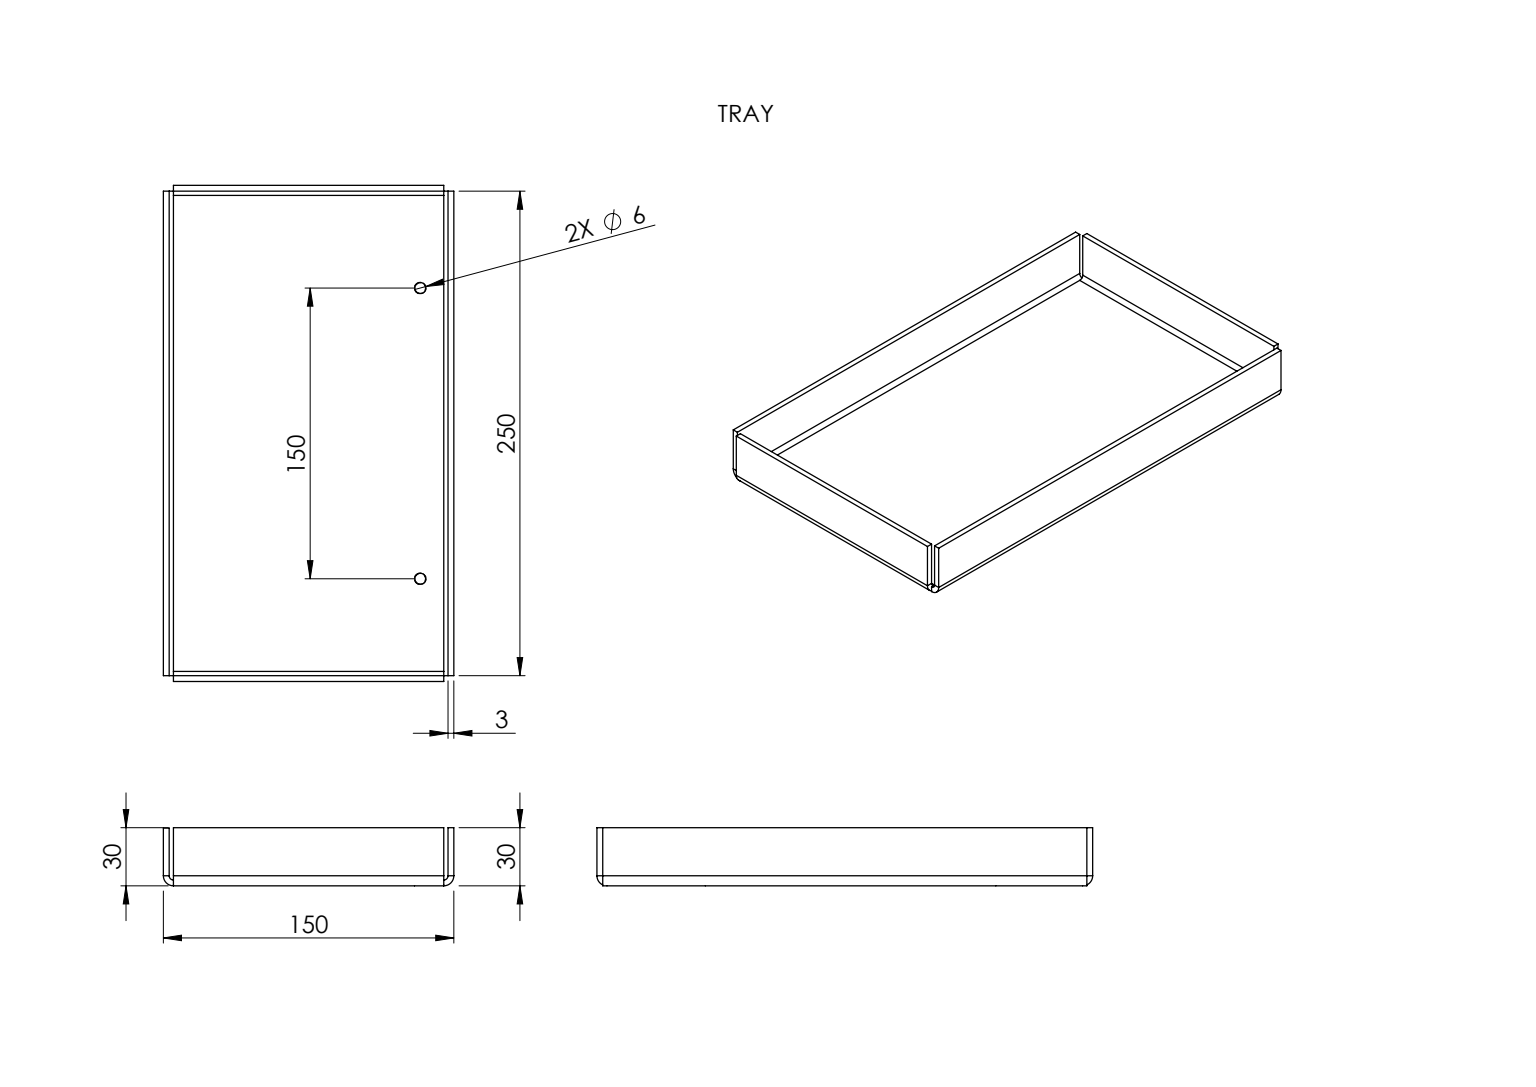
ISO-10303-21;
HEADER;
FILE_DESCRIPTION (('STEP AP214'),
    '1' );
FILE_NAME ('tray.step',
    '2026-10-25T17:17:34',
    ( '' ),
    ( '' ),
    'SwSTEP 2.0',
    'SolidWorks 2026',
    '' );
FILE_SCHEMA (( 'AUTOMOTIVE_DESIGN' ));
ENDSEC;

DATA;
#6=CARTESIAN_POINT ( 'NONE',  ( 231.0999999999999375, -32.62499999999999289, 102.5980762113533018 ) ) ;
#10=CARTESIAN_POINT ( 'NONE',  ( 232.5999999999999375, -34.55624999877095860, 96.53589838486223584 ) ) ;
#11=CARTESIAN_POINT ( 'NONE',  ( 234.0999999999999375, -32.34374999877096002, -52.59807621135342970 ) ) ;
#18=ORIENTED_EDGE ( 'NONE', *, *, #10099, .F. ) ;
#24=CARTESIAN_POINT ( 'NONE',  ( 231.7961524227065979, -33.50759618943233420, 103.0000000000000000 ) ) ;
#28=CARTESIAN_POINT ( 'NONE',  ( 233.9782151781249411, -31.19062499938547717, 97.61286128772489690 ) ) ;
#32=CARTESIAN_POINT ( 'NONE',  ( 233.4038475772933339, -34.57634618820330275, -53.00000000000011369 ) ) ;
#36=CARTESIAN_POINT ( 'NONE',  ( 233.9782151781249411, -32.54062499938547859, -52.38713871227520968 ) ) ;
#44=CARTESIAN_POINT ( 'NONE',  ( 235.3564303562499447, -33.92812499938548143, 98.40857419181659793 ) ) ;
#45=CARTESIAN_POINT ( 'NONE',  ( 232.5999999999999943, -33.40312499938547575, -53.18285161636690361 ) ) ;
#47=EDGE_CURVE ( 'NONE', #12317, #11119, #12856, .T. ) ;
#49=ORIENTED_EDGE ( 'NONE', *, *, #18550, .F. ) ;
#51=CARTESIAN_POINT ( 'NONE',  ( 235.3564303562499447, -34.41562499938547859, -50.00000000000011369 ) ) ;
#52=CARTESIAN_POINT ( 'NONE',  ( 232.5999999999999375, -33.20624999877097139, 97.00000000000000000 ) ) ;
#56=CARTESIAN_POINT ( 'NONE',  ( 233.9782151781249411, -31.90312499938548285, -47.61286128772501769 ) ) ;
#71=B_SPLINE_CURVE_WITH_KNOTS ( 'NONE', 3,
 ( #6677, #3729, #9694, #17123, #815, #2842, #14458, #7240, #5600, #9889, #2460, #18880, #18782, #15852, #1291, #17315, #16038, #17507 ),
 .UNSPECIFIED., .F., .F.,
 ( 4, 2, 2, 2, 2, 2, 2, 2, 4 ),
 ( 0.000000000000000000, 0.0007106627595359568412, 0.001421325519071913682, 0.002131988278607870740, 0.002842651038143827365, 0.003553313797679783989, 0.004263976557215741481, 0.004974639316751698105, 0.005685302076287654729 ),
 .UNSPECIFIED. ) ;
#78=PLANE ( 'NONE',  #7094 ) ;
#88=CARTESIAN_POINT ( 'NONE',  ( 105.2000000000000455, -29.80000000000002203, 147.7999999999999829 ) ) ;
#92=CARTESIAN_POINT ( 'NONE',  ( 229.8435696437499303, -31.60312499938548214, 99.99999999999998579 ) ) ;
#96=CARTESIAN_POINT ( 'NONE',  ( 233.4038475772933339, -33.67634618820329706, 96.99999999999998579 ) ) ;
#100=CARTESIAN_POINT ( 'NONE',  ( 232.5999999999999375, -33.43124999877096570, 102.9999999999999858 ) ) ;
#101=EDGE_CURVE ( 'NONE', #1894, #1510, #1410, .T. ) ;
#103=CARTESIAN_POINT ( 'NONE',  ( 232.5999999999999375, -34.61249999999999716, 96.53589838486223584 ) ) ;
#105=CARTESIAN_POINT ( 'NONE',  ( 231.2217848218749339, -34.22812499938548569, -47.61286128772501769 ) ) ;
#107=CARTESIAN_POINT ( 'NONE',  ( 233.9782151781249411, -30.55312499938548143, 102.3871387122750889 ) ) ;
#108=CARTESIAN_POINT ( 'NONE',  ( 229.5999999999999375, -33.99374999877096570, -50.00000000000011369 ) ) ;
#111=EDGE_CURVE ( 'NONE', #18607, #16633, #16646, .T. ) ;
#117=ORIENTED_EDGE ( 'NONE', *, *, #1142, .T. ) ;
#119=CARTESIAN_POINT ( 'NONE',  ( 232.5999999999999375, -32.36249999999999716, 97.00000000000000000 ) ) ;
#123=FACE_OUTER_BOUND ( 'NONE', #5516, .T. ) ;
#125=CARTESIAN_POINT ( 'NONE',  ( 234.0999999999999375, -33.29999999999999716, 97.40192378864668399 ) ) ;
#128=CARTESIAN_POINT ( 'NONE',  ( 229.8435696437499303, -31.04062499938547859, 99.99999999999998579 ) ) ;
#130=SHAPE_REPRESENTATION_RELATIONSHIP ( 'NONE' , 'NONE' ,  #4499, #5537 ) ;
#133=CARTESIAN_POINT ( 'NONE',  ( 233.4038475772933054, -34.76115380933863008, -47.00000000000011369 ) ) ;
#136=FACE_OUTER_BOUND ( 'NONE', #875, .T. ) ;
#137=CARTESIAN_POINT ( 'NONE',  ( 233.9782151781249411, -32.24062499938548143, -47.61286128772501769 ) ) ;
#138=VERTEX_POINT ( 'NONE', #3624 ) ;
#144=CARTESIAN_POINT ( 'NONE',  ( 244.7999999999999545, -32.00000000000000000, -100.0000000000000000 ) ) ;
#145=CARTESIAN_POINT ( 'NONE',  ( 231.2217848218749339, -34.71562499938547575, 97.61286128772489690 ) ) ;
#150=CARTESIAN_POINT ( 'NONE',  ( 235.5999999999999375, -32.47499999999999432, -50.00000000000011369 ) ) ;
#155=CARTESIAN_POINT ( 'NONE',  ( 229.8435696437499871, -31.11562499938547788, -48.40857419181671162 ) ) ;
#159=CARTESIAN_POINT ( 'NONE',  ( 233.9782151781249411, -34.94062499938547717, 102.3871387122750889 ) ) ;
#162=EDGE_CURVE ( 'NONE', #9344, #9023, #15270, .T. ) ;
#165=CARTESIAN_POINT ( 'NONE',  ( 230.0248882325332147, -35.00000000000000711, 98.48300226792288470 ) ) ;
#175=EDGE_CURVE ( 'NONE', #12231, #5767, #14452, .T. ) ;
#186=CARTESIAN_POINT ( 'NONE',  ( 232.5999999999999375, -34.61249999999999716, -53.00000000000011369 ) ) ;
#188=CARTESIAN_POINT ( 'NONE',  ( 233.9782151781249411, -32.35312499938547859, 102.3871387122750889 ) ) ;
#197=CARTESIAN_POINT ( 'NONE',  ( 235.5999999999999943, -34.76249999999999574, 101.7320508075688537 ) ) ;
#199=CARTESIAN_POINT ( 'NONE',  ( 231.2217848218749339, -34.37812499938547717, -52.38713871227520968 ) ) ;
#201=CARTESIAN_POINT ( 'NONE',  ( 229.8435696437499871, -30.66562499938547859, 101.5914258081833879 ) ) ;
#202=CARTESIAN_POINT ( 'NONE',  ( 229.5999999999999375, -33.95624999877095718, -48.26794919243123161 ) ) ;
#205=ORIENTED_EDGE ( 'NONE', *, *, #14467, .T. ) ;
#207=CARTESIAN_POINT ( 'NONE',  ( 105.1999999999999886, -29.80000000000002203, -100.0000000000000142 ) ) ;
#214=CARTESIAN_POINT ( 'NONE',  ( 229.5999999999999375, -33.60000000000000142, 99.99999999999998579 ) ) ;
#221=CARTESIAN_POINT ( 'NONE',  ( 235.3564303562499447, -32.16562499938547859, 99.99999999999998579 ) ) ;
#226=CARTESIAN_POINT ( 'NONE',  ( 235.5999999999999375, -33.82499999999999574, 99.99999999999998579 ) ) ;
#227=LINE ( 'NONE', #4417, #3668 ) ;
#228=CARTESIAN_POINT ( 'NONE',  ( 230.7429016803109221, -35.00000000000000711, -47.88253972981398476 ) ) ;
#229=LINE ( 'NONE', #334, #1662 ) ;
#238=CARTESIAN_POINT ( 'NONE',  ( 229.8435696437499303, -33.29062499938547148, 99.99999999999998579 ) ) ;
#239=CARTESIAN_POINT ( 'NONE',  ( 231.7960411235079050, -35.00000000000002132, -47.36341917746382535 ) ) ;
#240=VECTOR ( 'NONE', #19274, 1000.000000000000000 ) ;
#243=ORIENTED_EDGE ( 'NONE', *, *, #11982, .F. ) ;
#244=CARTESIAN_POINT ( 'NONE',  ( 229.5999999999999375, -32.21249999999999858, -48.26794919243123161 ) ) ;
#251=CARTESIAN_POINT ( 'NONE',  ( 233.9782151781249411, -33.70312499938548001, -47.61286128772501769 ) ) ;
#253=ORIENTED_EDGE ( 'NONE', *, *, #17135, .F. ) ;
#256=AXIS2_PLACEMENT_3D ( 'NONE', #7391, #10235, #1349 ) ;
#257=DIRECTION ( 'NONE',  ( 0.000000000000000000, 0.000000000000000000, -1.000000000000000000 ) ) ;
#267=CARTESIAN_POINT ( 'NONE',  ( 235.5999999999999943, -32.96249999999999858, -48.26794919243124582 ) ) ;
#274=AXIS2_PLACEMENT_3D ( 'NONE', #18067, #19141, #10151 ) ;
#285=CARTESIAN_POINT ( 'NONE',  ( 232.5999999999999375, -33.74062499938548143, 103.1828516163667899 ) ) ;
#297=CARTESIAN_POINT ( 'NONE',  ( 234.0999999999999375, -34.35000000000000142, 102.5980762113533018 ) ) ;
#299=CARTESIAN_POINT ( 'NONE',  ( 235.3564303562499447, -34.04062499938548569, -51.59142580818350154 ) ) ;
#301=CARTESIAN_POINT ( 'NONE',  ( 232.5999999999999375, -31.04062499938547859, 103.1828516163667899 ) ) ;
#302=CARTESIAN_POINT ( 'NONE',  ( 234.0999999999999375, -35.04374999877096286, -52.59807621135342970 ) ) ;
#303=ADVANCED_FACE ( 'NONE', ( #13187 ), #10269, .F. ) ;
#306=ORIENTED_EDGE ( 'NONE', *, *, #13225, .F. ) ;
#309=DIRECTION ( 'NONE',  ( -0.000000000000000000, -1.000000000000000000, -0.000000000000000000 ) ) ;
#310=ORIENTED_EDGE ( 'NONE', *, *, #16679, .T. ) ;
#312=CARTESIAN_POINT ( 'NONE',  ( 229.5999999999999375, -34.03124999877096002, 98.26794919243111792 ) ) ;
#317=CARTESIAN_POINT ( 'NONE',  ( 235.2013144571816952, -32.00000000000002132, -51.47161334219405404 ) ) ;
#318=ADVANCED_FACE ( 'NONE', ( #11630 ), #5967, .F. ) ;
#325=CARTESIAN_POINT ( 'NONE',  ( 229.8435696437499871, -32.42812499938548143, 98.40857419181659793 ) ) ;
#331=DIRECTION ( 'NONE',  ( 1.000000000000000000, 0.000000000000000000, 0.000000000000000000 ) ) ;
#333=CARTESIAN_POINT ( 'NONE',  ( 231.5655627039840567, -35.00000000000000000, -47.42249611015796518 ) ) ;
#334=CARTESIAN_POINT ( 'NONE',  ( 102.9999999999999858, -29.80000000000000071, -100.0000000000000000 ) ) ;
#343=CARTESIAN_POINT ( 'NONE',  ( 229.8435696437499871, -33.77812499938548285, 98.40857419181659793 ) ) ;
#347=ORIENTED_EDGE ( 'NONE', *, *, #19285, .F. ) ;
#348=CARTESIAN_POINT ( 'NONE',  ( 235.5999999999999943, -33.78749999999999432, -51.73205080756900287 ) ) ;
#354=CARTESIAN_POINT ( 'NONE',  ( 235.3564303562499447, -33.14062499938548001, -51.59142580818350865 ) ) ;
#356=ORIENTED_EDGE ( 'NONE', *, *, #12713, .T. ) ;
#358=CARTESIAN_POINT ( 'NONE',  ( 232.5999999999999943, -34.30312499938547433, 96.81714838363319586 ) ) ;
#360=CARTESIAN_POINT ( 'NONE',  ( 235.5999999999999943, -34.76249999999999574, 101.7320508075688537 ) ) ;
#362=CARTESIAN_POINT ( 'NONE',  ( 235.5999999999999375, -32.01330983656912821, 99.46005447970520663 ) ) ;
#365=CARTESIAN_POINT ( 'NONE',  ( 229.8435696437499303, -30.59062499938547575, -50.00000000000011369 ) ) ;
#370=CARTESIAN_POINT ( 'NONE',  ( 232.5999999999999091, -34.38749999999999574, 102.9999999999999858 ) ) ;
#379=CARTESIAN_POINT ( 'NONE',  ( 235.3564303562499447, -34.97812499938547859, 99.99999999999998579 ) ) ;
#381=EDGE_LOOP ( 'NONE', ( #16724, #7367, #9403, #6838, #9257, #5214, #15859, #12633, #9758, #10396, #17402, #15523, #2220, #3836, #18473, #563, #7521 ) ) ;
#385=CARTESIAN_POINT ( 'NONE',  ( 232.5999999999999375, -29.99999999999999645, -47.00000000000010658 ) ) ;
#389=AXIS2_PLACEMENT_3D ( 'NONE', #88, #5845, #13359 ) ;
#390=VECTOR ( 'NONE', #16629, 1000.000000000000000 ) ;
#392=CARTESIAN_POINT ( 'NONE',  ( 235.3564303562499447, -32.27812499938548285, -50.00000000000011369 ) ) ;
#393=CARTESIAN_POINT ( 'NONE',  ( 233.9782151781249411, -31.30312499938547788, 97.61286128772489690 ) ) ;
#394=CARTESIAN_POINT ( 'NONE',  ( 229.8435696437499303, -30.25312499938548072, -50.00000000000011369 ) ) ;
#401=ORIENTED_EDGE ( 'NONE', *, *, #14601, .T. ) ;
#407=AXIS2_PLACEMENT_3D ( 'NONE', #8734, #12848, #1036 ) ;
#412=EDGE_CURVE ( 'NONE', #3766, #15452, #4691, .T. ) ;
#416=CARTESIAN_POINT ( 'NONE',  ( 232.5999999999999375, -34.97812499938547859, 103.1828516163667899 ) ) ;
#417=CARTESIAN_POINT ( 'NONE',  ( 235.3564303562499447, -31.75312499938547717, 101.5914258081833879 ) ) ;
#424=CYLINDRICAL_SURFACE ( 'NONE', #15195, 5.200000000000009948 ) ;
#426=CARTESIAN_POINT ( 'NONE',  ( 230.1446115142513804, -34.99999999999998579, -51.72243138600839529 ) ) ;
#432=CARTESIAN_POINT ( 'NONE',  ( 233.4038475772933339, -33.28259618943232567, -53.00000000000011369 ) ) ;
#442=CARTESIAN_POINT ( 'NONE',  ( 231.0999999999999375, -33.07499999999999574, -47.40192378864679768 ) ) ;
#445=CARTESIAN_POINT ( 'NONE',  ( 230.2961164517930968, -35.00002705695767702, -51.92148140967023551 ) ) ;
#447=CARTESIAN_POINT ( 'NONE',  ( 232.5999999999999375, -33.29062499938547859, -46.81714838363331666 ) ) ;
#458=EDGE_CURVE ( 'NONE', #16633, #11798, #16899, .T. ) ;
#459=CARTESIAN_POINT ( 'NONE',  ( 229.8435696437499871, -31.90312499938547575, -48.40857419181671162 ) ) ;
#462=ORIENTED_EDGE ( 'NONE', *, *, #14610, .T. ) ;
#464=FACE_OUTER_BOUND ( 'NONE', #16767, .T. ) ;
#471=CARTESIAN_POINT ( 'NONE',  ( 231.7960411235079050, -35.00000000000002132, -47.36341917746382535 ) ) ;
#473=CARTESIAN_POINT ( 'NONE',  ( 231.7961524227065695, -33.00134618820329990, -47.00000000000011369 ) ) ;
#474=CARTESIAN_POINT ( 'NONE',  ( 230.4884518427504076, -35.25364861271050643, 98.22820072003833047 ) ) ;
#476=ORIENTED_EDGE ( 'NONE', *, *, #19168, .T. ) ;
#484=VERTEX_POINT ( 'NONE', #207 ) ;
#485=CARTESIAN_POINT ( 'NONE',  ( 235.3564303562499447, -32.76562499938548001, -48.40857419181671162 ) ) ;
#486=CARTESIAN_POINT ( 'NONE',  ( 231.2217848218749339, -32.42812499938548143, 102.3871387122750889 ) ) ;
#487=CARTESIAN_POINT ( 'NONE',  ( 229.8435696437499871, -31.56562499938547717, -48.40857419181671162 ) ) ;
#491=ORIENTED_EDGE ( 'NONE', *, *, #16294, .F. ) ;
#495=CARTESIAN_POINT ( 'NONE',  ( 105.1999999999999886, -29.80000000000001492, -97.80000000000002558 ) ) ;
#503=CARTESIAN_POINT ( 'NONE',  ( 233.4038475772933623, -32.32634618820329564, 97.00000000000000000 ) ) ;
#505=CARTESIAN_POINT ( 'NONE',  ( 235.3140393761304665, -32.00000000000000000, 101.2782762865722361 ) ) ;
#506=CARTESIAN_POINT ( 'NONE',  ( 235.3564303562499447, -34.45312499938548001, 101.5914258081833879 ) ) ;
#508=CARTESIAN_POINT ( 'NONE',  ( 235.5999999999999943, -30.58124999877096073, 98.26794919243110371 ) ) ;
#509=ORIENTED_EDGE ( 'NONE', *, *, #9352, .F. ) ;
#512=FACE_OUTER_BOUND ( 'NONE', #17537, .T. ) ;
#513=CARTESIAN_POINT ( 'NONE',  ( 229.7512376763150996, -35.00000000000002842, -49.45334139305044374 ) ) ;
#515=DIRECTION ( 'NONE',  ( 0.000000000000000000, 0.000000000000000000, 1.000000000000000000 ) ) ;
#524=CARTESIAN_POINT ( 'NONE',  ( 231.7961524227065979, -33.24240381056766580, 97.00000000000000000 ) ) ;
#525=AXIS2_PLACEMENT_3D ( 'NONE', #5549, #9836, #16188 ) ;
#529=ADVANCED_FACE ( 'NONE', ( #15427 ), #2038, .T. ) ;
#531=VERTEX_POINT ( 'NONE', #18462 ) ;
#532=CARTESIAN_POINT ( 'NONE',  ( 234.0999999999999375, -32.99999999999999289, -47.40192378864679768 ) ) ;
#535=CARTESIAN_POINT ( 'NONE',  ( 233.9782151781249411, -32.20312499938548001, 97.61286128772489690 ) ) ;
#537=CARTESIAN_POINT ( 'NONE',  ( 233.9782151781249411, -33.55312499938548143, -52.38713871227520968 ) ) ;
#539=EDGE_CURVE ( 'NONE', #8610, #7775, #12491, .T. ) ;
#542=CARTESIAN_POINT ( 'NONE',  ( 235.5999999999999943, -33.86249999999999716, -48.26794919243124582 ) ) ;
#545=CARTESIAN_POINT ( 'NONE',  ( 229.8848725447336960, -31.99999999999998579, -49.40473233008078324 ) ) ;
#552=CARTESIAN_POINT ( 'NONE',  ( 229.8435696437499303, -31.04062499938547859, -50.00000000000011369 ) ) ;
#558=AXIS2_PLACEMENT_3D ( 'NONE', #13780, #18191, #10944 ) ;
#562=CARTESIAN_POINT ( 'NONE',  ( 233.4038475772933623, -32.11740381056766580, -47.00000000000011369 ) ) ;
#563=ORIENTED_EDGE ( 'NONE', *, *, #2545, .T. ) ;
#565=AXIS2_PLACEMENT_3D ( 'NONE', #10279, #11928, #5692 ) ;
#570=CARTESIAN_POINT ( 'NONE',  ( 232.5999999999999375, -33.29062499938547859, 103.1828516163667899 ) ) ;
#578=DIRECTION ( 'NONE',  ( -0.000000000000000000, -1.000000000000000000, -0.000000000000000000 ) ) ;
#586=CARTESIAN_POINT ( 'NONE',  ( 231.2217848218749339, -33.32812499938548001, 102.3871387122750889 ) ) ;
#587=ADVANCED_FACE ( 'NONE', ( #14472 ), #5613, .F. ) ;
#588=CARTESIAN_POINT ( 'NONE',  ( 231.2217848218749339, -31.67812499938547788, -52.38713871227520968 ) ) ;
#605=DIRECTION ( 'NONE',  ( 0.000000000000000000, 0.000000000000000000, 1.000000000000000000 ) ) ;
#608=CARTESIAN_POINT ( 'NONE',  ( 229.8435696437499303, -33.74062499938548143, 99.99999999999998579 ) ) ;
#618=CARTESIAN_POINT ( 'NONE',  ( 233.9782151781249411, -34.34062499938547575, -52.38713871227520968 ) ) ;
#623=FACE_OUTER_BOUND ( 'NONE', #2442, .T. ) ;
#627=CARTESIAN_POINT ( 'NONE',  ( 229.5999999999999375, -33.14999999999999147, 99.99999999999998579 ) ) ;
#629=CARTESIAN_POINT ( 'NONE',  ( 235.2218879900010506, -35.00000000000000000, -49.14934632385183022 ) ) ;
#633=CARTESIAN_POINT ( 'NONE',  ( 231.0999999999999375, -33.97500000000000142, -47.40192378864679768 ) ) ;
#637=CARTESIAN_POINT ( 'NONE',  ( 232.5999999999999943, -32.84062499938548285, 103.1828516163667899 ) ) ;
#639=CARTESIAN_POINT ( 'NONE',  ( 235.3564303562499447, -33.59062499938548285, -51.59142580818350865 ) ) ;
#643=CARTESIAN_POINT ( 'NONE',  ( 232.5999999999999375, -33.93749999999999289, -47.00000000000011369 ) ) ;
#645=EDGE_CURVE ( 'NONE', #12702, #6637, #2949, .T. ) ;
#646=CARTESIAN_POINT ( 'NONE',  ( 230.5871892821561175, -32.00000000000001421, -51.89178425775511272 ) ) ;
#652=CARTESIAN_POINT ( 'NONE',  ( 235.3564303562499447, -31.26562499938547646, -50.00000000000011369 ) ) ;
#657=CARTESIAN_POINT ( 'NONE',  ( 233.4038475772933054, -34.36740381056765870, 102.9999999999999858 ) ) ;
#660=CARTESIAN_POINT ( 'NONE',  ( 235.5999999999999659, -32.01330983656912110, -50.53994552029475074 ) ) ;
#668=CARTESIAN_POINT ( 'NONE',  ( 229.8435696437499303, -33.40312499938547575, 99.99999999999998579 ) ) ;
#676=FACE_OUTER_BOUND ( 'NONE', #12537, .T. ) ;
#681=CARTESIAN_POINT ( 'NONE',  ( 235.3564303562499447, -33.17812499938548143, 99.99999999999998579 ) ) ;
#682=CARTESIAN_POINT ( 'NONE',  ( 232.5999999999999375, -32.39062499938548001, -46.81714838363331666 ) ) ;
#698=CARTESIAN_POINT ( 'NONE',  ( 229.5999999999999375, -34.03124999877096002, -51.73205080756898866 ) ) ;
#700=CARTESIAN_POINT ( 'NONE',  ( 235.3564303562499447, -33.02812499938547575, 98.40857419181659793 ) ) ;
#705=CARTESIAN_POINT ( 'NONE',  ( 229.5999999999999375, -31.25624999877096144, 101.7320508075688679 ) ) ;
#707=ORIENTED_EDGE ( 'NONE', *, *, #14527, .F. ) ;
#713=VECTOR ( 'NONE', #18943, 1000.000000000000000 ) ;
#727=AXIS2_PLACEMENT_3D ( 'NONE', #19099, #14307, #4057 ) ;
#730=CARTESIAN_POINT ( 'NONE',  ( 229.5999999999999375, -34.01249999999999574, -48.26794919243123161 ) ) ;
#732=DIRECTION ( 'NONE',  ( 0.000000000000000000, 0.000000000000000000, -1.000000000000000000 ) ) ;
#734=CARTESIAN_POINT ( 'NONE',  ( 235.3564303562499447, -31.22812499938548214, -51.59142580818350865 ) ) ;
#743=( BOUNDED_CURVE ( )  B_SPLINE_CURVE ( 2, ( #10018, #7083, #18723, #14593, #5344, #12754, #5443, #17347, #18913 ),
 .UNSPECIFIED., .F., .F. ) 
 B_SPLINE_CURVE_WITH_KNOTS ( ( 3, 2, 2, 2, 3 ),
 ( 0.6874999999999997780, 0.6944444444444444198, 0.7083333333333333703, 0.7222222222222222099, 0.7291666666666665186 ),
 .UNSPECIFIED. ) 
 CURVE ( )  GEOMETRIC_REPRESENTATION_ITEM ( )  RATIONAL_B_SPLINE_CURVE ( ( 0.9330127018922194093, 0.9330127018922171889, 1.000000000000000000, 0.8660254037844387076, 1.000000000000000000, 0.8660254037844387076, 1.000000000000000000, 0.9330127018922209636, 0.9330127018922194093 ) ) 
 REPRESENTATION_ITEM ( '' )  );
#745=CARTESIAN_POINT ( 'NONE',  ( 235.3564303562499447, -32.57812499938547290, -51.59142580818350865 ) ) ;
#754=EDGE_LOOP ( 'NONE', ( #205, #16125, #13208, #6303 ) ) ;
#756=EDGE_CURVE ( 'NONE', #10068, #15900, #4525, .T. ) ;
#757=EDGE_CURVE ( 'NONE', #1894, #5820, #10757, .T. ) ;
#759=CARTESIAN_POINT ( 'NONE',  ( 230.8788704469753839, -35.00000000000000000, -52.46580019096116132 ) ) ;
#761=CARTESIAN_POINT ( 'NONE',  ( 232.5999999999999375, -30.70312499938548001, 96.81714838363319586 ) ) ;
#764=CARTESIAN_POINT ( 'NONE',  ( 232.5999999999999659, -32.81249999999999289, 97.00000000000000000 ) ) ;
#774=CARTESIAN_POINT ( 'NONE',  ( 235.3564303562499447, -32.27812499938548285, 99.99999999999998579 ) ) ;
#775=CARTESIAN_POINT ( 'NONE',  ( 232.5999999999999375, -32.16562499938547859, -53.18285161636690361 ) ) ;
#783=EDGE_LOOP ( 'NONE', ( #3113, #7017, #8709, #2513 ) ) ;
#791=PRODUCT ( 'tray', 'tray', '', ( #18646 ) ) ;
#793=CARTESIAN_POINT ( 'NONE',  ( 234.1936318287815197, -32.00000000000000711, 102.4696265554870678 ) ) ;
#794=CARTESIAN_POINT ( 'NONE',  ( 232.5999999999999375, -32.95312499938548001, 96.81714838363319586 ) ) ;
#795=EDGE_LOOP ( 'NONE', ( #1159, #6294, #4402, #9977 ) ) ;
#797=CARTESIAN_POINT ( 'NONE',  ( 234.0999999999999375, -30.54374999877096286, 97.40192378864668399 ) ) ;
#798=CARTESIAN_POINT ( 'NONE',  ( 235.5999999999999943, -31.10624999877096286, -48.26794919243124582 ) ) ;
#801=CARTESIAN_POINT ( 'NONE',  ( 231.7961524227065695, -34.59240381056765301, 96.99999999999997158 ) ) ;
#804=VERTEX_POINT ( 'NONE', #7538 ) ;
#814=ADVANCED_FACE ( 'NONE', ( #136 ), #4908, .F. ) ;
#815=CARTESIAN_POINT ( 'NONE',  ( 233.5140320577117166, -35.00000000000000711, -52.81360193307793338 ) ) ;
#816=CYLINDRICAL_SURFACE ( 'NONE', #7870, 3.000000000000009770 ) ;
#818=DIRECTION ( 'NONE',  ( 0.000000000000000000, 0.000000000000000000, 1.000000000000000000 ) ) ;
#823=CARTESIAN_POINT ( 'NONE',  ( 235.5999999999999943, -34.23749999999999716, -51.73205080756900287 ) ) ;
#824=CARTESIAN_POINT ( 'NONE',  ( 233.4038475772932770, -33.22634618820329422, -53.00000000000011369 ) ) ;
#829=CARTESIAN_POINT ( 'NONE',  ( 231.2217848218749339, -30.21562499938547575, -52.38713871227520968 ) ) ;
#830=ORIENTED_EDGE ( 'NONE', *, *, #9352, .T. ) ;
#832=CARTESIAN_POINT ( 'NONE',  ( 249.9999999999999716, -29.80000000000000426, 150.0000000000000000 ) ) ;
#834=CARTESIAN_POINT ( 'NONE',  ( 234.0999999999999375, -33.89999999999999147, -47.40192378864679768 ) ) ;
#841=CARTESIAN_POINT ( 'NONE',  ( 235.3564303562499447, -33.06562499938547717, -50.00000000000011369 ) ) ;
#849=PLANE ( 'NONE',  #7119 ) ;
#850=ORIENTED_EDGE ( 'NONE', *, *, #11503, .F. ) ;
#862=CARTESIAN_POINT ( 'NONE',  ( 232.1470656674051440, -31.99999999999999289, 97.19890519204298585 ) ) ;
#869=CARTESIAN_POINT ( 'NONE',  ( 234.8201511961207757, -35.00000000000002132, -48.35655086105373357 ) ) ;
#870=CARTESIAN_POINT ( 'NONE',  ( 229.8435696437499871, -32.91562499938547859, -48.40857419181671162 ) ) ;
#875=EDGE_LOOP ( 'NONE', ( #11455, #8700, #7987, #17282 ) ) ;
#878=ORIENTED_EDGE ( 'NONE', *, *, #756, .T. ) ;
#890=LINE ( 'NONE', #18471, #3199 ) ;
#891=CARTESIAN_POINT ( 'NONE',  ( 231.0999999999999375, -30.37499999999999645, 102.5980762113533018 ) ) ;
#896=CARTESIAN_POINT ( 'NONE',  ( 234.0999999999999375, -32.04374999877096286, -47.40192378864679768 ) ) ;
#898=CARTESIAN_POINT ( 'NONE',  ( 229.5999999999999375, -32.64374999877096428, 99.99999999999998579 ) ) ;
#901=ORIENTED_EDGE ( 'NONE', *, *, #18919, .F. ) ;
#902=CARTESIAN_POINT ( 'NONE',  ( 232.5999999999999091, -33.03749999999998721, -47.00000000000011369 ) ) ;
#904=ORIENTED_EDGE ( 'NONE', *, *, #13663, .T. ) ;
#912=CARTESIAN_POINT ( 'NONE',  ( 233.0909187468006678, -31.99999999999998579, -52.83814945501250548 ) ) ;
#920=CARTESIAN_POINT ( 'NONE',  ( 230.3018593135002448, -35.00052333152935802, -51.92835406112443053 ) ) ;
#923=CARTESIAN_POINT ( 'NONE',  ( 232.5999999999999943, -33.96562499938547575, 96.81714838363319586 ) ) ;
#926=CARTESIAN_POINT ( 'NONE',  ( 229.8435696437499871, -30.62812499938547717, -51.59142580818350865 ) ) ;
#927=VERTEX_POINT ( 'NONE', #3719 ) ;
#932=LINE ( 'NONE', #5430, #6200 ) ;
#933=CARTESIAN_POINT ( 'NONE',  ( 232.5999999999999943, -32.50312499938547717, -53.18285161636690361 ) ) ;
#939=CARTESIAN_POINT ( 'NONE',  ( 233.9782151781249411, -34.04062499938547859, -47.61286128772501769 ) ) ;
#944=CARTESIAN_POINT ( 'NONE',  ( 231.0999999999999375, -32.32499999999999574, 97.40192378864668399 ) ) ;
#951=ORIENTED_EDGE ( 'NONE', *, *, #14019, .F. ) ;
#968=CARTESIAN_POINT ( 'NONE',  ( 229.8435696437499871, -34.34062499938547575, 98.40857419181659793 ) ) ;
#969=CARTESIAN_POINT ( 'NONE',  ( 233.9782151781249411, -33.70312499938548001, -47.61286128772501769 ) ) ;
#975=EDGE_LOOP ( 'NONE', ( #10803, #15981, #15454, #9666, #3524 ) ) ;
#979=CARTESIAN_POINT ( 'NONE',  ( 231.2217848218749339, -30.32812499938548001, 97.61286128772489690 ) ) ;
#983=CARTESIAN_POINT ( 'NONE',  ( 233.7151113960924818, -35.00000000000000711, 102.5271494742949017 ) ) ;
#985=CARTESIAN_POINT ( 'NONE',  ( 231.0999999999999375, -31.27499999999999858, 102.5980762113533018 ) ) ;
#988=CARTESIAN_POINT ( 'NONE',  ( 234.0999999999999375, -33.69374999877096144, 97.40192378864668399 ) ) ;
#989=CARTESIAN_POINT ( 'NONE',  ( 232.5999999999999375, -32.08124999877095718, -46.53589838486234953 ) ) ;
#994=ORIENTED_EDGE ( 'NONE', *, *, #2088, .F. ) ;
#996=CARTESIAN_POINT ( 'NONE',  ( 229.5999999999999375, -33.05624999877096570, 101.7320508075688821 ) ) ;
#1002=ADVANCED_FACE ( 'NONE', ( #18772 ), #8405, .F. ) ;
#1006=LINE ( 'NONE', #5601, #3813 ) ;
#1011=EDGE_LOOP ( 'NONE', ( #18338, #12679, #3902, #3454 ) ) ;
#1012=CARTESIAN_POINT ( 'NONE',  ( 235.5999999999999943, -34.76249999999999574, -48.26794919243124582 ) ) ;
#1014=AXIS2_PLACEMENT_3D ( 'NONE', #15088, #13614, #257 ) ;
#1016=EDGE_CURVE ( 'NONE', #17889, #804, #14357, .T. ) ;
#1018=CARTESIAN_POINT ( 'NONE',  ( 229.8435696437499587, -33.89062499938548001, 98.40857419181659793 ) ) ;
#1021=CARTESIAN_POINT ( 'NONE',  ( 229.8435696437499871, -31.07812499938548001, -51.59142580818350865 ) ) ;
#1022=VERTEX_POINT ( 'NONE', #9780 ) ;
#1026=CARTESIAN_POINT ( 'NONE',  ( 244.7999999999999545, -35.00000000000000000, -100.0000000000000000 ) ) ;
#1027=CARTESIAN_POINT ( 'NONE',  ( 231.2217848218749339, -32.31562499938547717, -47.61286128772501769 ) ) ;
#1032=CARTESIAN_POINT ( 'NONE',  ( 235.3564303562499447, -32.16562499938547859, -50.00000000000011369 ) ) ;
#1036=DIRECTION ( 'NONE',  ( 0.000000000000000000, -3.154042683594203897E-15, -1.000000000000000000 ) ) ;
#1042=CARTESIAN_POINT ( 'NONE',  ( 232.5999999999999375, -34.16249999999999432, 96.99999999999998579 ) ) ;
#1044=CARTESIAN_POINT ( 'NONE',  ( 233.9782151781249411, -32.69062499938547717, 102.3871387122750889 ) ) ;
#1051=CARTESIAN_POINT ( 'NONE',  ( 232.5999999999999375, -29.99999999999999645, -50.00000000000011369 ) ) ;
#1054=CARTESIAN_POINT ( 'NONE',  ( 229.5999999999999375, -34.08749999999999147, 98.26794919243111792 ) ) ;
#1057=CARTESIAN_POINT ( 'NONE',  ( 232.5999999999999375, -34.83749999999999147, 103.0000000000000000 ) ) ;
#1058=CARTESIAN_POINT ( 'NONE',  ( 232.5999999999999375, -32.84062499938548285, -46.81714838363331666 ) ) ;
#1061=ORIENTED_EDGE ( 'NONE', *, *, #15792, .T. ) ;
#1072=CARTESIAN_POINT ( 'NONE',  ( 235.1663847376153740, -35.00000000000000000, 101.0217260113606983 ) ) ;
#1074=CARTESIAN_POINT ( 'NONE',  ( 231.0999999999999375, -30.52499999999999503, 97.40192378864668399 ) ) ;
#1075=ORIENTED_EDGE ( 'NONE', *, *, #13319, .F. ) ;
#1077=CARTESIAN_POINT ( 'NONE',  ( 229.5999999999999375, -31.74374999877096215, 99.99999999999998579 ) ) ;
#1079=CARTESIAN_POINT ( 'NONE',  ( 231.0999999999999375, -34.42499999999999716, 102.5980762113533018 ) ) ;
#1082=ORIENTED_EDGE ( 'NONE', *, *, #1142, .F. ) ;
#1104=CARTESIAN_POINT ( 'NONE',  ( 235.3564303562499447, -34.97812499938547859, -50.00000000000011369 ) ) ;
#1110=CARTESIAN_POINT ( 'NONE',  ( 229.8435696437499871, -31.00312499938547361, 101.5914258081833879 ) ) ;
#1112=EDGE_CURVE ( 'NONE', #11694, #3907, #10561, .T. ) ;
#1118=CARTESIAN_POINT ( 'NONE',  ( 229.8435696437499303, -33.74062499938548143, -50.00000000000011369 ) ) ;
#1130=ORIENTED_EDGE ( 'NONE', *, *, #13051, .F. ) ;
#1132=CARTESIAN_POINT ( 'NONE',  ( 229.8435696437499303, -32.39062499938548001, 99.99999999999998579 ) ) ;
#1142=EDGE_CURVE ( 'NONE', #18598, #4852, #9158, .T. ) ;
#1150=CARTESIAN_POINT ( 'NONE',  ( 231.2217848218749339, -33.92812499938548143, 97.61286128772489690 ) ) ;
#1153=CARTESIAN_POINT ( 'NONE',  ( 235.5999999999999375, -34.21874999877096002, 99.99999999999998579 ) ) ;
#1159=ORIENTED_EDGE ( 'NONE', *, *, #47, .F. ) ;
#1167=DIRECTION ( 'NONE',  ( -0.000000000000000000, -1.000000000000000000, -0.000000000000000000 ) ) ;
#1172=CARTESIAN_POINT ( 'NONE',  ( 229.5999999999999375, -31.79999999999999361, 99.99999999999998579 ) ) ;
#1174=CARTESIAN_POINT ( 'NONE',  ( 233.4038475772933054, -34.76115380933863008, 102.9999999999999858 ) ) ;
#1176=CARTESIAN_POINT ( 'NONE',  ( 235.5999999999999943, -31.93124999877096570, 98.26794919243110371 ) ) ;
#1177=CARTESIAN_POINT ( 'NONE',  ( 231.0999999999999375, -31.36874999877096215, -52.59807621135342970 ) ) ;
#1178=CARTESIAN_POINT ( 'NONE',  ( 231.0999999999999375, -32.71874999877096002, 97.40192378864668399 ) ) ;
#1194=DIRECTION ( 'NONE',  ( 1.000000000000000000, 0.000000000000000000, 0.000000000000000000 ) ) ;
#1197=CARTESIAN_POINT ( 'NONE',  ( 233.9782151781249411, -30.89062499938548001, 102.3871387122750889 ) ) ;
#1198=ORIENTED_EDGE ( 'NONE', *, *, #12336, .T. ) ;
#1203=CARTESIAN_POINT ( 'NONE',  ( 229.8435696437499587, -34.26562499938548001, 101.5914258081833879 ) ) ;
#1205=DIRECTION ( 'NONE',  ( 0.000000000000000000, -1.000000000000000000, 0.000000000000000000 ) ) ;
#1206=CARTESIAN_POINT ( 'NONE',  ( 229.8435696437499871, -31.97812499938548214, -51.59142580818350865 ) ) ;
#1207=ORIENTED_EDGE ( 'NONE', *, *, #17821, .T. ) ;
#1213=CARTESIAN_POINT ( 'NONE',  ( 231.2217848218749339, -31.41562499938547859, 102.3871387122750889 ) ) ;
#1219=CARTESIAN_POINT ( 'NONE',  ( 229.8435696437499871, -34.60312499938547859, -48.40857419181671162 ) ) ;
#1230=EDGE_CURVE ( 'NONE', #15440, #927, #890, .T. ) ;
#1231=CARTESIAN_POINT ( 'NONE',  ( 229.8435696437499587, -32.35312499938547859, 101.5914258081833879 ) ) ;
#1235=EDGE_CURVE ( 'NONE', #18970, #10663, #1963, .T. ) ;
#1237=CARTESIAN_POINT ( 'NONE',  ( 234.7546687845693327, -31.99999999999999289, -47.95829548583744639 ) ) ;
#1242=CARTESIAN_POINT ( 'NONE',  ( 229.5999999999999375, -34.89374999877096428, 99.99999999999998579 ) ) ;
#1248=CARTESIAN_POINT ( 'NONE',  ( 234.1913891058630099, -35.00000000000002842, -47.72105564972103053 ) ) ;
#1249=CARTESIAN_POINT ( 'NONE',  ( 233.9782151781249411, -34.60312499938548569, -47.61286128772501769 ) ) ;
#1255=ADVANCED_FACE ( 'NONE', ( #8008 ), #5384, .F. ) ;
#1264=CARTESIAN_POINT ( 'NONE',  ( 235.3564303562499447, -32.31562499938547717, 101.5914258081833879 ) ) ;
#1269=CARTESIAN_POINT ( 'NONE',  ( 230.2961164517930968, -35.00002705695778360, 98.07851859032987818 ) ) ;
#1271=CARTESIAN_POINT ( 'NONE',  ( 235.5999999999999943, -31.61249999999999716, 101.7320508075688537 ) ) ;
#1275=CARTESIAN_POINT ( 'NONE',  ( 235.5999999999999943, -32.83124999877095718, 98.26794919243110371 ) ) ;
#1276=CARTESIAN_POINT ( 'NONE',  ( 229.5999999999999375, -33.54374999877096286, -50.00000000000011369 ) ) ;
#1278=ORIENTED_EDGE ( 'NONE', *, *, #15378, .T. ) ;
#1291=CARTESIAN_POINT ( 'NONE',  ( 235.4063471324518275, -34.99999999999999289, -50.07101444713918426 ) ) ;
#1296=CARTESIAN_POINT ( 'NONE',  ( 229.8435696437499303, -30.14062499938548001, 99.99999999999998579 ) ) ;
#1299=CARTESIAN_POINT ( 'NONE',  ( 232.5999999999999659, -32.58749999999999858, -47.00000000000011369 ) ) ;
#1304=DIRECTION ( 'NONE',  ( 0.000000000000000000, 0.000000000000000000, -1.000000000000000000 ) ) ;
#1305=CARTESIAN_POINT ( 'NONE',  ( 229.8435696437499871, -33.77812499938548285, -51.59142580818350865 ) ) ;
#1313=CARTESIAN_POINT ( 'NONE',  ( 231.2217848218749339, -31.11562499938547788, 97.61286128772489690 ) ) ;
#1314=CARTESIAN_POINT ( 'NONE',  ( 233.9782151781249411, -34.34062499938547575, -52.38713871227520968 ) ) ;
#1319=CARTESIAN_POINT ( 'NONE',  ( 235.5999999999999943, -30.63749999999999574, -51.73205080756900287 ) ) ;
#1326=ORIENTED_EDGE ( 'NONE', *, *, #11982, .T. ) ;
#1332=CARTESIAN_POINT ( 'NONE',  ( 230.7186334667983658, -32.00000000000000711, 97.98546077809203325 ) ) ;
#1338=CARTESIAN_POINT ( 'NONE',  ( 230.5871892821561460, -32.00000000000002132, 98.10821574224502228 ) ) ;
#1344=VECTOR ( 'NONE', #12767, 1000.000000000000000 ) ;
#1349=DIRECTION ( 'NONE',  ( 0.000000000000000000, 0.000000000000000000, -1.000000000000000000 ) ) ;
#1352=CARTESIAN_POINT ( 'NONE',  ( 232.5999999999999375, -29.99999999999999645, -50.00000000000011369 ) ) ;
#1358=LINE ( 'NONE', #16493, #4568 ) ;
#1360=CARTESIAN_POINT ( 'NONE',  ( 229.8435696437499871, -31.64062499938547290, 98.40857419181659793 ) ) ;
#1368=CARTESIAN_POINT ( 'NONE',  ( 229.5999999999999375, -34.49999999999999289, 99.99999999999998579 ) ) ;
#1370=VERTEX_POINT ( 'NONE', #1536 ) ;
#1372=CARTESIAN_POINT ( 'NONE',  ( 234.0999999999999375, -33.84374999877096002, 102.5980762113533018 ) ) ;
#1373=CARTESIAN_POINT ( 'NONE',  ( 231.0999999999999375, -33.61874999877096570, -52.59807621135342970 ) ) ;
#1376=ORIENTED_EDGE ( 'NONE', *, *, #12861, .T. ) ;
#1377=ORIENTED_EDGE ( 'NONE', *, *, #4747, .T. ) ;
#1379=CARTESIAN_POINT ( 'NONE',  ( 229.5999999999999091, -34.97364041986482164, 98.90809577818235709 ) ) ;
#1390=CARTESIAN_POINT ( 'NONE',  ( 105.1999999999999744, -31.99999999999999289, 150.0000000000000000 ) ) ;
#1394=LINE ( 'NONE', #3134, #18639 ) ;
#1397=CARTESIAN_POINT ( 'NONE',  ( 232.5999999999999375, -32.95312499938548001, -53.18285161636690361 ) ) ;
#1406=CARTESIAN_POINT ( 'NONE',  ( 229.8435696437499871, -31.45312499938547290, 101.5914258081833879 ) ) ;
#1407=CARTESIAN_POINT ( 'NONE',  ( 232.9413037568956497, -34.96883842999723413, -47.01420019955246943 ) ) ;
#1410=( BOUNDED_CURVE ( )  B_SPLINE_CURVE ( 2, ( #17115, #5399, #8408, #996, #12710, #18873, #5300, #11342, #17307 ),
 .UNSPECIFIED., .F., .F. ) 
 B_SPLINE_CURVE_WITH_KNOTS ( ( 3, 2, 2, 2, 3 ),
 ( 0.4791666666666666852, 0.4861111111111111049, 0.5000000000000000000, 0.5138888888888888395, 0.5208333333333331483 ),
 .UNSPECIFIED. ) 
 CURVE ( )  GEOMETRIC_REPRESENTATION_ITEM ( )  RATIONAL_B_SPLINE_CURVE ( ( 0.9330127018922194093, 0.9330127018922196314, 1.000000000000000000, 0.8660254037844387076, 1.000000000000000000, 0.8660254037844387076, 1.000000000000000000, 0.9330127018922209636, 0.9330127018922194093 ) ) 
 REPRESENTATION_ITEM ( '' )  );
#1411=CARTESIAN_POINT ( 'NONE',  ( 234.0999999999999375, -31.19999999999999574, -47.40192378864679768 ) ) ;
#1417=CARTESIAN_POINT ( 'NONE',  ( 233.9782151781249411, -31.30312499938547788, -52.38713871227520968 ) ) ;
#1426=DIRECTION ( 'NONE',  ( 0.000000000000000000, 0.000000000000000000, 1.000000000000000000 ) ) ;
#1436=CARTESIAN_POINT ( 'NONE',  ( 235.3564303562499447, -35.01562499938548001, -48.40857419181671162 ) ) ;
#1438=( BOUNDED_CURVE ( )  B_SPLINE_CURVE ( 2, ( #16800, #7900, #18171, #3212, #17981, #6256, #12109, #12397, #3501 ),
 .UNSPECIFIED., .F., .F. ) 
 B_SPLINE_CURVE_WITH_KNOTS ( ( 3, 2, 2, 2, 3 ),
 ( 0.3958333333333333703, 0.4027777777777777901, 0.4166666666666666852, 0.4305555555555555802, 0.4375000000000001110 ),
 .UNSPECIFIED. ) 
 CURVE ( )  GEOMETRIC_REPRESENTATION_ITEM ( )  RATIONAL_B_SPLINE_CURVE ( ( 0.9330127018922194093, 0.9330127018922196314, 1.000000000000000000, 0.8660254037844387076, 1.000000000000000000, 0.8660254037844387076, 1.000000000000000000, 0.9330127018922182991, 0.9330127018922194093 ) ) 
 REPRESENTATION_ITEM ( '' )  );
#1449=CARTESIAN_POINT ( 'NONE',  ( 229.8435696437499303, -30.70312499938548001, 99.99999999999998579 ) ) ;
#1457=CARTESIAN_POINT ( 'NONE',  ( 234.0999999999999375, -33.29999999999999716, 97.40192378864668399 ) ) ;
#1461=CARTESIAN_POINT ( 'NONE',  ( 233.9782151781249411, -31.00312499938548072, 102.3871387122750889 ) ) ;
#1462=CARTESIAN_POINT ( 'NONE',  ( 231.0999999999999375, -33.01874999877096428, -47.40192378864679768 ) ) ;
#1472=CYLINDRICAL_SURFACE ( 'NONE', #10483, 3.000000000000002665 ) ;
#1481=LINE ( 'NONE', #1390, #9928 ) ;
#1488=LINE ( 'NONE', #7441, #11783 ) ;
#1493=CARTESIAN_POINT ( 'NONE',  ( 235.3564303562499447, -33.55312499938548143, -48.40857419181671162 ) ) ;
#1498=VERTEX_POINT ( 'NONE', #7268 ) ;
#1500=EDGE_CURVE ( 'NONE', #484, #2622, #14883, .T. ) ;
#1503=VECTOR ( 'NONE', #6129, 1000.000000000000000 ) ;
#1505=CARTESIAN_POINT ( 'NONE',  ( 235.3564303562499447, -33.10312499938547859, 101.5914258081833879 ) ) ;
#1506=CARTESIAN_POINT ( 'NONE',  ( 235.3564303562499447, -33.92812499938548143, -51.59142580818350154 ) ) ;
#1510=VERTEX_POINT ( 'NONE', #52 ) ;
#1512=CARTESIAN_POINT ( 'NONE',  ( 235.5999999999999943, -30.71249999999999858, -48.26794919243124582 ) ) ;
#1515=ORIENTED_EDGE ( 'NONE', *, *, #11295, .T. ) ;
#1516=CARTESIAN_POINT ( 'NONE',  ( 232.5999999999999375, -34.33124999877097139, -47.00000000000011369 ) ) ;
#1519=CARTESIAN_POINT ( 'NONE',  ( 229.8435696437499871, -31.56562499938547717, -48.40857419181671162 ) ) ;
#1536=CARTESIAN_POINT ( 'NONE',  ( 232.5999999999999091, -34.10624999877096286, -53.00000000000010658 ) ) ;
#1539=ORIENTED_EDGE ( 'NONE', *, *, #14831, .T. ) ;
#1542=FACE_OUTER_BOUND ( 'NONE', #2026, .T. ) ;
#1553=CARTESIAN_POINT ( 'NONE',  ( 232.5999999999999375, -32.84062499938548285, 103.1828516163667899 ) ) ;
#1558=CARTESIAN_POINT ( 'NONE',  ( 244.7999999999999545, -29.80000000000000426, -100.0000000000000000 ) ) ;
#1561=CARTESIAN_POINT ( 'NONE',  ( 235.5999999999999943, -34.31249999999999289, 101.7320508075688537 ) ) ;
#1563=CARTESIAN_POINT ( 'NONE',  ( 235.3564303562499447, -34.11562499938548143, -48.40857419181671162 ) ) ;
#1565=CARTESIAN_POINT ( 'NONE',  ( 229.5999999999999375, -34.85624999877096286, 101.7320508075688679 ) ) ;
#1566=CARTESIAN_POINT ( 'NONE',  ( 235.5999999999999375, -33.31874999877096144, -50.00000000000011369 ) ) ;
#1585=CARTESIAN_POINT ( 'NONE',  ( 105.1999999999999744, -34.51168759575592304, 150.0000000000000000 ) ) ;
#1587=CARTESIAN_POINT ( 'NONE',  ( 235.5999999999999943, -33.86249999999999716, 101.7320508075688537 ) ) ;
#1588=DIRECTION ( 'NONE',  ( -4.625929269271485791E-17, -1.000000000000000000, 0.000000000000000000 ) ) ;
#1590=CARTESIAN_POINT ( 'NONE',  ( 230.2961164517930968, -35.00002705695767702, -51.92148140967023551 ) ) ;
#1591=CARTESIAN_POINT ( 'NONE',  ( 229.8435696437499303, -31.94062499938547717, -50.00000000000011369 ) ) ;
#1593=ADVANCED_FACE ( 'NONE', ( #19245 ), #7034, .T. ) ;
#1600=DIRECTION ( 'NONE',  ( 5.836151346627967635E-31, -2.699762333426451414E-47, -1.000000000000000000 ) ) ;
#1601=CARTESIAN_POINT ( 'NONE',  ( 232.5999999999999375, -32.72812499938547859, 103.1828516163667899 ) ) ;
#1602=CARTESIAN_POINT ( 'NONE',  ( 235.3564303562499447, -33.06562499938547717, -50.00000000000011369 ) ) ;
#1607=CARTESIAN_POINT ( 'NONE',  ( 232.5999999999999375, -31.23749999999999361, -46.53589838486234953 ) ) ;
#1613=CARTESIAN_POINT ( 'NONE',  ( 235.3564303562499447, -30.44062499938548072, -51.59142580818350865 ) ) ;
#1624=CARTESIAN_POINT ( 'NONE',  ( 229.5999999999999375, -33.11249999999999716, -48.26794919243123161 ) ) ;
#1632=AXIS2_PLACEMENT_3D ( 'NONE', #9289, #13587, #3137 ) ;
#1634=FACE_OUTER_BOUND ( 'NONE', #9231, .T. ) ;
#1639=EDGE_CURVE ( 'NONE', #531, #13951, #18644, .T. ) ;
#1641=CARTESIAN_POINT ( 'NONE',  ( 232.5999999999999375, -29.99999999999999645, -47.00000000000010658 ) ) ;
#1642=CARTESIAN_POINT ( 'NONE',  ( 231.2217848218749339, -31.52812499938548285, 102.3871387122750889 ) ) ;
#1647=DIRECTION ( 'NONE',  ( -0.000000000000000000, -1.000000000000000000, -0.000000000000000000 ) ) ;
#1648=VECTOR ( 'NONE', #8322, 1000.000000000000000 ) ;
#1649=VECTOR ( 'NONE', #3154, 1000.000000000000000 ) ;
#1652=CARTESIAN_POINT ( 'NONE',  ( 235.5999999999999943, -32.43749999999999289, 98.26794919243110371 ) ) ;
#1654=CARTESIAN_POINT ( 'NONE',  ( 233.9782151781249411, -33.25312499938547717, -47.61286128772501769 ) ) ;
#1656=CARTESIAN_POINT ( 'NONE',  ( 231.2217848218749339, -31.22812499938547859, 97.61286128772489690 ) ) ;
#1657=CARTESIAN_POINT ( 'NONE',  ( 232.5999999999999375, -32.98124999877096286, -46.53589838486234953 ) ) ;
#1662=VECTOR ( 'NONE', #515, 1000.000000000000000 ) ;
#1675=CARTESIAN_POINT ( 'NONE',  ( 232.5999999999999375, -32.05312499938548143, 96.81714838363319586 ) ) ;
#1680=DIRECTION ( 'NONE',  ( -1.000000000000000000, 0.000000000000000000, 0.000000000000000000 ) ) ;
#1681=PLANE ( 'NONE',  #8961 ) ;
#1683=CARTESIAN_POINT ( 'NONE',  ( 231.2217848218749339, -34.11562499938548143, -47.61286128772501769 ) ) ;
#1684=ORIENTED_EDGE ( 'NONE', *, *, #2088, .T. ) ;
#1691=CARTESIAN_POINT ( 'NONE',  ( 232.5999999999999375, -34.30312499938547433, 96.81714838363319586 ) ) ;
#1696=CARTESIAN_POINT ( 'NONE',  ( 235.5999999999999943, -32.88749999999998863, -51.73205080756900287 ) ) ;
#1701=CARTESIAN_POINT ( 'NONE',  ( 232.5999999999999375, -32.84062499938548285, -46.81714838363331666 ) ) ;
#1705=CARTESIAN_POINT ( 'NONE',  ( 229.8435696437499587, -34.22812499938547859, 98.40857419181659793 ) ) ;
#1710=CARTESIAN_POINT ( 'NONE',  ( 231.5655627039825504, -35.00000000000000000, 102.5775038898417080 ) ) ;
#1714=CARTESIAN_POINT ( 'NONE',  ( 232.5999999999999375, -31.60312499938548214, -53.18285161636690361 ) ) ;
#1723=EDGE_CURVE ( 'NONE', #16053, #18412, #14010, .T. ) ;
#1730=CARTESIAN_POINT ( 'NONE',  ( 235.3564303562499447, -34.52812499938547575, 99.99999999999998579 ) ) ;
#1740=CARTESIAN_POINT ( 'NONE',  ( 229.5999999999999375, -34.46249999999999147, 101.7320508075688679 ) ) ;
#1742=CARTESIAN_POINT ( 'NONE',  ( 232.5999999999999943, -32.84062499938548285, -46.81714838363331666 ) ) ;
#1745=CARTESIAN_POINT ( 'NONE',  ( 229.5999999999999375, -34.93124999877095860, 98.26794919243111792 ) ) ;
#1746=CARTESIAN_POINT ( 'NONE',  ( 229.5999999999999375, -35.34374999877096002, -50.00000000000011369 ) ) ;
#1763=CARTESIAN_POINT ( 'NONE',  ( 249.9999999999999716, -35.00000000000000000, -100.0000000000000000 ) ) ;
#1766=CARTESIAN_POINT ( 'NONE',  ( 232.5999999999999375, -32.27812499938547575, 103.1828516163667899 ) ) ;
#1769=DIRECTION ( 'NONE',  ( -0.000000000000000000, 1.000000000000000000, 0.000000000000000000 ) ) ;
#1771=CARTESIAN_POINT ( 'NONE',  ( 231.7961524227065695, -34.35134618820329422, 103.0000000000000000 ) ) ;
#1773=CARTESIAN_POINT ( 'NONE',  ( 233.9782151781249411, -34.49062499938548143, -47.61286128772501769 ) ) ;
#1774=CARTESIAN_POINT ( 'NONE',  ( 229.8435696437499303, -32.50312499938547717, 99.99999999999998579 ) ) ;
#1782=CARTESIAN_POINT ( 'NONE',  ( 233.9782151781249411, -34.49062499938548143, 102.3871387122750889 ) ) ;
#1788=CARTESIAN_POINT ( 'NONE',  ( 231.0999999999999375, -33.67499999999999716, -52.59807621135342970 ) ) ;
#1794=CARTESIAN_POINT ( 'NONE',  ( 232.5999999999999375, -32.39062499938548001, -46.81714838363331666 ) ) ;
#1800=AXIS2_PLACEMENT_3D ( 'NONE', #15147, #16426, #4607 ) ;
#1811=ORIENTED_EDGE ( 'NONE', *, *, #6489, .F. ) ;
#1814=VECTOR ( 'NONE', #818, 1000.000000000000000 ) ;
#1822=ADVANCED_FACE ( 'NONE', ( #7179 ), #13129, .F. ) ;
#1827=CARTESIAN_POINT ( 'NONE',  ( 229.8435696437499871, -34.79062499938547859, 98.40857419181659793 ) ) ;
#1830=CARTESIAN_POINT ( 'NONE',  ( 231.0999999999999375, -32.62499999999999289, 102.5980762113533018 ) ) ;
#1834=DIRECTION ( 'NONE',  ( 0.000000000000000000, 0.000000000000000000, -1.000000000000000000 ) ) ;
#1836=CYLINDRICAL_SURFACE ( 'NONE', #10218, 3.000000000000002665 ) ;
#1837=ADVANCED_FACE ( 'NONE', ( #9921 ), #16171, .F. ) ;
#1839=CARTESIAN_POINT ( 'NONE',  ( 231.2217848218749339, -32.42812499938548143, -47.61286128772501769 ) ) ;
#1841=CARTESIAN_POINT ( 'NONE',  ( 231.0999999999999375, -34.51874999877096428, 97.40192378864668399 ) ) ;
#1843=CARTESIAN_POINT ( 'NONE',  ( 231.0999999999999375, -35.26874999877096428, -47.40192378864679768 ) ) ;
#1861=CARTESIAN_POINT ( 'NONE',  ( 229.8435696437499871, -34.67812499938547433, 98.40857419181659793 ) ) ;
#1862=CARTESIAN_POINT ( 'NONE',  ( 233.9782151781249411, -32.09062499938547575, 97.61286128772489690 ) ) ;
#1879=DIRECTION ( 'NONE',  ( -1.000000000000000000, 0.000000000000000000, 0.000000000000000000 ) ) ;
#1880=CARTESIAN_POINT ( 'NONE',  ( 235.3564303562499447, -33.55312499938548143, 101.5914258081833879 ) ) ;
#1884=VERTEX_POINT ( 'NONE', #13516 ) ;
#1886=CARTESIAN_POINT ( 'NONE',  ( 234.0999999999999375, -31.49999999999999289, -52.59807621135342970 ) ) ;
#1890=CARTESIAN_POINT ( 'NONE',  ( 229.8435696437499303, -33.40312499938547575, 99.99999999999998579 ) ) ;
#1892=CARTESIAN_POINT ( 'NONE',  ( 231.2217848218749339, -33.02812499938547575, -52.38713871227520968 ) ) ;
#1894=VERTEX_POINT ( 'NONE', #2969 ) ;
#1896=CARTESIAN_POINT ( 'NONE',  ( 235.3564303562499447, -34.41562499938547859, 99.99999999999998579 ) ) ;
#1898=CARTESIAN_POINT ( 'NONE',  ( 229.8538686580537558, -31.99999999999998579, -50.29785994008192773 ) ) ;
#1903=CARTESIAN_POINT ( 'NONE',  ( 229.8435696437499871, -31.00312499938547361, -48.40857419181671162 ) ) ;
#1908=CARTESIAN_POINT ( 'NONE',  ( 235.5999999999999943, -34.23749999999999716, 98.26794919243110371 ) ) ;
#1910=( BOUNDED_CURVE ( )  B_SPLINE_CURVE ( 2, ( #13585, #7248, #4614, #10570, #226, #1587, #9190, #8810, #14765 ),
 .UNSPECIFIED., .F., .F. ) 
 B_SPLINE_CURVE_WITH_KNOTS ( ( 3, 2, 2, 2, 3 ),
 ( 0.6875000000000000000, 0.6944444444444444198, 0.7083333333333333703, 0.7222222222222222099, 0.7291666666666667407 ),
 .UNSPECIFIED. ) 
 CURVE ( )  GEOMETRIC_REPRESENTATION_ITEM ( )  RATIONAL_B_SPLINE_CURVE ( ( 0.9330127018922194093, 0.9330127018922194093, 1.000000000000000000, 0.8660254037844387076, 1.000000000000000000, 0.8660254037844387076, 1.000000000000000000, 0.9330127018922187432, 0.9330127018922192983 ) ) 
 REPRESENTATION_ITEM ( '' )  );
#1917=CARTESIAN_POINT ( 'NONE',  ( 232.5999999999999375, -32.98124999877095576, -47.00000000000011369 ) ) ;
#1918=CARTESIAN_POINT ( 'NONE',  ( 235.3564303562499447, -33.59062499938548285, 98.40857419181659793 ) ) ;
#1921=CARTESIAN_POINT ( 'NONE',  ( 244.7999999999999545, -35.00000000000000000, 150.0000000000000000 ) ) ;
#1923=CARTESIAN_POINT ( 'NONE',  ( 229.9620029755566293, -32.00000000000000711, 99.18121545504293124 ) ) ;
#1924=DIRECTION ( 'NONE',  ( 0.000000000000000000, 0.000000000000000000, -1.000000000000000000 ) ) ;
#1927=DIRECTION ( 'NONE',  ( -0.000000000000000000, -1.000000000000000000, -0.000000000000000000 ) ) ;
#1929=VECTOR ( 'NONE', #11797, 1000.000000000000000 ) ;
#1932=CARTESIAN_POINT ( 'NONE',  ( 231.2217848218749339, -33.02812499938547575, -52.38713871227520968 ) ) ;
#1934=CARTESIAN_POINT ( 'NONE',  ( 232.5999999999999375, -32.61562499938548143, 96.81714838363319586 ) ) ;
#1935=CARTESIAN_POINT ( 'NONE',  ( 231.2217848218749339, -31.22812499938547859, -52.38713871227520968 ) ) ;
#1953=CARTESIAN_POINT ( 'NONE',  ( 231.0999999999999375, -33.91874999877096286, -47.40192378864679768 ) ) ;
#1955=CARTESIAN_POINT ( 'NONE',  ( 231.2217848218749339, -34.71562499938547575, 97.61286128772489690 ) ) ;
#1958=FILL_AREA_STYLE_COLOUR ( '', #14898 ) ;
#1963=B_SPLINE_CURVE_WITH_KNOTS ( 'NONE', 3,
 ( #14159, #9866, #2440, #3801, #15539, #793, #3611, #6750, #16907, #15731, #15438, #2154, #6850, #15827, #18670, #11130, #12795, #5286 ),
 .UNSPECIFIED., .F., .F.,
 ( 4, 2, 2, 2, 2, 2, 2, 2, 4 ),
 ( 0.000000000000000000, 0.0007106627595359821031, 0.001421325519071964206, 0.002131988278607946201, 0.002842651038143928412, 0.003553313797679910624, 0.004263976557215892402, 0.004974639316751875047, 0.005685302076287856825 ),
 .UNSPECIFIED. ) ;
#1971=VERTEX_POINT ( 'NONE', #6206 ) ;
#1978=CARTESIAN_POINT ( 'NONE',  ( 105.1999999999999744, -4.999999999999976907, 153.0000000000000000 ) ) ;
#1984=CARTESIAN_POINT ( 'NONE',  ( 232.5999999999999375, -32.36249999999999716, -53.46410161513786363 ) ) ;
#1988=CARTESIAN_POINT ( 'NONE',  ( 229.8435696437499587, -32.54062499938547859, 98.40857419181659793 ) ) ;
#1991=CARTESIAN_POINT ( 'NONE',  ( 235.3564303562499447, -32.31562499938547717, -48.40857419181671162 ) ) ;
#1995=CARTESIAN_POINT ( 'NONE',  ( 232.5999999999999375, -29.99999999999999645, -50.00000000000011369 ) ) ;
#2004=VERTEX_POINT ( 'NONE', #1516 ) ;
#2006=CARTESIAN_POINT ( 'NONE',  ( 235.5999999999999943, -34.31249999999999289, 101.7320508075688537 ) ) ;
#2010=ORIENTED_EDGE ( 'NONE', *, *, #7677, .T. ) ;
#2012=CARTESIAN_POINT ( 'NONE',  ( 229.5999999999999375, -34.44374999877096144, -50.00000000000011369 ) ) ;
#2015=CARTESIAN_POINT ( 'NONE',  ( 229.8435696437499303, -33.85312499938548569, 99.99999999999998579 ) ) ;
#2019=DIRECTION ( 'NONE',  ( 0.000000000000000000, 0.000000000000000000, 1.000000000000000000 ) ) ;
#2020=CARTESIAN_POINT ( 'NONE',  ( 230.5523683116323355, -32.00000000000000000, 101.8452947671440540 ) ) ;
#2024=CARTESIAN_POINT ( 'NONE',  ( 232.5999999999999375, -32.36249999999999716, -53.00000000000011369 ) ) ;
#2026=EDGE_LOOP ( 'NONE', ( #49, #19244, #4813, #12099, #5239 ) ) ;
#2030=CARTESIAN_POINT ( 'NONE',  ( 232.5999999999999375, -33.06562499938547717, 96.81714838363319586 ) ) ;
#2031=CARTESIAN_POINT ( 'NONE',  ( 235.3564303562499447, -30.96562499938547930, -48.40857419181671162 ) ) ;
#2033=CARTESIAN_POINT ( 'NONE',  ( 235.5999999999999375, -34.72499999999999432, -50.00000000000011369 ) ) ;
#2035=ORIENTED_EDGE ( 'NONE', *, *, #14754, .F. ) ;
#2038=PLANE ( 'NONE',  #2554 ) ;
#2048=CARTESIAN_POINT ( 'NONE',  ( 232.5999999999999091, -34.10624999877096286, -53.00000000000010658 ) ) ;
#2050=CARTESIAN_POINT ( 'NONE',  ( 233.9782151781249411, -34.94062499938547717, 102.3871387122750889 ) ) ;
#2051=ORIENTED_EDGE ( 'NONE', *, *, #2656, .F. ) ;
#2053=LINE ( 'NONE', #5291, #15203 ) ;
#2065=( BOUNDED_CURVE ( )  B_SPLINE_CURVE ( 2, ( #8023, #432, #13983, #6377, #12426, #6569, #18394, #2169, #11050 ),
 .UNSPECIFIED., .F., .F. ) 
 B_SPLINE_CURVE_WITH_KNOTS ( ( 3, 2, 2, 2, 3 ),
 ( 0.6041666666666667407, 0.6111111111111111605, 0.6250000000000000000, 0.6388888888888888395, 0.6458333333333332593 ),
 .UNSPECIFIED. ) 
 CURVE ( )  GEOMETRIC_REPRESENTATION_ITEM ( )  RATIONAL_B_SPLINE_CURVE ( ( 0.9330127018922192983, 0.9330127018922198534, 1.000000000000000000, 0.8660254037844387076, 1.000000000000000000, 0.8660254037844387076, 1.000000000000000000, 0.9330127018922198534, 0.9330127018922192983 ) ) 
 REPRESENTATION_ITEM ( '' )  );
#2073=LINE ( 'NONE', #8030, #8496 ) ;
#2080=CARTESIAN_POINT ( 'NONE',  ( 229.5999999999999375, -32.28750000000000142, -51.73205080756898866 ) ) ;
#2085=CARTESIAN_POINT ( 'NONE',  ( 229.8435696437499303, -32.95312499938548001, 99.99999999999998579 ) ) ;
#2087=CARTESIAN_POINT ( 'NONE',  ( 235.3564303562499447, -32.72812499938547859, -50.00000000000011369 ) ) ;
#2088=EDGE_CURVE ( 'NONE', #3907, #1884, #3065, .T. ) ;
#2091=CARTESIAN_POINT ( 'NONE',  ( 232.5999999999999375, -33.71249999999999147, -53.00000000000010658 ) ) ;
#2101=CARTESIAN_POINT ( 'NONE',  ( 232.5999999999999375, -32.81249999999999289, -53.00000000000011369 ) ) ;
#2116=LINE ( 'NONE', #15402, #14711 ) ;
#2119=CARTESIAN_POINT ( 'NONE',  ( 233.9782151781249411, -34.60312499938548569, 102.3871387122750889 ) ) ;
#2121=AXIS2_PLACEMENT_3D ( 'NONE', #12853, #8358, #12655 ) ;
#2126=CARTESIAN_POINT ( 'NONE',  ( 230.1427008797911640, -31.99999999999999289, 101.2614033343866424 ) ) ;
#2127=CARTESIAN_POINT ( 'NONE',  ( 232.5999999999999375, -33.88124999877096855, 103.0000000000000000 ) ) ;
#2131=CARTESIAN_POINT ( 'NONE',  ( 231.6691923799541826, -35.05289549976082952, 96.44210921874548603 ) ) ;
#2133=ORIENTED_EDGE ( 'NONE', *, *, #8502, .T. ) ;
#2136=CARTESIAN_POINT ( 'NONE',  ( 232.5999999999999375, -31.49062499938547788, 103.1828516163667899 ) ) ;
#2137=CARTESIAN_POINT ( 'NONE',  ( 229.5999999999999375, -34.85624999877096286, -48.26794919243123161 ) ) ;
#2140=ORIENTED_EDGE ( 'NONE', *, *, #19313, .T. ) ;
#2153=CARTESIAN_POINT ( 'NONE',  ( 232.5999999999999659, -32.53124999877096712, 102.9999999999999858 ) ) ;
#2154=CARTESIAN_POINT ( 'NONE',  ( 232.1383900424027900, -31.99999999999999289, 102.8104067583494157 ) ) ;
#2155=CARTESIAN_POINT ( 'NONE',  ( 229.8435696437499871, -33.25312499938547717, 101.5914258081833879 ) ) ;
#2159=CARTESIAN_POINT ( 'NONE',  ( 231.0999999999999375, -32.11874999877096570, 102.5980762113533018 ) ) ;
#2162=FACE_OUTER_BOUND ( 'NONE', #18529, .T. ) ;
#2163=CARTESIAN_POINT ( 'NONE',  ( 246.9999999999999716, -29.80000000000000426, -100.0000000000000000 ) ) ;
#2169=CARTESIAN_POINT ( 'NONE',  ( 233.4038475772933339, -33.46740381056766012, -47.00000000000011369 ) ) ;
#2171=DIRECTION ( 'NONE',  ( 0.000000000000000000, 0.000000000000000000, -1.000000000000000000 ) ) ;
#2174=CARTESIAN_POINT ( 'NONE',  ( 232.5999999999999375, -32.75624999877096144, 96.99999999999998579 ) ) ;
#2185=CARTESIAN_POINT ( 'NONE',  ( 232.5999999999999943, -33.29062499938547859, 103.1828516163667899 ) ) ;
#2187=CARTESIAN_POINT ( 'NONE',  ( 233.9782151781249411, -34.90312499938547575, -52.38713871227520968 ) ) ;
#2191=DIRECTION ( 'NONE',  ( 0.000000000000000000, 0.000000000000000000, -1.000000000000000000 ) ) ;
#2198=CARTESIAN_POINT ( 'NONE',  ( 235.3564303562499447, -32.12812499938547717, -51.59142580818350865 ) ) ;
#2200=ADVANCED_FACE ( 'NONE', ( #18217 ), #13998, .F. ) ;
#2209=CARTESIAN_POINT ( 'NONE',  ( 232.5999999999999375, -34.55624999877095860, -53.00000000000011369 ) ) ;
#2210=CARTESIAN_POINT ( 'NONE',  ( 231.3931070460713499, -35.00000000000000000, -52.75353082432724960 ) ) ;
#2212=CARTESIAN_POINT ( 'NONE',  ( 229.8435696437499303, -32.39062499938548001, 99.99999999999998579 ) ) ;
#2220=ORIENTED_EDGE ( 'NONE', *, *, #14527, .T. ) ;
#2221=CARTESIAN_POINT ( 'NONE',  ( 231.2217848218749339, -34.67812499938548143, -47.61286128772501769 ) ) ;
#2223=CARTESIAN_POINT ( 'NONE',  ( 233.9782151781249411, -33.55312499938548143, 97.61286128772489690 ) ) ;
#2224=CARTESIAN_POINT ( 'NONE',  ( 235.3564303562499447, -34.04062499938547859, -51.59142580818350865 ) ) ;
#2235=CARTESIAN_POINT ( 'NONE',  ( 232.5999999999999375, -33.20624999877097139, -53.00000000000011369 ) ) ;
#2239=FACE_OUTER_BOUND ( 'NONE', #2585, .T. ) ;
#2242=CARTESIAN_POINT ( 'NONE',  ( 231.2217848218749339, -33.66562499938547859, 102.3871387122750889 ) ) ;
#2246=CARTESIAN_POINT ( 'NONE',  ( 235.5999999999999943, -31.55624999877096215, 101.7320508075688537 ) ) ;
#2249=CARTESIAN_POINT ( 'NONE',  ( 229.5999999999999375, -34.46249999999999147, 101.7320508075688821 ) ) ;
#2252=ORIENTED_EDGE ( 'NONE', *, *, #175, .F. ) ;
#2263=CARTESIAN_POINT ( 'NONE',  ( 229.5999999999999375, -33.18749999999999289, 98.26794919243111792 ) ) ;
#2264=CARTESIAN_POINT ( 'NONE',  ( 229.5999999999999375, -32.23124999877096286, -51.73205080756898866 ) ) ;
#2266=CARTESIAN_POINT ( 'NONE',  ( 246.9999999999999716, -5.000000000000004441, -100.0000000000000000 ) ) ;
#2272=ORIENTED_EDGE ( 'NONE', *, *, #12971, .F. ) ;
#2273=CARTESIAN_POINT ( 'NONE',  ( 232.5999999999999375, -29.99999999999999645, 96.99999999999998579 ) ) ;
#2276=CARTESIAN_POINT ( 'NONE',  ( 231.0999999999999375, -34.87499999999999289, -47.40192378864679768 ) ) ;
#2278=CARTESIAN_POINT ( 'NONE',  ( 235.3564303562499447, -35.01562499938548001, -48.40857419181671162 ) ) ;
#2285=CARTESIAN_POINT ( 'NONE',  ( 230.7186334667984227, -32.00000000000000711, -52.01453922190813728 ) ) ;
#2290=CARTESIAN_POINT ( 'NONE',  ( 231.2217848218749339, -32.76562499938548001, -47.61286128772501769 ) ) ;
#2307=CARTESIAN_POINT ( 'NONE',  ( 235.5999999999999943, -32.88749999999999574, 98.26794919243110371 ) ) ;
#2310=FACE_OUTER_BOUND ( 'NONE', #8168, .T. ) ;
#2311=CARTESIAN_POINT ( 'NONE',  ( 232.3466685930879123, -34.99995246259152282, -52.98928446312130802 ) ) ;
#2318=CARTESIAN_POINT ( 'NONE',  ( 229.8435696437499871, -34.79062499938547859, 98.40857419181659793 ) ) ;
#2319=CARTESIAN_POINT ( 'NONE',  ( 229.8435696437499303, -33.85312499938548569, -50.00000000000011369 ) ) ;
#2325=EDGE_CURVE ( 'NONE', #17759, #5681, #5512, .T. ) ;
#2331=CARTESIAN_POINT ( 'NONE',  ( 233.9782151781249411, -30.40312499938547930, 97.61286128772489690 ) ) ;
#2339=CARTESIAN_POINT ( 'NONE',  ( 231.0999999999999375, -32.32499999999999574, 97.40192378864668399 ) ) ;
#2343=CARTESIAN_POINT ( 'NONE',  ( 231.0999999999999375, -30.46874999877096002, 97.40192378864668399 ) ) ;
#2344=CARTESIAN_POINT ( 'NONE',  ( 235.5999999999999943, -31.93124999877096570, -51.73205080756900287 ) ) ;
#2348=ORIENTED_EDGE ( 'NONE', *, *, #12952, .T. ) ;
#2351=DIRECTION ( 'NONE',  ( 1.000000000000000000, 0.000000000000000000, 4.163336342344333240E-14 ) ) ;
#2367=CARTESIAN_POINT ( 'NONE',  ( 232.5999999999999375, -34.16249999999999432, -53.46410161513786363 ) ) ;
#2370=FACE_OUTER_BOUND ( 'NONE', #17466, .T. ) ;
#2372=CARTESIAN_POINT ( 'NONE',  ( 233.9782151781249411, -34.60312499938548569, -47.61286128772501769 ) ) ;
#2387=CARTESIAN_POINT ( 'NONE',  ( 231.2217848218749339, -32.91562499938547148, -52.38713871227520968 ) ) ;
#2390=ORIENTED_EDGE ( 'NONE', *, *, #9593, .F. ) ;
#2396=CARTESIAN_POINT ( 'NONE',  ( 246.9999999999999716, -29.80000000000000426, -100.0000000000000000 ) ) ;
#2407=CARTESIAN_POINT ( 'NONE',  ( 231.4797793666089945, -32.00000000000000711, 97.42682425340032637 ) ) ;
#2408=AXIS2_PLACEMENT_3D ( 'NONE', #5217, #10778, #15666 ) ;
#2415=CARTESIAN_POINT ( 'NONE',  ( 229.8435696437499303, -33.85312499938548569, 99.99999999999998579 ) ) ;
#2416=CARTESIAN_POINT ( 'NONE',  ( 233.9782151781249411, -32.20312499938548001, -52.38713871227520968 ) ) ;
#2421=CARTESIAN_POINT ( 'NONE',  ( 233.4038475772933054, -34.12634618820329280, 96.99999999999997158 ) ) ;
#2426=ORIENTED_EDGE ( 'NONE', *, *, #3306, .F. ) ;
#2434=CIRCLE ( 'NONE', #8986, 5.199999999999996625 ) ;
#2438=CARTESIAN_POINT ( 'NONE',  ( 231.7961524227065695, -32.34240381056765301, -53.00000000000011369 ) ) ;
#2440=CARTESIAN_POINT ( 'NONE',  ( 235.0681666926251694, -31.99999999999997158, 101.6855250459193627 ) ) ;
#2441=CARTESIAN_POINT ( 'NONE',  ( 229.5999999999999375, -29.99999999999999645, 99.99999999999998579 ) ) ;
#2442=EDGE_LOOP ( 'NONE', ( #18, #13707, #1278 ) ) ;
#2445=CARTESIAN_POINT ( 'NONE',  ( 232.5999999999999375, -32.53124999877096002, 103.4641016151377499 ) ) ;
#2446=CARTESIAN_POINT ( 'NONE',  ( 229.5999999999999375, -30.43124999877096215, -51.73205080756898866 ) ) ;
#2452=CARTESIAN_POINT ( 'NONE',  ( 232.5999999999999375, -33.65624999877096002, 97.00000000000000000 ) ) ;
#2460=CARTESIAN_POINT ( 'NONE',  ( 235.0804598586380507, -35.00000000000002132, -51.44276241308963193 ) ) ;
#2461=CARTESIAN_POINT ( 'NONE',  ( 234.3965303555545461, -31.99999999999998579, -52.32517275847976634 ) ) ;
#2467=CARTESIAN_POINT ( 'NONE',  ( 233.4038475772933339, -32.06115380933863435, -47.00000000000011369 ) ) ;
#2470=CARTESIAN_POINT ( 'NONE',  ( 233.9782151781249411, -33.70312499938548001, 102.3871387122750889 ) ) ;
#2472=CARTESIAN_POINT ( 'NONE',  ( 231.2217848218749339, -31.56562499938547717, -52.38713871227520968 ) ) ;
#2483=CARTESIAN_POINT ( 'NONE',  ( 232.5999999999999375, -33.62812499938547717, -46.81714838363331666 ) ) ;
#2494=CARTESIAN_POINT ( 'NONE',  ( 232.5999999999999943, -32.05312499938548143, 96.81714838363319586 ) ) ;
#2502=CARTESIAN_POINT ( 'NONE',  ( 235.3193635794330874, -31.99999999999998579, 98.73478688818596538 ) ) ;
#2503=EDGE_CURVE ( 'NONE', #2622, #2968, #1394, .T. ) ;
#2509=CARTESIAN_POINT ( 'NONE',  ( 233.5505106857032729, -35.00000000000002132, -47.40655328406458580 ) ) ;
#2510=CARTESIAN_POINT ( 'NONE',  ( 229.8435696437499871, -32.09062499938548285, -51.59142580818350865 ) ) ;
#2512=DIRECTION ( 'NONE',  ( -0.000000000000000000, 0.000000000000000000, -1.000000000000000000 ) ) ;
#2513=ORIENTED_EDGE ( 'NONE', *, *, #4747, .F. ) ;
#2516=ORIENTED_EDGE ( 'NONE', *, *, #15618, .F. ) ;
#2520=CARTESIAN_POINT ( 'NONE',  ( 246.9999999999999716, -5.000000000000004441, -100.0000000000000000 ) ) ;
#2526=CARTESIAN_POINT ( 'NONE',  ( 232.5999999999999375, -31.91249999999999432, 96.53589838486223584 ) ) ;
#2528=CARTESIAN_POINT ( 'NONE',  ( 235.5999999999999943, -34.70624999877096428, 101.7320508075688537 ) ) ;
#2529=CARTESIAN_POINT ( 'NONE',  ( 232.5999999999999375, -32.75624999877096144, 96.53589838486223584 ) ) ;
#2530=CARTESIAN_POINT ( 'NONE',  ( 229.5999999999999375, -31.29374999877096286, -50.00000000000011369 ) ) ;
#2533=ORIENTED_EDGE ( 'NONE', *, *, #6272, .F. ) ;
#2545=EDGE_CURVE ( 'NONE', #18744, #15781, #14514, .T. ) ;
#2546=CARTESIAN_POINT ( 'NONE',  ( 231.7961524227065695, -32.28615380933862156, -53.00000000000011369 ) ) ;
#2551=CARTESIAN_POINT ( 'NONE',  ( 229.5999999999999375, -34.53749999999999432, -51.73205080756898866 ) ) ;
#2554=AXIS2_PLACEMENT_3D ( 'NONE', #5082, #11024, #13955 ) ;
#2559=CARTESIAN_POINT ( 'NONE',  ( 232.5999999999999375, -30.25312499938548072, -53.18285161636690361 ) ) ;
#2560=EDGE_CURVE ( 'NONE', #17012, #5681, #1910, .T. ) ;
#2568=CARTESIAN_POINT ( 'NONE',  ( 233.9782151781249411, -32.54062499938547859, 97.61286128772489690 ) ) ;
#2575=ADVANCED_FACE ( 'NONE', ( #8900 ), #4713, .F. ) ;
#2576=CARTESIAN_POINT ( 'NONE',  ( 229.8435696437499871, -34.15312499938547575, -48.40857419181671162 ) ) ;
#2581=DIRECTION ( 'NONE',  ( -0.000000000000000000, -1.000000000000000000, -0.000000000000000000 ) ) ;
#2585=EDGE_LOOP ( 'NONE', ( #7926, #17793, #18316 ) ) ;
#2587=CARTESIAN_POINT ( 'NONE',  ( 235.3564303562499447, -33.06562499938547717, 99.99999999999998579 ) ) ;
#2591=DIRECTION ( 'NONE',  ( 1.000000000000000000, 0.000000000000000000, 0.000000000000000000 ) ) ;
#2596=CARTESIAN_POINT ( 'NONE',  ( 233.7735609739808353, -32.00000000000002132, 97.33634050170194030 ) ) ;
#2597=CARTESIAN_POINT ( 'NONE',  ( 105.2000000000001307, -29.80000000000002203, 147.7999999999999829 ) ) ;
#2603=CARTESIAN_POINT ( 'NONE',  ( 233.9782151781249411, -34.45312499938548001, 97.61286128772489690 ) ) ;
#2604=CARTESIAN_POINT ( 'NONE',  ( 231.2217848218749339, -33.92812499938548143, -52.38713871227520968 ) ) ;
#2611=ORIENTED_EDGE ( 'NONE', *, *, #17471, .T. ) ;
#2618=LINE ( 'NONE', #8579, #19133 ) ;
#2621=CARTESIAN_POINT ( 'NONE',  ( 234.0999999999999375, -30.74999999999999645, 102.5980762113533018 ) ) ;
#2622=VERTEX_POINT ( 'NONE', #13203 ) ;
#2623=CARTESIAN_POINT ( 'NONE',  ( 231.2217848218749339, -32.12812499938547717, -52.38713871227520968 ) ) ;
#2625=CARTESIAN_POINT ( 'NONE',  ( 235.5999999999999375, -32.41874999877096286, 99.99999999999998579 ) ) ;
#2626=CARTESIAN_POINT ( 'NONE',  ( 235.5999999999999943, -31.48124999877096286, -51.73205080756900287 ) ) ;
#2629=EDGE_LOOP ( 'NONE', ( #3384, #9873, #14255, #8421 ) ) ;
#2633=ORIENTED_EDGE ( 'NONE', *, *, #645, .T. ) ;
#2647=CARTESIAN_POINT ( 'NONE',  ( 235.3058334582607074, -35.00000000000002132, 100.6274906301342327 ) ) ;
#2655=CARTESIAN_POINT ( 'NONE',  ( 229.8435696437499303, -32.84062499938547575, -50.00000000000011369 ) ) ;
#2656=EDGE_CURVE ( 'NONE', #15452, #3491, #13298, .T. ) ;
#2663=CARTESIAN_POINT ( 'NONE',  ( 235.3564303562499447, -30.32812499938548001, 98.40857419181659793 ) ) ;
#2664=CARTESIAN_POINT ( 'NONE',  ( 233.9782151781249411, -32.24062499938548143, -47.61286128772501769 ) ) ;
#2670=CARTESIAN_POINT ( 'NONE',  ( 232.5999999999999375, -30.78749999999999432, -46.53589838486234953 ) ) ;
#2674=ADVANCED_FACE ( 'NONE', ( #2162 ), #424, .T. ) ;
#2691=LINE ( 'NONE', #11299, #11643 ) ;
#2694=CARTESIAN_POINT ( 'NONE',  ( 230.7186334667983658, -32.00000000000000711, 97.98546077809203325 ) ) ;
#2695=CARTESIAN_POINT ( 'NONE',  ( 231.7961524227065411, -33.05759618943232425, -47.00000000000012790 ) ) ;
#2697=CARTESIAN_POINT ( 'NONE',  ( 229.5999999999999375, -34.04999999999999716, 99.99999999999998579 ) ) ;
#2701=CARTESIAN_POINT ( 'NONE',  ( 233.9782151781249411, -34.90312499938547575, 97.61286128772489690 ) ) ;
#2703=CARTESIAN_POINT ( 'NONE',  ( 235.3564303562499447, -34.52812499938547575, -50.00000000000011369 ) ) ;
#2709=AXIS2_PLACEMENT_3D ( 'NONE', #15635, #9768, #11129 ) ;
#2711=ORIENTED_EDGE ( 'NONE', *, *, #8413, .T. ) ;
#2716=CARTESIAN_POINT ( 'NONE',  ( 231.2217848218749339, -32.12812499938547717, 97.61286128772489690 ) ) ;
#2721=FACE_OUTER_BOUND ( 'NONE', #1011, .T. ) ;
#2725=CARTESIAN_POINT ( 'NONE',  ( 234.0999999999999375, -30.14999999999999503, 97.40192378864668399 ) ) ;
#2726=( BOUNDED_CURVE ( )  B_SPLINE_CURVE ( 2, ( #11190, #17153, #3761, #15690, #4440, #16459, #5816, #2782, #8833 ),
 .UNSPECIFIED., .F., .F. ) 
 B_SPLINE_CURVE_WITH_KNOTS ( ( 3, 2, 2, 2, 3 ),
 ( 0.4375000000000001110, 0.4444444444444444198, 0.4583333333333333148, 0.4722222222222222099, 0.4791666666666666852 ),
 .UNSPECIFIED. ) 
 CURVE ( )  GEOMETRIC_REPRESENTATION_ITEM ( )  RATIONAL_B_SPLINE_CURVE ( ( 0.9330127018922194093, 0.9330127018922204085, 1.000000000000000000, 0.8660254037844387076, 1.000000000000000000, 0.8660254037844387076, 1.000000000000000000, 0.9330127018922190762, 0.9330127018922194093 ) ) 
 REPRESENTATION_ITEM ( '' )  );
#2727=ORIENTED_EDGE ( 'NONE', *, *, #13319, .T. ) ;
#2729=CARTESIAN_POINT ( 'NONE',  ( 232.5999999999999375, -33.20624999877095718, 96.53589838486223584 ) ) ;
#2730=CARTESIAN_POINT ( 'NONE',  ( 234.0999999999999375, -33.69374999877096144, -52.59807621135342970 ) ) ;
#2733=ORIENTED_EDGE ( 'NONE', *, *, #2503, .T. ) ;
#2735=DIRECTION ( 'NONE',  ( 0.000000000000000000, 0.000000000000000000, 1.000000000000000000 ) ) ;
#2737=DIRECTION ( 'NONE',  ( -1.000000000000000000, 6.244088828561840598E-46, 1.735459783503185124E-31 ) ) ;
#2742=VECTOR ( 'NONE', #8367, 1000.000000000000000 ) ;
#2745=CARTESIAN_POINT ( 'NONE',  ( 233.4038475772933054, -32.51115380933862298, -47.00000000000010658 ) ) ;
#2754=CARTESIAN_POINT ( 'NONE',  ( 232.5999999999999375, -33.20624999877097139, -53.00000000000011369 ) ) ;
#2755=VECTOR ( 'NONE', #4872, 1000.000000000000000 ) ;
#2756=AXIS2_PLACEMENT_3D ( 'NONE', #6720, #16883, #1834 ) ;
#2758=CARTESIAN_POINT ( 'NONE',  ( 235.2218879900010791, -35.00000000000000000, 100.8506536761482124 ) ) ;
#2761=CARTESIAN_POINT ( 'NONE',  ( 233.9782151781249411, -32.09062499938547575, -52.38713871227520968 ) ) ;
#2766=CARTESIAN_POINT ( 'NONE',  ( 232.5999999999999375, -33.43124999877096570, -47.00000000000011369 ) ) ;
#2770=CARTESIAN_POINT ( 'NONE',  ( 231.2217848218749339, -30.51562499938548001, 102.3871387122750889 ) ) ;
#2771=CARTESIAN_POINT ( 'NONE',  ( 235.3564303562499447, -34.90312499938547575, -48.40857419181671162 ) ) ;
#2777=CARTESIAN_POINT ( 'NONE',  ( 229.5999999999999375, -30.03749999999999432, -51.73205080756898866 ) ) ;
#2782=CARTESIAN_POINT ( 'NONE',  ( 233.4038475772933054, -32.96115380933862582, 102.9999999999999858 ) ) ;
#2783=CARTESIAN_POINT ( 'NONE',  ( 232.5999999999999375, -31.71562499938547930, -53.18285161636690361 ) ) ;
#2794=CARTESIAN_POINT ( 'NONE',  ( 233.9825576637931022, -32.00000000000000000, -47.41649131116869853 ) ) ;
#2796=CARTESIAN_POINT ( 'NONE',  ( 232.5999999999999375, -33.93749999999999289, -47.00000000000011369 ) ) ;
#2800=CARTESIAN_POINT ( 'NONE',  ( 229.5999999999999375, -34.93124999877095860, 98.26794919243111792 ) ) ;
#2806=CARTESIAN_POINT ( 'NONE',  ( 233.9782151781249411, -34.45312499938548001, -52.38713871227520968 ) ) ;
#2807=CARTESIAN_POINT ( 'NONE',  ( 235.5999999999999943, -34.25624999877096144, 101.7320508075688537 ) ) ;
#2809=ORIENTED_EDGE ( 'NONE', *, *, #14777, .T. ) ;
#2815=CARTESIAN_POINT ( 'NONE',  ( 231.7961524227065695, -34.59240381056765301, -53.00000000000011369 ) ) ;
#2817=CARTESIAN_POINT ( 'NONE',  ( 231.2217848218749339, -31.22812499938547859, 97.61286128772489690 ) ) ;
#2820=CARTESIAN_POINT ( 'NONE',  ( 234.0999999999999375, -33.84374999877096002, 102.5980762113533018 ) ) ;
#2821=CARTESIAN_POINT ( 'NONE',  ( -1.788378118793200470E-29, -3.597944987211158634E-13, -100.0000000000001137 ) ) ;
#2822=CARTESIAN_POINT ( 'NONE',  ( 232.5999999999999375, -33.43124999877096570, 102.9999999999999858 ) ) ;
#2824=CARTESIAN_POINT ( 'NONE',  ( 234.0999999999999375, -34.19999999999999574, 97.40192378864668399 ) ) ;
#2829=CARTESIAN_POINT ( 'NONE',  ( 234.0999999999999375, -31.89374999877096073, 97.40192378864668399 ) ) ;
#2830=CARTESIAN_POINT ( 'NONE',  ( 235.5999999999999943, -33.28124999877096002, -51.73205080756900287 ) ) ;
#2833=ORIENTED_EDGE ( 'NONE', *, *, #4119, .T. ) ;
#2836=ORIENTED_EDGE ( 'NONE', *, *, #10425, .F. ) ;
#2842=CARTESIAN_POINT ( 'NONE',  ( 233.9419434205216817, -35.00000000000000711, -52.61493892574790010 ) ) ;
#2843=CARTESIAN_POINT ( 'NONE',  ( 232.1470656674052577, -31.99999999999997868, -52.80109480795715626 ) ) ;
#2844=EDGE_CURVE ( 'NONE', #4900, #13568, #11392, .T. ) ;
#2849=VERTEX_POINT ( 'NONE', #10066 ) ;
#2857=CARTESIAN_POINT ( 'NONE',  ( 233.9782151781249411, -34.04062499938547859, -47.61286128772501769 ) ) ;
#2858=ORIENTED_EDGE ( 'NONE', *, *, #101, .F. ) ;
#2864=CARTESIAN_POINT ( 'NONE',  ( 102.9999999999999858, -29.80000000000000071, -100.0000000000000000 ) ) ;
#2865=CARTESIAN_POINT ( 'NONE',  ( 232.5999999999999375, -31.15312499938547930, 96.81714838363319586 ) ) ;
#2866=CARTESIAN_POINT ( 'NONE',  ( 235.3564303562499447, -34.00312499938547717, -48.40857419181671162 ) ) ;
#2871=CARTESIAN_POINT ( 'NONE',  ( 231.2217848218749339, -34.71562499938547575, -52.38713871227520968 ) ) ;
#2877=CARTESIAN_POINT ( 'NONE',  ( 231.2217848218749339, -30.62812499938548072, -47.61286128772501769 ) ) ;
#2883=CARTESIAN_POINT ( 'NONE',  ( 235.3564303562499447, -32.65312499938547575, 101.5914258081833879 ) ) ;
#2889=CARTESIAN_POINT ( 'NONE',  ( 229.7688980899111186, -34.99999999999998579, 99.14248198115953414 ) ) ;
#2896=( BOUNDED_CURVE ( )  B_SPLINE_CURVE ( 2, ( #13460, #96, #16591, #16499, #6048, #3101, #2820, #9060, #3196 ),
 .UNSPECIFIED., .F., .F. ) 
 B_SPLINE_CURVE_WITH_KNOTS ( ( 3, 2, 2, 2, 3 ),
 ( 0.6041666666666667407, 0.6111111111111111605, 0.6250000000000000000, 0.6388888888888888395, 0.6458333333333331483 ),
 .UNSPECIFIED. ) 
 CURVE ( )  GEOMETRIC_REPRESENTATION_ITEM ( )  RATIONAL_B_SPLINE_CURVE ( ( 0.9330127018922192983, 0.9330127018922198534, 1.000000000000000000, 0.8660254037844387076, 1.000000000000000000, 0.8660254037844387076, 1.000000000000000000, 0.9330127018922209636, 0.9330127018922194093 ) ) 
 REPRESENTATION_ITEM ( '' )  );
#2900=CARTESIAN_POINT ( 'NONE',  ( 229.8435696437499303, -34.75312499938547717, -50.00000000000011369 ) ) ;
#2906=EDGE_CURVE ( 'NONE', #18744, #9588, #16025, .T. ) ;
#2910=CARTESIAN_POINT ( 'NONE',  ( 231.0999999999999375, -34.57499999999999574, -52.59807621135342970 ) ) ;
#2912=CARTESIAN_POINT ( 'NONE',  ( 233.9782151781249411, -32.65312499938548285, 97.61286128772489690 ) ) ;
#2917=EDGE_CURVE ( 'NONE', #19255, #5568, #6165, .T. ) ;
#2919=CARTESIAN_POINT ( 'NONE',  ( 231.0999999999999375, -34.12499999999999289, 97.40192378864668399 ) ) ;
#2920=EDGE_CURVE ( 'NONE', #3185, #19282, #10647, .T. ) ;
#2923=CARTESIAN_POINT ( 'NONE',  ( 232.5999999999999375, -30.36562499938548498, 96.81714838363319586 ) ) ;
#2924=CARTESIAN_POINT ( 'NONE',  ( 234.0999999999999375, -34.59374999877096002, -52.59807621135342970 ) ) ;
#2931=DIRECTION ( 'NONE',  ( 0.000000000000000000, -1.000000000000000000, 0.000000000000000000 ) ) ;
#2942=CARTESIAN_POINT ( 'NONE',  ( 235.3564303562499447, -30.36562499938547788, 99.99999999999998579 ) ) ;
#2947=CARTESIAN_POINT ( 'NONE',  ( 229.5999999999999375, -34.48124999877096286, 98.26794919243111792 ) ) ;
#2949=LINE ( 'NONE', #5893, #17854 ) ;
#2951=CARTESIAN_POINT ( 'NONE',  ( 229.8435696437499871, -32.80312499938548143, -48.40857419181671162 ) ) ;
#2952=ORIENTED_EDGE ( 'NONE', *, *, #9274, .F. ) ;
#2953=ORIENTED_EDGE ( 'NONE', *, *, #1112, .F. ) ;
#2960=CARTESIAN_POINT ( 'NONE',  ( 235.3564303562499447, -33.02812499938547575, 98.40857419181659793 ) ) ;
#2961=CARTESIAN_POINT ( 'NONE',  ( 233.9782151781249411, -33.44062499938547717, -52.38713871227520968 ) ) ;
#2965=CARTESIAN_POINT ( 'NONE',  ( 235.5999999999999375, -30.22499999999999432, -50.00000000000011369 ) ) ;
#2968=VERTEX_POINT ( 'NONE', #4663 ) ;
#2969=CARTESIAN_POINT ( 'NONE',  ( 232.5999999999999375, -32.98124999877095576, 102.9999999999999858 ) ) ;
#2971=CARTESIAN_POINT ( 'NONE',  ( 233.9782151781249411, -31.00312499938548072, -47.61286128772501769 ) ) ;
#2974=CARTESIAN_POINT ( 'NONE',  ( 244.7999999999999545, -29.80000000000002203, -100.0000000000000142 ) ) ;
#2975=CARTESIAN_POINT ( 'NONE',  ( 235.3564303562499447, -34.90312499938547575, 101.5914258081833879 ) ) ;
#2979=LINE ( 'NONE', #10504, #7735 ) ;
#2984=CARTESIAN_POINT ( 'NONE',  ( 229.5999999999999375, -34.85624999877096286, 101.7320508075688821 ) ) ;
#2991=CARTESIAN_POINT ( 'NONE',  ( 229.8435696437499871, -35.22676544108146857, -51.00325357418267913 ) ) ;
#3001=CARTESIAN_POINT ( 'NONE',  ( 229.5999999999999375, -34.53749999999999432, -51.73205080756898866 ) ) ;
#3003=CARTESIAN_POINT ( 'NONE',  ( 232.5999999999999375, -31.94062499938548072, 103.1828516163667899 ) ) ;
#3011=CARTESIAN_POINT ( 'NONE',  ( 234.0999999999999375, -32.84999999999999432, 97.40192378864668399 ) ) ;
#3014=ORIENTED_EDGE ( 'NONE', *, *, #14640, .F. ) ;
#3015=CARTESIAN_POINT ( 'NONE',  ( 229.8435696437499587, -32.91562499938547859, -48.40857419181671162 ) ) ;
#3016=CARTESIAN_POINT ( 'NONE',  ( 235.5999999999999943, -35.08124999877096428, 98.26794919243110371 ) ) ;
#3017=CARTESIAN_POINT ( 'NONE',  ( 235.5999999999999375, -32.41874999877096286, -50.00000000000011369 ) ) ;
#3038=ORIENTED_EDGE ( 'NONE', *, *, #3467, .F. ) ;
#3046=CARTESIAN_POINT ( 'NONE',  ( 231.2217848218749339, -32.01562499938548001, -52.38713871227520968 ) ) ;
#3047=CIRCLE ( 'NONE', #12407, 5.200000000000009948 ) ;
#3048=ORIENTED_EDGE ( 'NONE', *, *, #6746, .F. ) ;
#3056=CARTESIAN_POINT ( 'NONE',  ( 229.8435696437499871, -33.70312499938548001, 101.5914258081833879 ) ) ;
#3061=ORIENTED_EDGE ( 'NONE', *, *, #14228, .F. ) ;
#3062=CARTESIAN_POINT ( 'NONE',  ( 235.5999999999999375, -30.67499999999999361, -50.00000000000011369 ) ) ;
#3065=LINE ( 'NONE', #5914, #6339 ) ;
#3072=CARTESIAN_POINT ( 'NONE',  ( 231.2217848218749339, -33.81562499938547717, 97.61286128772489690 ) ) ;
#3075=CARTESIAN_POINT ( 'NONE',  ( 235.4117376914898898, -32.00000000000000000, -51.04600724388262023 ) ) ;
#3078=CARTESIAN_POINT ( 'NONE',  ( 229.7064227204490408, -35.00000000000000711, 100.3154961327744985 ) ) ;
#3086=DIRECTION ( 'NONE',  ( -4.970554372426382520E-17, -1.000000000000000000, 3.491481338843133355E-15 ) ) ;
#3096=CARTESIAN_POINT ( 'NONE',  ( 231.7961524227065979, -33.63615380933863008, -53.00000000000011369 ) ) ;
#3097=CARTESIAN_POINT ( 'NONE',  ( 232.5999999999999375, -30.81562499938547717, 96.81714838363319586 ) ) ;
#3101=CARTESIAN_POINT ( 'NONE',  ( 235.5999999999999943, -33.80624999877096570, 101.7320508075688537 ) ) ;
#3102=MANIFOLD_SOLID_BREP ( 'Cavity1', #6354 ) ;
#3107=CARTESIAN_POINT ( 'NONE',  ( 234.0999999999999375, -33.44999999999999574, 102.5980762113533018 ) ) ;
#3108=ORIENTED_EDGE ( 'NONE', *, *, #19189, .F. ) ;
#3109=CARTESIAN_POINT ( 'NONE',  ( 235.3564303562499447, -32.72812499938547859, -50.00000000000011369 ) ) ;
#3110=CARTESIAN_POINT ( 'NONE',  ( 235.3564303562499447, -30.51562499938548001, 101.5914258081833879 ) ) ;
#3111=CARTESIAN_POINT ( 'NONE',  ( 235.5999999999999943, -32.83124999877095718, -51.73205080756900287 ) ) ;
#3113=ORIENTED_EDGE ( 'NONE', *, *, #4119, .F. ) ;
#3116=CARTESIAN_POINT ( 'NONE',  ( 231.0999999999999375, -34.87499999999999289, 102.5980762113533018 ) ) ;
#3120=CARTESIAN_POINT ( 'NONE',  ( 232.5999999999999375, -33.88124999877096855, 102.9999999999999858 ) ) ;
#3125=CARTESIAN_POINT ( 'NONE',  ( 232.5999999999999375, -33.48749999999999716, 103.0000000000000000 ) ) ;
#3129=CARTESIAN_POINT ( 'NONE',  ( 235.3564303562499447, -31.71562499938547575, 99.99999999999998579 ) ) ;
#3133=CARTESIAN_POINT ( 'NONE',  ( 234.0999999999999375, -33.39374999877096428, -47.40192378864679768 ) ) ;
#3134=CARTESIAN_POINT ( 'NONE',  ( 244.7999999999999545, -4.999999999999990230, -100.0000000000000995 ) ) ;
#3135=LINE ( 'NONE', #11935, #9599 ) ;
#3137=DIRECTION ( 'NONE',  ( 0.000000000000000000, 0.000000000000000000, -1.000000000000000000 ) ) ;
#3138=CARTESIAN_POINT ( 'NONE',  ( 229.8435696437499303, -35.09062499938547575, -50.00000000000011369 ) ) ;
#3139=EDGE_LOOP ( 'NONE', ( #16917, #3061, #16609, #1684 ) ) ;
#3143=EDGE_CURVE ( 'NONE', #8999, #13758, #9728, .T. ) ;
#3147=CARTESIAN_POINT ( 'NONE',  ( 232.5999999999999375, -34.75312499938547717, 96.81714838363319586 ) ) ;
#3148=CARTESIAN_POINT ( 'NONE',  ( 235.3564303562499447, -34.86562499938547433, -50.00000000000011369 ) ) ;
#3151=ORIENTED_EDGE ( 'NONE', *, *, #11313, .F. ) ;
#3152=CARTESIAN_POINT ( 'NONE',  ( 229.5999999999999375, -32.66249999999999432, -48.26794919243123161 ) ) ;
#3154=DIRECTION ( 'NONE',  ( 5.139921410301648824E-16, 1.000000000000000000, -3.597944987211154374E-15 ) ) ;
#3159=CARTESIAN_POINT ( 'NONE',  ( 229.8435696437499871, -30.29062499938548214, -51.59142580818350865 ) ) ;
#3165=CARTESIAN_POINT ( 'NONE',  ( 229.8435696437499303, -34.19062499938547717, 99.99999999999998579 ) ) ;
#3174=CARTESIAN_POINT ( 'NONE',  ( 232.5999999999999375, -31.37812499938547717, -46.81714838363331666 ) ) ;
#3185=VERTEX_POINT ( 'NONE', #9405 ) ;
#3192=CARTESIAN_POINT ( 'NONE',  ( 235.3564303562499447, -33.62812499938547717, 99.99999999999998579 ) ) ;
#3194=ORIENTED_EDGE ( 'NONE', *, *, #18015, .F. ) ;
#3196=CARTESIAN_POINT ( 'NONE',  ( 232.5999999999999375, -33.88124999877096855, 102.9999999999999858 ) ) ;
#3198=CARTESIAN_POINT ( 'NONE',  ( 105.1999999999999886, -29.79999999999997229, -103.0000000000000142 ) ) ;
#3199=VECTOR ( 'NONE', #12599, 1000.000000000000000 ) ;
#3202=CARTESIAN_POINT ( 'NONE',  ( 235.5999999999999375, -32.47499999999999432, 99.99999999999998579 ) ) ;
#3204=CARTESIAN_POINT ( 'NONE',  ( 231.2217848218749339, -33.47812499938547859, -52.38713871227520968 ) ) ;
#3206=CARTESIAN_POINT ( 'NONE',  ( 235.3564303562499447, -30.89062499938548001, 98.40857419181659793 ) ) ;
#3207=CARTESIAN_POINT ( 'NONE',  ( 232.5999999999999375, -35.00624999877096855, -53.46410161513786363 ) ) ;
#3211=VERTEX_POINT ( 'NONE', #14284 ) ;
#3212=CARTESIAN_POINT ( 'NONE',  ( 229.5999999999999375, -32.60624999877096286, -48.26794919243123161 ) ) ;
#3225=CARTESIAN_POINT ( 'NONE',  ( 105.1999999999999744, -29.80000000000000071, 150.0000000000000000 ) ) ;
#3226=CARTESIAN_POINT ( 'NONE',  ( 235.3564303562499447, -31.67812499938547788, 98.40857419181659793 ) ) ;
#3228=( NAMED_UNIT ( * ) SI_UNIT ( $, .STERADIAN. ) SOLID_ANGLE_UNIT ( ) );
#3232=CARTESIAN_POINT ( 'NONE',  ( 230.4006479041978821, -35.00000000000000711, -48.20719995774843625 ) ) ;
#3243=CARTESIAN_POINT ( 'NONE',  ( 232.5999999999999375, -34.52812499938548285, 103.1828516163667899 ) ) ;
#3245=EDGE_CURVE ( 'NONE', #15781, #10258, #9799, .T. ) ;
#3248=CARTESIAN_POINT ( 'NONE',  ( 229.5999999999999375, -33.56249999999999289, -48.26794919243123161 ) ) ;
#3255=CARTESIAN_POINT ( 'NONE',  ( 229.8435696437499871, -33.89062499938548001, -51.59142580818350865 ) ) ;
#3259=CARTESIAN_POINT ( 'NONE',  ( 233.9782151781249411, -34.79062499938547859, 97.61286128772489690 ) ) ;
#3262=EDGE_CURVE ( 'NONE', #5496, #1022, #7739, .T. ) ;
#3263=CARTESIAN_POINT ( 'NONE',  ( 234.0999999999999375, -34.64999999999999147, 97.40192378864668399 ) ) ;
#3270=CARTESIAN_POINT ( 'NONE',  ( 231.2217848218749339, -30.51562499938548001, -47.61286128772501769 ) ) ;
#3275=DIRECTION ( 'NONE',  ( 0.000000000000000000, 0.000000000000000000, 1.000000000000000000 ) ) ;
#3281=ORIENTED_EDGE ( 'NONE', *, *, #14640, .T. ) ;
#3283=CARTESIAN_POINT ( 'NONE',  ( 244.7999999999999545, -29.80000000000001492, -97.80000000000002558 ) ) ;
#3287=CARTESIAN_POINT ( 'NONE',  ( 235.3564303562499447, -34.56562499938547717, 101.5914258081833879 ) ) ;
#3293=AXIS2_PLACEMENT_3D ( 'NONE', #8549, #4164, #8840 ) ;
#3299=ORIENTED_EDGE ( 'NONE', *, *, #10930, .F. ) ;
#3300=CARTESIAN_POINT ( 'NONE',  ( 232.5999999999999943, -34.41562499938547859, -53.18285161636690361 ) ) ;
#3302=CARTESIAN_POINT ( 'NONE',  ( 234.0999999999999375, -34.74374999877096570, 102.5980762113533018 ) ) ;
#3303=CARTESIAN_POINT ( 'NONE',  ( 233.9782151781249411, -31.00312499938548072, -47.61286128772501769 ) ) ;
#3306=EDGE_CURVE ( 'NONE', #10687, #6930, #3916, .T. ) ;
#3310=DIRECTION ( 'NONE',  ( -0.000000000000000000, -1.000000000000000000, -0.000000000000000000 ) ) ;
#3318=DIRECTION ( 'NONE',  ( -1.000000000000000000, 4.625929269271485791E-17, 1.459037836657010301E-31 ) ) ;
#3321=CARTESIAN_POINT ( 'NONE',  ( 235.3564303562499447, -32.65312499938547575, 101.5914258081833879 ) ) ;
#3322=ORIENTED_EDGE ( 'NONE', *, *, #16294, .T. ) ;
#3330=CARTESIAN_POINT ( 'NONE',  ( 235.3564303562499447, -34.41562499938547859, -50.00000000000011369 ) ) ;
#3340=CARTESIAN_POINT ( 'NONE',  ( 229.8435696437499871, -35.05312499938547433, 101.5914258081833879 ) ) ;
#3343=( GEOMETRIC_REPRESENTATION_CONTEXT ( 3 ) GLOBAL_UNCERTAINTY_ASSIGNED_CONTEXT ( ( #9790 ) ) GLOBAL_UNIT_ASSIGNED_CONTEXT ( ( #9330, #7871, #18335 ) ) REPRESENTATION_CONTEXT ( 'NONE', 'WORKASPACE' ) );
#3348=CARTESIAN_POINT ( 'NONE',  ( 232.5999999999999375, -33.71249999999999147, -53.46410161513786363 ) ) ;
#3350=AXIS2_PLACEMENT_3D ( 'NONE', #13629, #10417, #11978 ) ;
#3356=CARTESIAN_POINT ( 'NONE',  ( 229.8435696437499303, -34.30312499938548143, -50.00000000000011369 ) ) ;
#3361=CARTESIAN_POINT ( 'NONE',  ( 233.9782151781249411, -34.49062499938548143, 102.3871387122750889 ) ) ;
#3366=CIRCLE ( 'NONE', #11792, 5.200000000000009948 ) ;
#3372=CARTESIAN_POINT ( 'NONE',  ( 235.3564303562499447, -31.67812499938547788, -51.59142580818350865 ) ) ;
#3379=VECTOR ( 'NONE', #5505, 1000.000000000000000 ) ;
#3383=CARTESIAN_POINT ( 'NONE',  ( 105.1999999999999886, -4.999999999999993783, -103.0000000000000995 ) ) ;
#3384=ORIENTED_EDGE ( 'NONE', *, *, #11545, .F. ) ;
#3389=CARTESIAN_POINT ( 'NONE',  ( 234.0999999999999375, -32.94374999877096144, -47.40192378864679768 ) ) ;
#3391=CARTESIAN_POINT ( 'NONE',  ( 235.3564303562499447, -33.66562499938548569, 101.5914258081833879 ) ) ;
#3402=CARTESIAN_POINT ( 'NONE',  ( 229.8435696437499587, -32.54062499938547859, -51.59142580818350154 ) ) ;
#3404=CARTESIAN_POINT ( 'NONE',  ( 235.3564303562499447, -31.37812499938547717, 99.99999999999998579 ) ) ;
#3405=CARTESIAN_POINT ( 'NONE',  ( 229.5999999999999375, -34.89374999877096428, -50.00000000000011369 ) ) ;
#3407=ORIENTED_EDGE ( 'NONE', *, *, #3262, .F. ) ;
#3413=VERTEX_POINT ( 'NONE', #1585 ) ;
#3420=CARTESIAN_POINT ( 'NONE',  ( 231.3931070460713499, -35.00000000000000000, 97.24646917567284277 ) ) ;
#3422=DIRECTION ( 'NONE',  ( 0.000000000000000000, 1.000000000000000000, 0.000000000000000000 ) ) ;
#3424=CARTESIAN_POINT ( 'NONE',  ( 229.8435696437499303, -35.09062499938547575, 99.99999999999998579 ) ) ;
#3425=CARTESIAN_POINT ( 'NONE',  ( 229.8435696437499871, -31.90312499938547575, 101.5914258081833879 ) ) ;
#3427=CARTESIAN_POINT ( 'NONE',  ( 231.0999999999999375, -31.66874999877096641, 102.5980762113533018 ) ) ;
#3434=CARTESIAN_POINT ( 'NONE',  ( 231.0999999999999375, -33.46874999877096002, 102.5980762113533018 ) ) ;
#3440=CARTESIAN_POINT ( 'NONE',  ( 232.5999999999999375, -29.99999999999999645, -50.00000000000011369 ) ) ;
#3449=CARTESIAN_POINT ( 'NONE',  ( 231.0999999999999375, -32.32499999999999574, -52.59807621135342970 ) ) ;
#3450=CARTESIAN_POINT ( 'NONE',  ( 229.8435696437499587, -32.91562499938547859, 101.5914258081833879 ) ) ;
#3452=CARTESIAN_POINT ( 'NONE',  ( 231.2217848218749339, -33.47812499938547859, -52.38713871227520968 ) ) ;
#3454=ORIENTED_EDGE ( 'NONE', *, *, #2503, .F. ) ;
#3464=CARTESIAN_POINT ( 'NONE',  ( 231.2217848218749339, -31.41562499938547859, -47.61286128772501769 ) ) ;
#3467=EDGE_CURVE ( 'NONE', #15949, #16690, #12639, .T. ) ;
#3470=CARTESIAN_POINT ( 'NONE',  ( 229.5999999999999375, -32.21249999999999858, 101.7320508075688821 ) ) ;
#3479=CARTESIAN_POINT ( 'NONE',  ( 229.8435696437499871, -30.17812499938547433, 98.40857419181659793 ) ) ;
#3481=EDGE_LOOP ( 'NONE', ( #16334, #11188, #3151, #9045 ) ) ;
#3489=EDGE_CURVE ( 'NONE', #4350, #7254, #1488, .T. ) ;
#3491=VERTEX_POINT ( 'NONE', #12415 ) ;
#3492=CARTESIAN_POINT ( 'NONE',  ( 235.3564303562499447, -34.94062499938547717, -51.59142580818350154 ) ) ;
#3494=CARTESIAN_POINT ( 'NONE',  ( 231.2217848218749339, -31.52812499938548285, 102.3871387122750889 ) ) ;
#3495=CARTESIAN_POINT ( 'NONE',  ( 235.3564303562499447, -31.37812499938547717, -50.00000000000011369 ) ) ;
#3501=CARTESIAN_POINT ( 'NONE',  ( 232.5999999999999375, -32.75624999877096144, -53.00000000000010658 ) ) ;
#3504=EDGE_LOOP ( 'NONE', ( #8592, #11763, #310, #18188 ) ) ;
#3514=EDGE_CURVE ( 'NONE', #5195, #12222, #6669, .T. ) ;
#3517=CARTESIAN_POINT ( 'NONE',  ( 233.9782151781249411, -34.04062499938547859, 102.3871387122750889 ) ) ;
#3518=EDGE_CURVE ( 'NONE', #3491, #12219, #10847, .T. ) ;
#3519=ORIENTED_EDGE ( 'NONE', *, *, #6542, .F. ) ;
#3521=CARTESIAN_POINT ( 'NONE',  ( 232.5999999999999091, -32.08124999877096428, 102.9999999999999858 ) ) ;
#3524=ORIENTED_EDGE ( 'NONE', *, *, #8413, .F. ) ;
#3527=PLANE ( 'NONE',  #11801 ) ;
#3535=ADVANCED_FACE ( 'NONE', ( #10849, #12604, #8116 ), #13973, .F. ) ;
#3546=CARTESIAN_POINT ( 'NONE',  ( 232.5999999999999375, -31.91249999999999432, -53.46410161513786363 ) ) ;
#3550=CARTESIAN_POINT ( 'NONE',  ( 235.3564303562499447, -32.69062499938547717, 98.40857419181659793 ) ) ;
#3552=CARTESIAN_POINT ( 'NONE',  ( 235.3564303562499447, -33.17812499938548143, -50.00000000000011369 ) ) ;
#3559=CARTESIAN_POINT ( 'NONE',  ( 235.5999999999999943, -34.68749999999999289, 98.26794919243110371 ) ) ;
#3564=CARTESIAN_POINT ( 'NONE',  ( 231.2217848218749339, -31.56562499938547717, -52.38713871227520968 ) ) ;
#3578=CARTESIAN_POINT ( 'NONE',  ( 232.5999999999999375, -33.06562499938547717, 96.81714838363319586 ) ) ;
#3592=CARTESIAN_POINT ( 'NONE',  ( 233.9782151781249411, -32.65312499938548285, 97.61286128772489690 ) ) ;
#3593=CARTESIAN_POINT ( 'NONE',  ( 235.3564303562499447, -31.82812499938547646, -50.00000000000011369 ) ) ;
#3596=EDGE_LOOP ( 'NONE', ( #12625, #3987, #13591 ) ) ;
#3611=CARTESIAN_POINT ( 'NONE',  ( 233.9825576637930169, -32.00000000000000000, 102.5835086888314294 ) ) ;
#3612=CARTESIAN_POINT ( 'NONE',  ( 233.9782151781249411, -34.49062499938548143, 102.3871387122750889 ) ) ;
#3616=DIRECTION ( 'NONE',  ( 1.000000000000000000, 0.000000000000000000, 0.000000000000000000 ) ) ;
#3624=CARTESIAN_POINT ( 'NONE',  ( 230.7186334667983658, -32.00000000000000711, 97.98546077809203325 ) ) ;
#3634=DIRECTION ( 'NONE',  ( -0.000000000000000000, -1.000000000000000000, -0.000000000000000000 ) ) ;
#3642=CARTESIAN_POINT ( 'NONE',  ( 229.5999999999999375, -34.46249999999999147, -48.26794919243123161 ) ) ;
#3646=FACE_OUTER_BOUND ( 'NONE', #16921, .T. ) ;
#3648=CARTESIAN_POINT ( 'NONE',  ( 235.3564303562499447, -32.69062499938547717, -51.59142580818350865 ) ) ;
#3653=CARTESIAN_POINT ( 'NONE',  ( 235.5999999999999943, -33.78750000000000142, -51.73205080756900287 ) ) ;
#3658=VECTOR ( 'NONE', #12966, 1000.000000000000000 ) ;
#3663=CARTESIAN_POINT ( 'NONE',  ( 232.5999999999999375, -32.05312499938548143, -53.18285161636690361 ) ) ;
#3668=VECTOR ( 'NONE', #5983, 1000.000000000000000 ) ;
#3676=( GEOMETRIC_REPRESENTATION_CONTEXT ( 3 ) GLOBAL_UNCERTAINTY_ASSIGNED_CONTEXT ( ( #15446 ) ) GLOBAL_UNIT_ASSIGNED_CONTEXT ( ( #7533, #12318, #3228 ) ) REPRESENTATION_CONTEXT ( 'NONE', 'WORKASPACE' ) );
#3678=CARTESIAN_POINT ( 'NONE',  ( 231.9572389284484757, -35.00000000000000000, -52.93757093704014949 ) ) ;
#3680=CARTESIAN_POINT ( 'NONE',  ( 232.5999999999999375, -32.05312499938548143, 96.81714838363319586 ) ) ;
#3683=CARTESIAN_POINT ( 'NONE',  ( 231.7961524227065979, -32.79240381056765585, 97.00000000000000000 ) ) ;
#3689=VECTOR ( 'NONE', #15560, 1000.000000000000000 ) ;
#3691=CARTESIAN_POINT ( 'NONE',  ( 235.3564303562499447, -34.97812499938547859, -50.00000000000011369 ) ) ;
#3692=CARTESIAN_POINT ( 'NONE',  ( 233.9782151781249411, -33.10312499938547859, 97.61286128772489690 ) ) ;
#3693=CARTESIAN_POINT ( 'NONE',  ( 235.3564303562499447, -34.11562499938548143, -48.40857419181671162 ) ) ;
#3698=FACE_OUTER_BOUND ( 'NONE', #3723, .T. ) ;
#3708=CARTESIAN_POINT ( 'NONE',  ( 231.9572389284484757, -35.00000000000000000, 97.06242906295996420 ) ) ;
#3710=CARTESIAN_POINT ( 'NONE',  ( 233.9782151781249411, -33.59062499938547575, 102.3871387122750889 ) ) ;
#3714=CARTESIAN_POINT ( 'NONE',  ( 232.5999999999999375, -31.40624999877096712, 96.53589838486223584 ) ) ;
#3715=CARTESIAN_POINT ( 'NONE',  ( 234.0999999999999375, -31.44374999877096144, -52.59807621135342970 ) ) ;
#3719=CARTESIAN_POINT ( 'NONE',  ( 244.7999999999999545, -29.80000000000003268, -103.0000000000000284 ) ) ;
#3720=ORIENTED_EDGE ( 'NONE', *, *, #14601, .F. ) ;
#3723=EDGE_LOOP ( 'NONE', ( #3194, #2426, #5492, #8499 ) ) ;
#3729=CARTESIAN_POINT ( 'NONE',  ( 232.5880334581522106, -34.99999999999999289, -52.99916460278299013 ) ) ;
#3730=CARTESIAN_POINT ( 'NONE',  ( 230.4884518427504076, -35.14114861271050216, 98.22820072003833047 ) ) ;
#3741=CARTESIAN_POINT ( 'NONE',  ( 231.2217848218749339, -34.82812499938548001, -52.38713871227520968 ) ) ;
#3748=CARTESIAN_POINT ( 'NONE',  ( 232.5999999999999943, -32.95312499938548001, -53.18285161636690361 ) ) ;
#3749=ADVANCED_FACE ( 'NONE', ( #18866 ), #6035, .F. ) ;
#3755=CARTESIAN_POINT ( 'NONE',  ( 229.8435696437499871, -33.70312499938548001, -48.40857419181671162 ) ) ;
#3758=ADVANCED_FACE ( 'NONE', ( #1542 ), #14618, .T. ) ;
#3761=CARTESIAN_POINT ( 'NONE',  ( 234.0999999999999375, -32.79374999877096286, 97.40192378864668399 ) ) ;
#3766=VERTEX_POINT ( 'NONE', #17660 ) ;
#3774=CARTESIAN_POINT ( 'NONE',  ( 230.0666556977843982, -31.99999999999997868, 101.1009827666099596 ) ) ;
#3783=CARTESIAN_POINT ( 'NONE',  ( 232.5999999999999375, -32.16562499938547859, 96.81714838363319586 ) ) ;
#3785=CARTESIAN_POINT ( 'NONE',  ( 235.3564303562499447, -33.59062499938548285, -51.59142580818350865 ) ) ;
#3788=VERTEX_POINT ( 'NONE', #4177 ) ;
#3799=VECTOR ( 'NONE', #3422, 1000.000000000000000 ) ;
#3801=CARTESIAN_POINT ( 'NONE',  ( 234.7546687845694180, -31.99999999999997868, 102.0417045141626176 ) ) ;
#3802=CARTESIAN_POINT ( 'NONE',  ( 233.9782151781249411, -32.99062499938548143, 97.61286128772489690 ) ) ;
#3808=CARTESIAN_POINT ( 'NONE',  ( 231.0999999999999375, -32.56874999877096144, 102.5980762113533018 ) ) ;
#3813=VECTOR ( 'NONE', #5408, 1000.000000000000000 ) ;
#3815=CARTESIAN_POINT ( 'NONE',  ( 234.0999999999999375, -33.69374999877096144, -52.59807621135342970 ) ) ;
#3822=CARTESIAN_POINT ( 'NONE',  ( 231.0999999999999375, -33.22499999999999432, 97.40192378864668399 ) ) ;
#3833=CARTESIAN_POINT ( 'NONE',  ( 233.9782151781249411, -34.90312499938547575, 97.61286128772489690 ) ) ;
#3835=CARTESIAN_POINT ( 'NONE',  ( 233.9782151781249411, -30.74062499938547788, -52.38713871227520968 ) ) ;
#3836=ORIENTED_EDGE ( 'NONE', *, *, #16768, .T. ) ;
#3840=AXIS2_PLACEMENT_3D ( 'NONE', #9295, #16725, #12138 ) ;
#3849=ADVANCED_FACE ( 'NONE', ( #4272 ), #16288, .F. ) ;
#3851=EDGE_CURVE ( 'NONE', #10258, #15900, #8532, .T. ) ;
#3853=CARTESIAN_POINT ( 'NONE',  ( 231.2217848218749339, -33.81562499938547717, -52.38713871227520968 ) ) ;
#3856=ORIENTED_EDGE ( 'NONE', *, *, #12684, .T. ) ;
#3864=ORIENTED_EDGE ( 'NONE', *, *, #6640, .T. ) ;
#3866=ADVANCED_FACE ( 'NONE', ( #3646 ), #17133, .F. ) ;
#3883=CARTESIAN_POINT ( 'NONE',  ( 232.5002178375173116, -35.00000000000000711, -47.23961338448017955 ) ) ;
#3884=CARTESIAN_POINT ( 'NONE',  ( 233.9782151781249411, -32.65312499938548285, -52.38713871227520968 ) ) ;
#3886=ORIENTED_EDGE ( 'NONE', *, *, #5074, .T. ) ;
#3899=CARTESIAN_POINT ( 'NONE',  ( 229.5999999999999375, -32.28749999999999432, -51.73205080756898866 ) ) ;
#3901=CARTESIAN_POINT ( 'NONE',  ( 232.5999999999999375, -30.33749999999999503, 103.4641016151377499 ) ) ;
#3902=ORIENTED_EDGE ( 'NONE', *, *, #12813, .F. ) ;
#3904=EDGE_CURVE ( 'NONE', #10663, #1022, #8022, .T. ) ;
#3905=CARTESIAN_POINT ( 'NONE',  ( 229.5999999999999375, -34.03124999877096002, 98.26794919243111792 ) ) ;
#3906=CARTESIAN_POINT ( 'NONE',  ( 232.5999999999999375, -30.95624999877096428, -53.46410161513786363 ) ) ;
#3907=VERTEX_POINT ( 'NONE', #4038 ) ;
#3913=VECTOR ( 'NONE', #16703, 1000.000000000000000 ) ;
#3916=( BOUNDED_CURVE ( )  B_SPLINE_CURVE ( 2, ( #2754, #824, #6783, #12731, #7246, #11740, #3133, #13399, #5786 ),
 .UNSPECIFIED., .F., .F. ) 
 B_SPLINE_CURVE_WITH_KNOTS ( ( 3, 2, 2, 2, 3 ),
 ( 0.5208333333333331483, 0.5277777777777777901, 0.5416666666666666297, 0.5555555555555555802, 0.5625000000000001110 ),
 .UNSPECIFIED. ) 
 CURVE ( )  GEOMETRIC_REPRESENTATION_ITEM ( )  RATIONAL_B_SPLINE_CURVE ( ( 0.9330127018922194093, 0.9330127018922177440, 1.000000000000000000, 0.8660254037844387076, 1.000000000000000000, 0.8660254037844387076, 1.000000000000000000, 0.9330127018922182991, 0.9330127018922194093 ) ) 
 REPRESENTATION_ITEM ( '' )  );
#3923=DIRECTION ( 'NONE',  ( 0.000000000000000000, 0.000000000000000000, 1.000000000000000000 ) ) ;
#3924=CARTESIAN_POINT ( 'NONE',  ( 229.5999999999999375, -32.19374999877096144, -50.00000000000011369 ) ) ;
#3931=CARTESIAN_POINT ( 'NONE',  ( 232.5999999999999375, -34.38749999999999574, -46.53589838486234953 ) ) ;
#3932=CARTESIAN_POINT ( 'NONE',  ( 233.2908335840015184, -34.99999999999998579, 97.11314983874018480 ) ) ;
#3934=CARTESIAN_POINT ( 'NONE',  ( 235.3564303562499447, -34.97812499938547859, 99.99999999999998579 ) ) ;
#3936=CARTESIAN_POINT ( 'NONE',  ( 231.2217848218749339, -34.67812499938548143, -47.61286128772501769 ) ) ;
#3938=CARTESIAN_POINT ( 'NONE',  ( 232.5999999999999659, -32.13749999999999574, -47.00000000000011369 ) ) ;
#3944=LINE ( 'NONE', #1026, #17424 ) ;
#3945=CARTESIAN_POINT ( 'NONE',  ( 231.2217848218749339, -32.01562499938548001, -52.38713871227520968 ) ) ;
#3952=CARTESIAN_POINT ( 'NONE',  ( 235.3564303562499447, -32.20312499938548001, -48.40857419181671162 ) ) ;
#3961=DIRECTION ( 'NONE',  ( 1.000000000000000000, -5.139921410301648824E-16, 1.621047990368529987E-30 ) ) ;
#3963=CARTESIAN_POINT ( 'NONE',  ( 229.8435696437499587, -33.32812499938548001, 98.40857419181659793 ) ) ;
#3971=CARTESIAN_POINT ( 'NONE',  ( 232.5999999999999375, -29.99999999999999645, -47.00000000000010658 ) ) ;
#3972=CARTESIAN_POINT ( 'NONE',  ( 234.7581833435467047, -32.00000000000000000, 97.97695283456471316 ) ) ;
#3977=ADVANCED_FACE ( 'NONE', ( #2370 ), #8331, .T. ) ;
#3981=CARTESIAN_POINT ( 'NONE',  ( 235.0940413310670465, -34.99999999999998579, -48.81289630734742246 ) ) ;
#3982=CARTESIAN_POINT ( 'NONE',  ( 229.8435696437499303, -32.50312499938547717, -50.00000000000011369 ) ) ;
#3983=CIRCLE ( 'NONE', #565, 2.200000000000007283 ) ;
#3984=( BOUNDED_CURVE ( )  B_SPLINE_CURVE ( 2, ( #14323, #4171, #9743, #14414, #7101 ),
 .UNSPECIFIED., .F., .F. ) 
 B_SPLINE_CURVE_WITH_KNOTS ( ( 3, 2, 3 ),
 ( 0.2975293541897499061, 0.3055555555555555802, 0.3125000000000000555 ),
 .UNSPECIFIED. ) 
 CURVE ( )  GEOMETRIC_REPRESENTATION_ITEM ( )  RATIONAL_B_SPLINE_CURVE ( ( 0.9346381638529874802, 0.9225778897267407075, 1.000000000000000000, 0.9330127018922187432, 0.9330127018922192983 ) ) 
 REPRESENTATION_ITEM ( '' )  );
#3987=ORIENTED_EDGE ( 'NONE', *, *, #9704, .T. ) ;
#3993=AXIS2_PLACEMENT_3D ( 'NONE', #17952, #10421, #11693 ) ;
#4002=FACE_OUTER_BOUND ( 'NONE', #16942, .T. ) ;
#4004=CARTESIAN_POINT ( 'NONE',  ( 232.5999999999999375, -30.78749999999999432, 103.4641016151377499 ) ) ;
#4010=CARTESIAN_POINT ( 'NONE',  ( 232.5999999999999375, -32.30624999877095860, 96.53589838486223584 ) ) ;
#4011=CARTESIAN_POINT ( 'NONE',  ( 235.5999999999999943, -31.03124999877096357, -51.73205080756900287 ) ) ;
#4012=ADVANCED_FACE ( 'NONE', ( #16245 ), #1681, .T. ) ;
#4016=EDGE_LOOP ( 'NONE', ( #8880, #9781, #1377, #1515 ) ) ;
#4030=CARTESIAN_POINT ( 'NONE',  ( 232.5999999999999375, -33.65624999877096002, -53.00000000000011369 ) ) ;
#4034=CARTESIAN_POINT ( 'NONE',  ( 231.0999999999999375, -34.87499999999999289, -47.40192378864679768 ) ) ;
#4035=CARTESIAN_POINT ( 'NONE',  ( 235.3288510558096505, -35.00000000000001421, 99.22311565912356457 ) ) ;
#4038=CARTESIAN_POINT ( 'NONE',  ( 249.9999999999999716, -5.000000000000004441, -100.0000000000000000 ) ) ;
#4041=CARTESIAN_POINT ( 'NONE',  ( 233.9782151781249411, -35.05312499938548143, -47.61286128772501769 ) ) ;
#4047=CARTESIAN_POINT ( 'NONE',  ( 235.3564303562499447, -30.36562499938547788, 99.99999999999998579 ) ) ;
#4048=CARTESIAN_POINT ( 'NONE',  ( 229.8435696437499303, -32.84062499938547575, -50.00000000000011369 ) ) ;
#4053=CARTESIAN_POINT ( 'NONE',  ( 233.9782151781249411, -33.14062499938548001, -47.61286128772501769 ) ) ;
#4057=DIRECTION ( 'NONE',  ( 0.000000000000000000, 0.000000000000000000, -1.000000000000000000 ) ) ;
#4062=EDGE_LOOP ( 'NONE', ( #14614, #10676, #16220, #18509 ) ) ;
#4063=CARTESIAN_POINT ( 'NONE',  ( 232.5999999999999091, -32.08124999877096428, 102.9999999999999858 ) ) ;
#4066=CARTESIAN_POINT ( 'NONE',  ( 233.9782151781249411, -33.59062499938547575, 102.3871387122750889 ) ) ;
#4067=LINE ( 'NONE', #7186, #12652 ) ;
#4077=ORIENTED_EDGE ( 'NONE', *, *, #1230, .T. ) ;
#4079=CARTESIAN_POINT ( 'NONE',  ( 232.5999999999999375, -34.64062499938548001, 103.1828516163667899 ) ) ;
#4080=CARTESIAN_POINT ( 'NONE',  ( 229.8435696437499303, -32.95312499938548001, -50.00000000000011369 ) ) ;
#4095=CARTESIAN_POINT ( 'NONE',  ( 232.5002178375172832, -34.99999999999998579, 102.7603866155199199 ) ) ;
#4097=CARTESIAN_POINT ( 'NONE',  ( 229.5999999999999375, -30.86249999999999361, 101.7320508075688679 ) ) ;
#4098=( BOUNDED_CURVE ( )  B_SPLINE_CURVE ( 2, ( #13861, #503, #16906, #16812, #6456, #18669, #15336, #14063, #2153 ),
 .UNSPECIFIED., .F., .F. ) 
 B_SPLINE_CURVE_WITH_KNOTS ( ( 3, 2, 2, 2, 3 ),
 ( 0.3541666666666666852, 0.3611111111111111049, 0.3750000000000000000, 0.3888888888888888951, 0.3958333333333333703 ),
 .UNSPECIFIED. ) 
 CURVE ( )  GEOMETRIC_REPRESENTATION_ITEM ( )  RATIONAL_B_SPLINE_CURVE ( ( 0.9330127018922194093, 0.9330127018922196314, 1.000000000000000000, 0.8660254037844387076, 1.000000000000000000, 0.8660254037844387076, 1.000000000000000000, 0.9330127018922190762, 0.9330127018922194093 ) ) 
 REPRESENTATION_ITEM ( '' )  );
#4099=EDGE_CURVE ( 'NONE', #18958, #8738, #3135, .T. ) ;
#4101=CARTESIAN_POINT ( 'NONE',  ( 229.8435696437499587, -32.02817623523064583, -48.94122380911299075 ) ) ;
#4103=CARTESIAN_POINT ( 'NONE',  ( 231.0999999999999375, -33.46874999877096002, 102.5980762113533018 ) ) ;
#4104=CARTESIAN_POINT ( 'NONE',  ( 235.5999999999999943, -30.58124999877096073, -51.73205080756900287 ) ) ;
#4110=CARTESIAN_POINT ( 'NONE',  ( 234.0999999999999375, -34.35000000000000142, -47.40192378864679768 ) ) ;
#4112=DIRECTION ( 'NONE',  ( -1.000000000000000000, 0.000000000000000000, 0.000000000000000000 ) ) ;
#4115=EDGE_CURVE ( 'NONE', #14649, #4852, #227, .T. ) ;
#4119=EDGE_CURVE ( 'NONE', #6709, #531, #12017, .T. ) ;
#4120=CARTESIAN_POINT ( 'NONE',  ( 231.0999999999999375, -32.26874999877096428, -52.59807621135342970 ) ) ;
#4130=CARTESIAN_POINT ( 'NONE',  ( 232.5999999999999375, -29.99999999999999645, 103.0000000000000000 ) ) ;
#4131=CARTESIAN_POINT ( 'NONE',  ( 229.8435696437499587, -33.81562499938547717, 101.5914258081833879 ) ) ;
#4134=CARTESIAN_POINT ( 'NONE',  ( 232.5999999999999375, -31.15312499938547930, -53.18285161636690361 ) ) ;
#4135=ORIENTED_EDGE ( 'NONE', *, *, #3489, .F. ) ;
#4140=CARTESIAN_POINT ( 'NONE',  ( 233.9782151781249411, -32.24062499938548143, 102.3871387122750889 ) ) ;
#4149=CARTESIAN_POINT ( 'NONE',  ( 229.5999999999999375, -30.89999999999999858, -50.00000000000011369 ) ) ;
#4163=CARTESIAN_POINT ( 'NONE',  ( 235.3564303562499447, -33.51562499938548001, 99.99999999999998579 ) ) ;
#4164=DIRECTION ( 'NONE',  ( 0.000000000000000000, -1.000000000000000000, 0.000000000000000000 ) ) ;
#4168=CARTESIAN_POINT ( 'NONE',  ( 234.0999999999999375, -32.84999999999999432, 97.40192378864668399 ) ) ;
#4169=FACE_BOUND ( 'NONE', #10381, .T. ) ;
#4171=CARTESIAN_POINT ( 'NONE',  ( 234.9136945297046850, -32.02340763552835767, 102.1282894555902061 ) ) ;
#4176=CARTESIAN_POINT ( 'NONE',  ( 232.5999999999999375, -34.41562499938547859, 96.81714838363319586 ) ) ;
#4177=CARTESIAN_POINT ( 'NONE',  ( 244.7999999999999545, -29.80000000000002203, 150.0000000000000000 ) ) ;
#4182=DIRECTION ( 'NONE',  ( 0.000000000000000000, -1.000000000000000000, 0.000000000000000000 ) ) ;
#4191=CARTESIAN_POINT ( 'NONE',  ( 231.7960411235079050, -35.00000000000002132, 102.6365808225362883 ) ) ;
#4193=CARTESIAN_POINT ( 'NONE',  ( 229.5999999999999375, -31.31249999999998934, 101.7320508075688679 ) ) ;
#4197=CARTESIAN_POINT ( 'NONE',  ( 234.0999999999999375, -32.79374999877096286, 97.40192378864668399 ) ) ;
#4198=CARTESIAN_POINT ( 'NONE',  ( 235.5999999999999943, -32.90624999877096002, -48.26794919243124582 ) ) ;
#4204=CARTESIAN_POINT ( 'NONE',  ( 235.5999999999999375, -34.27499999999999147, -50.00000000000011369 ) ) ;
#4209=ADVANCED_FACE ( 'NONE', ( #13783 ), #9683, .F. ) ;
#4213=CARTESIAN_POINT ( 'NONE',  ( 235.5999999999999943, -32.38124999877096144, -51.73205080756900287 ) ) ;
#4218=CARTESIAN_POINT ( 'NONE',  ( 231.7960411235079050, -35.00000000000002132, 102.6365808225362883 ) ) ;
#4223=AXIS2_PLACEMENT_3D ( 'NONE', #7397, #14526, #11890 ) ;
#4226=CARTESIAN_POINT ( 'NONE',  ( 235.3564303562499447, -34.49062499938548143, 98.40857419181659793 ) ) ;
#4229=CARTESIAN_POINT ( 'NONE',  ( 229.8435696437499871, -33.70312499938548001, -48.40857419181671162 ) ) ;
#4231=ORIENTED_EDGE ( 'NONE', *, *, #11858, .T. ) ;
#4234=EDGE_CURVE ( 'NONE', #16126, #13209, #9581, .T. ) ;
#4238=CARTESIAN_POINT ( 'NONE',  ( 231.2217848218749339, -30.96562499938547930, 102.3871387122750889 ) ) ;
#4239=AXIS2_PLACEMENT_3D ( 'NONE', #5354, #10317, #5826 ) ;
#4240=CARTESIAN_POINT ( 'NONE',  ( 244.7999999999999545, -32.00000000000000000, -97.80000000000002558 ) ) ;
#4245=CARTESIAN_POINT ( 'NONE',  ( 233.9782151781249411, -34.34062499938547575, -52.38713871227520968 ) ) ;
#4256=CARTESIAN_POINT ( 'NONE',  ( 232.5999999999999375, -29.99999999999999645, 99.99999999999998579 ) ) ;
#4271=CARTESIAN_POINT ( 'NONE',  ( 231.7960411235079050, -35.00000000000002132, -47.36341917746382535 ) ) ;
#4272=FACE_OUTER_BOUND ( 'NONE', #6582, .T. ) ;
#4273=CARTESIAN_POINT ( 'NONE',  ( 232.5999999999999375, -34.33124999877097139, 102.9999999999999858 ) ) ;
#4274=CARTESIAN_POINT ( 'NONE',  ( 232.5999999999999375, -29.99999999999999645, 96.99999999999998579 ) ) ;
#4277=AXIS2_PLACEMENT_3D ( 'NONE', #16017, #9966, #11329 ) ;
#4282=CARTESIAN_POINT ( 'NONE',  ( 231.0999999999999375, -34.42499999999999716, -47.40192378864679768 ) ) ;
#4284=CARTESIAN_POINT ( 'NONE',  ( 235.3564303562499447, -31.41562499938548214, 101.5914258081833879 ) ) ;
#4286=AXIS2_PLACEMENT_3D ( 'NONE', #15644, #12993, #14355 ) ;
#4289=DIRECTION ( 'NONE',  ( 1.000000000000000000, 0.000000000000000000, 0.000000000000000000 ) ) ;
#4290=CARTESIAN_POINT ( 'NONE',  ( 232.5999999999999375, -32.36249999999999716, -53.00000000000011369 ) ) ;
#4293=CARTESIAN_POINT ( 'NONE',  ( 232.5999999999999375, -33.93750000000000000, 103.4641016151377499 ) ) ;
#4296=CARTESIAN_POINT ( 'NONE',  ( 229.5999999999999375, -33.50624999877096144, 101.7320508075688679 ) ) ;
#4297=CARTESIAN_POINT ( 'NONE',  ( 232.5999999999999375, -34.33124999877096428, -46.53589838486234953 ) ) ;
#4302=PLANE ( 'NONE',  #5412 ) ;
#4309=AXIS2_PLACEMENT_3D ( 'NONE', #8868, #14826, #11810 ) ;
#4324=CARTESIAN_POINT ( 'NONE',  ( 234.0999999999999375, -34.74374999877096570, -47.40192378864679768 ) ) ;
#4328=CARTESIAN_POINT ( 'NONE',  ( 235.3564303562499447, -34.00312499938547717, -48.40857419181671162 ) ) ;
#4335=CARTESIAN_POINT ( 'NONE',  ( 232.5999999999999375, -33.20624999877097139, -53.00000000000011369 ) ) ;
#4336=CARTESIAN_POINT ( 'NONE',  ( 232.5999999999999375, -31.82812499938547290, 103.1828516163667899 ) ) ;
#4337=CARTESIAN_POINT ( 'NONE',  ( 235.3564303562499447, -34.45312499938548001, -48.40857419181671162 ) ) ;
#4341=CARTESIAN_POINT ( 'NONE',  ( 235.3564303562499447, -34.45312499938548001, -48.40857419181671162 ) ) ;
#4348=CARTESIAN_POINT ( 'NONE',  ( 232.5999999999999375, -30.36562499938548498, -53.18285161636690361 ) ) ;
#4350=VERTEX_POINT ( 'NONE', #2163 ) ;
#4351=CARTESIAN_POINT ( 'NONE',  ( 233.9782151781249411, -32.54062499938547859, 97.61286128772489690 ) ) ;
#4363=CARTESIAN_POINT ( 'NONE',  ( 231.6794753800827777, -34.98323688327302960, 97.06736352196708140 ) ) ;
#4368=CARTESIAN_POINT ( 'NONE',  ( 232.5999999999999375, -29.99999999999999645, 99.99999999999998579 ) ) ;
#4369=CARTESIAN_POINT ( 'NONE',  ( 229.8435696437499871, -35.16562499938547148, -48.40857419181671162 ) ) ;
#4371=CYLINDRICAL_SURFACE ( 'NONE', #3993, 2.200000000000007283 ) ;
#4381=CARTESIAN_POINT ( 'NONE',  ( 232.5999999999999375, -31.71562499938547930, 96.81714838363319586 ) ) ;
#4387=ADVANCED_FACE ( 'NONE', ( #512 ), #3527, .F. ) ;
#4389=CARTESIAN_POINT ( 'NONE',  ( 229.5999999999999375, -32.69999999999999574, 99.99999999999998579 ) ) ;
#4391=CARTESIAN_POINT ( 'NONE',  ( 232.5999999999999375, -34.78124999877096002, 102.9999999999999858 ) ) ;
#4392=CARTESIAN_POINT ( 'NONE',  ( 234.0999999999999375, -34.29374999877096286, 102.5980762113533018 ) ) ;
#4393=CARTESIAN_POINT ( 'NONE',  ( 229.5999999999999375, -34.03124999877096002, -51.73205080756898866 ) ) ;
#4402=ORIENTED_EDGE ( 'NONE', *, *, #11313, .T. ) ;
#4404=CARTESIAN_POINT ( 'NONE',  ( 232.5999999999999091, -34.10624999877096286, 96.99999999999998579 ) ) ;
#4411=FACE_OUTER_BOUND ( 'NONE', #14793, .T. ) ;
#4417=CARTESIAN_POINT ( 'NONE',  ( 232.5999999999999375, -29.99999999999999645, 103.0000000000000000 ) ) ;
#4420=CARTESIAN_POINT ( 'NONE',  ( 232.5999999999999375, -33.40312499938547575, -53.18285161636690361 ) ) ;
#4421=ORIENTED_EDGE ( 'NONE', *, *, #15209, .T. ) ;
#4423=CARTESIAN_POINT ( 'NONE',  ( 102.9999999999999858, -29.80000000000000071, -100.0000000000000000 ) ) ;
#4428=CARTESIAN_POINT ( 'NONE',  ( 232.5999999999999375, -34.07812499938548001, 103.1828516163667899 ) ) ;
#4431=AXIS2_PLACEMENT_3D ( 'NONE', #4796, #15234, #8197 ) ;
#4435=CARTESIAN_POINT ( 'NONE',  ( 229.8435696437499303, -35.09062499938547575, -50.00000000000011369 ) ) ;
#4440=CARTESIAN_POINT ( 'NONE',  ( 235.5999999999999375, -32.86874999877096570, 99.99999999999998579 ) ) ;
#4441=CARTESIAN_POINT ( 'NONE',  ( 235.3564303562499447, -31.79062499938547859, -51.59142580818350865 ) ) ;
#4451=EDGE_CURVE ( 'NONE', #3788, #15137, #5077, .T. ) ;
#4463=PLANE ( 'NONE',  #3350 ) ;
#4472=CARTESIAN_POINT ( 'NONE',  ( 229.5999999999999375, -33.63749999999999574, -51.73205080756898866 ) ) ;
#4476=CARTESIAN_POINT ( 'NONE',  ( 235.3564303562499447, -31.82812499938547646, 99.99999999999998579 ) ) ;
#4484=CARTESIAN_POINT ( 'NONE',  ( 231.0999999999999375, -33.07499999999999574, 102.5980762113533018 ) ) ;
#4485=ORIENTED_EDGE ( 'NONE', *, *, #1639, .T. ) ;
#4486=CARTESIAN_POINT ( 'NONE',  ( 229.8435696437499303, -33.40312499938547575, -50.00000000000011369 ) ) ;
#4488=CARTESIAN_POINT ( 'NONE',  ( 232.5999999999999375, -35.00624999877096855, 96.53589838486223584 ) ) ;
#4489=CARTESIAN_POINT ( 'NONE',  ( 232.5999999999999375, -32.53124999877096002, -46.53589838486234953 ) ) ;
#4499=SHAPE_REPRESENTATION ( 'tray', ( #10540 ), #13638 ) ;
#4503=DIRECTION ( 'NONE',  ( -0.000000000000000000, 1.000000000000000000, -0.000000000000000000 ) ) ;
#4514=CARTESIAN_POINT ( 'NONE',  ( 232.5999999999999375, -32.27812499938547575, -46.81714838363331666 ) ) ;
#4524=CARTESIAN_POINT ( 'NONE',  ( 229.8435696437499871, -34.22812499938547148, 98.40857419181659793 ) ) ;
#4525=B_SPLINE_CURVE_WITH_KNOTS ( 'NONE', 3,
 ( #18197, #333, #6281, #15061, #228, #3232, #13784, #12134, #10660, #513, #15256, #9192, #13691, #18389, #5009, #12225, #426, #1590 ),
 .UNSPECIFIED., .F., .F.,
 ( 4, 2, 2, 2, 2, 2, 2, 2, 4 ),
 ( 0.000000000000000000, 0.0007089252359836048425, 0.001417850471967209685, 0.002126775707950814311, 0.002835700943934419370, 0.003544626179918024429, 0.004253551415901628621, 0.004962476651885233681, 0.005671401887868838740 ),
 .UNSPECIFIED. ) ;
#4526=CARTESIAN_POINT ( 'NONE',  ( 235.3564303562499447, -33.47812499938547859, -51.59142580818350154 ) ) ;
#4530=ORIENTED_EDGE ( 'NONE', *, *, #8590, .T. ) ;
#4531=CARTESIAN_POINT ( 'NONE',  ( 234.0999999999999375, -30.74999999999999645, -47.40192378864679768 ) ) ;
#4535=DIRECTION ( 'NONE',  ( -1.000000000000000000, 0.000000000000000000, 0.000000000000000000 ) ) ;
#4536=CARTESIAN_POINT ( 'NONE',  ( 231.2217848218749339, -31.07812499938548001, -47.61286128772501769 ) ) ;
#4539=DIRECTION ( 'NONE',  ( -0.000000000000000000, -1.000000000000000000, -0.000000000000000000 ) ) ;
#4540=EDGE_CURVE ( 'NONE', #9588, #10258, #7399, .T. ) ;
#4543=CARTESIAN_POINT ( 'NONE',  ( 233.9782151781249411, -33.89062499938548001, 97.61286128772489690 ) ) ;
#4556=VERTEX_POINT ( 'NONE', #5167 ) ;
#4558=FACE_OUTER_BOUND ( 'NONE', #7055, .T. ) ;
#4562=CYLINDRICAL_SURFACE ( 'NONE', #7744, 3.000000000000009770 ) ;
#4568=VECTOR ( 'NONE', #14819, 1000.000000000000000 ) ;
#4570=CARTESIAN_POINT ( 'NONE',  ( 233.9782151781249411, -32.20312499938548001, 97.61286128772489690 ) ) ;
#4575=DIRECTION ( 'NONE',  ( 0.000000000000000000, 0.000000000000000000, 1.000000000000000000 ) ) ;
#4581=CARTESIAN_POINT ( 'NONE',  ( 235.5999999999999943, -34.68749999999999289, 98.26794919243110371 ) ) ;
#4582=ORIENTED_EDGE ( 'NONE', *, *, #15340, .T. ) ;
#4583=CARTESIAN_POINT ( 'NONE',  ( 232.5999999999999943, -33.29062499938547859, -46.81714838363331666 ) ) ;
#4585=CARTESIAN_POINT ( 'NONE',  ( 231.2217848218749339, -31.07812499938548001, 102.3871387122750889 ) ) ;
#4586=CARTESIAN_POINT ( 'NONE',  ( 232.5999999999999375, -33.65624999877096002, -53.46410161513786363 ) ) ;
#4587=VECTOR ( 'NONE', #16475, 1000.000000000000000 ) ;
#4588=ADVANCED_FACE ( 'NONE', ( #8469 ), #11316, .F. ) ;
#4591=ORIENTED_EDGE ( 'NONE', *, *, #15939, .T. ) ;
#4598=CARTESIAN_POINT ( 'NONE',  ( 235.5999999999999943, -32.43749999999999289, 98.26794919243110371 ) ) ;
#4601=EDGE_CURVE ( 'NONE', #16690, #10239, #10767, .T. ) ;
#4607=DIRECTION ( 'NONE',  ( 0.000000000000000000, 0.000000000000000000, -1.000000000000000000 ) ) ;
#4609=CARTESIAN_POINT ( 'NONE',  ( 235.3564303562499447, -31.30312499938547788, 101.5914258081833879 ) ) ;
#4614=CARTESIAN_POINT ( 'NONE',  ( 234.0999999999999375, -33.74999999999999289, 97.40192378864668399 ) ) ;
#4618=CARTESIAN_POINT ( 'NONE',  ( 231.2217848218749339, -35.01562499938548001, -47.61286128772501769 ) ) ;
#4620=( BOUNDED_CURVE ( )  B_SPLINE_CURVE ( 2, ( #8684, #5758, #14535, #8778, #13079, #3899, #5383, #2438, #4290 ),
 .UNSPECIFIED., .F., .F. ) 
 B_SPLINE_CURVE_WITH_KNOTS ( ( 3, 2, 2, 2, 3 ),
 ( 0.3958333333333333148, 0.4027777777777777901, 0.4166666666666666852, 0.4305555555555555802, 0.4374999999999999445 ),
 .UNSPECIFIED. ) 
 CURVE ( )  GEOMETRIC_REPRESENTATION_ITEM ( )  RATIONAL_B_SPLINE_CURVE ( ( 0.9330127018922194093, 0.9330127018922190762, 1.000000000000000000, 0.8660254037844387076, 1.000000000000000000, 0.8660254037844387076, 1.000000000000000000, 0.9330127018922198534, 0.9330127018922192983 ) ) 
 REPRESENTATION_ITEM ( '' )  );
#4622=ORIENTED_EDGE ( 'NONE', *, *, #15566, .F. ) ;
#4630=CARTESIAN_POINT ( 'NONE',  ( 232.5999999999999375, -33.62812499938547717, 103.1828516163667899 ) ) ;
#4631=CARTESIAN_POINT ( 'NONE',  ( 233.9782151781249411, -33.14062499938548001, -47.61286128772501769 ) ) ;
#4638=CARTESIAN_POINT ( 'NONE',  ( 234.0999999999999375, -33.29999999999999716, -52.59807621135342970 ) ) ;
#4643=CARTESIAN_POINT ( 'NONE',  ( 105.1999999999999744, -29.80000000000000071, -100.0000000000000000 ) ) ;
#4644=CARTESIAN_POINT ( 'NONE',  ( 229.8435696437499871, -31.19062499938548072, -51.59142580818350865 ) ) ;
#4649=CARTESIAN_POINT ( 'NONE',  ( 232.5999999999999943, -34.52812499938547575, 103.1828516163667899 ) ) ;
#4654=CARTESIAN_POINT ( 'NONE',  ( 235.4117376914898045, -31.99999999999999289, 98.95399275611721635 ) ) ;
#4657=CARTESIAN_POINT ( 'NONE',  ( 232.5999999999999375, -34.78124999877096002, 102.9999999999999858 ) ) ;
#4663=CARTESIAN_POINT ( 'NONE',  ( 244.7999999999999545, -4.999999999999990230, -100.0000000000000995 ) ) ;
#4672=CARTESIAN_POINT ( 'NONE',  ( 232.5999999999999375, -29.99999999999999645, 99.99999999999998579 ) ) ;
#4673=CARTESIAN_POINT ( 'NONE',  ( 232.5999999999999375, -31.04062499938547859, 103.1828516163667899 ) ) ;
#4678=FACE_OUTER_BOUND ( 'NONE', #15835, .T. ) ;
#4681=CARTESIAN_POINT ( 'NONE',  ( 232.5999999999999375, -32.58749999999999858, 103.4641016151377499 ) ) ;
#4683=CARTESIAN_POINT ( 'NONE',  ( 233.9782151781249411, -33.55312499938548143, -52.38713871227520968 ) ) ;
#4684=CARTESIAN_POINT ( 'NONE',  ( 232.5999999999999375, -30.59062499938547930, 103.1828516163667899 ) ) ;
#4685=CARTESIAN_POINT ( 'NONE',  ( 235.3564303562499447, -31.34062499938548285, -51.59142580818350865 ) ) ;
#4689=CARTESIAN_POINT ( 'NONE',  ( 232.5999999999999091, -34.38749999999999574, -47.00000000000011369 ) ) ;
#4691=LINE ( 'NONE', #18270, #14102 ) ;
#4694=CARTESIAN_POINT ( 'NONE',  ( 229.5999999999999375, -33.95624999877096428, 101.7320508075688821 ) ) ;
#4698=( BOUNDED_CURVE ( )  B_SPLINE_CURVE ( 2, ( #4654, #362, #15095, #7381, #16279, #13341, #18132 ),
 .UNSPECIFIED., .F., .F. ) 
 B_SPLINE_CURVE_WITH_KNOTS ( ( 3, 2, 2, 3 ),
 ( 0.3702305174531553833, 0.3750000000000000000, 0.3888888888888888951, 0.3958333333333333148 ),
 .UNSPECIFIED. ) 
 CURVE ( )  GEOMETRIC_REPRESENTATION_ITEM ( )  RATIONAL_B_SPLINE_CURVE ( ( 0.9395835397632974484, 0.9539927561173113801, 1.000000000000000000, 0.8660254037844387076, 1.000000000000000000, 0.9330127018922196314, 0.9330127018922194093 ) ) 
 REPRESENTATION_ITEM ( '' )  );
#4703=CARTESIAN_POINT ( 'NONE',  ( 232.5999999999999375, -32.30624999877096570, -53.00000000000011369 ) ) ;
#4704=CARTESIAN_POINT ( 'NONE',  ( 235.5999999999999375, -33.37499999999999289, 99.99999999999998579 ) ) ;
#4707=CARTESIAN_POINT ( 'NONE',  ( 235.3564303562499447, -31.22812499938548214, 98.40857419181659793 ) ) ;
#4708=ORIENTED_EDGE ( 'NONE', *, *, #7742, .F. ) ;
#4709=APPLICATION_CONTEXT ( 'automotive_design' ) ;
#4713=PLANE ( 'NONE',  #11139 ) ;
#4716=CARTESIAN_POINT ( 'NONE',  ( 235.3564303562499447, -34.82812499938548001, -51.59142580818350865 ) ) ;
#4717=ORIENTED_EDGE ( 'NONE', *, *, #6180, .T. ) ;
#4722=ADVANCED_FACE ( 'NONE', ( #11984 ), #4371, .F. ) ;
#4727=CARTESIAN_POINT ( 'NONE',  ( 229.8435696437499303, -32.84062499938547575, 99.99999999999998579 ) ) ;
#4732=CARTESIAN_POINT ( 'NONE',  ( 235.5999999999999943, -33.41250000000000142, -48.26794919243124582 ) ) ;
#4739=CARTESIAN_POINT ( 'NONE',  ( 229.8435696437499871, -32.99062499938548143, -51.59142580818350865 ) ) ;
#4741=ORIENTED_EDGE ( 'NONE', *, *, #4115, .F. ) ;
#4743=CARTESIAN_POINT ( 'NONE',  ( 235.3564303562499447, -33.92812499938548143, 98.40857419181659793 ) ) ;
#4744=ADVANCED_FACE ( 'NONE', ( #1634 ), #4562, .F. ) ;
#4747=EDGE_CURVE ( 'NONE', #531, #19282, #13155, .T. ) ;
#4748=AXIS2_PLACEMENT_3D ( 'NONE', #12398, #9461, #18368 ) ;
#4756=CARTESIAN_POINT ( 'NONE',  ( 235.3564303562499447, -31.75312499938547717, -48.40857419181671162 ) ) ;
#4773=CARTESIAN_POINT ( 'NONE',  ( 235.5999999999999375, -32.86874999877096570, -50.00000000000011369 ) ) ;
#4774=CARTESIAN_POINT ( 'NONE',  ( 229.8435696437499871, -33.81562499938547717, 101.5914258081833879 ) ) ;
#4777=CARTESIAN_POINT ( 'NONE',  ( 231.7961524227065979, -32.60759618943232852, 103.0000000000000000 ) ) ;
#4780=AXIS2_PLACEMENT_3D ( 'NONE', #1995, #6593, #2191 ) ;
#4786=CARTESIAN_POINT ( 'NONE',  ( 235.3564303562499447, -33.21562499938548285, -48.40857419181671162 ) ) ;
#4788=CARTESIAN_POINT ( 'NONE',  ( 235.5999999999999375, -34.66874999877096286, 99.99999999999998579 ) ) ;
#4789=CARTESIAN_POINT ( 'NONE',  ( 235.3564303562499447, -30.47812499938547859, -50.00000000000011369 ) ) ;
#4792=VERTEX_POINT ( 'NONE', #10330 ) ;
#4795=( BOUNDED_CURVE ( )  B_SPLINE_CURVE ( 2, ( #9172, #18172, #3116, #13566, #10268, #1379, #13669 ),
 .UNSPECIFIED., .F., .F. ) 
 B_SPLINE_CURVE_WITH_KNOTS ( ( 3, 2, 2, 3 ),
 ( 0.8958333333333332593, 0.9027777777777777901, 0.9166666666666666297, 0.9258785066912882389 ),
 .UNSPECIFIED. ) 
 CURVE ( )  GEOMETRIC_REPRESENTATION_ITEM ( )  RATIONAL_B_SPLINE_CURVE ( ( 0.9330127018922192983, 0.9330127018922187432, 1.000000000000000000, 0.8660254037844387076, 1.000000000000000000, 0.9111410165655264848, 0.9401539157124900736 ) ) 
 REPRESENTATION_ITEM ( '' )  );
#4796=CARTESIAN_POINT ( 'NONE',  ( 105.1999999999999744, -29.80000000000000071, -100.0000000000000000 ) ) ;
#4799=LINE ( 'NONE', #10739, #3913 ) ;
#4809=CARTESIAN_POINT ( 'NONE',  ( 233.9782151781249411, -32.54062499938547859, 97.61286128772489690 ) ) ;
#4813=ORIENTED_EDGE ( 'NONE', *, *, #13211, .F. ) ;
#4826=CARTESIAN_POINT ( 'NONE',  ( 235.3564303562499447, -34.45312499938548001, 101.5914258081833879 ) ) ;
#4830=EDGE_CURVE ( 'NONE', #11119, #5593, #6902, .T. ) ;
#4833=CARTESIAN_POINT ( 'NONE',  ( 235.5999999999999943, -31.53749999999999432, -51.73205080756900287 ) ) ;
#4837=CARTESIAN_POINT ( 'NONE',  ( 229.8435696437499871, -34.26562499938548001, -48.40857419181671162 ) ) ;
#4842=CARTESIAN_POINT ( 'NONE',  ( 233.9782151781249411, -34.04062499938547859, 102.3871387122750889 ) ) ;
#4845=CARTESIAN_POINT ( 'NONE',  ( 105.1999999999999744, -34.99999999999999289, -100.0000000000000000 ) ) ;
#4849=CARTESIAN_POINT ( 'NONE',  ( 235.3564303562499447, -30.81562499938547717, -50.00000000000011369 ) ) ;
#4852=VERTEX_POINT ( 'NONE', #18337 ) ;
#4866=CARTESIAN_POINT ( 'NONE',  ( 232.5999999999999375, -35.09062499938547575, 103.1828516163667899 ) ) ;
#4872=DIRECTION ( 'NONE',  ( -1.000000000000000000, -0.000000000000000000, -0.000000000000000000 ) ) ;
#4878=CARTESIAN_POINT ( 'NONE',  ( 235.3564303562499447, -33.62812499938547717, -50.00000000000011369 ) ) ;
#4879=CARTESIAN_POINT ( 'NONE',  ( 233.9782151781249411, -31.45312499938548356, 102.3871387122750889 ) ) ;
#4880=CARTESIAN_POINT ( 'NONE',  ( 232.5999999999999375, -31.49062499938547788, -46.81714838363331666 ) ) ;
#4897=CARTESIAN_POINT ( 'NONE',  ( 244.7999999999999545, -5.000000000000000888, -103.0000000000000995 ) ) ;
#4898=CARTESIAN_POINT ( 'NONE',  ( 232.5999999999999375, -33.62812499938547717, 103.1828516163667899 ) ) ;
#4899=CARTESIAN_POINT ( 'NONE',  ( 235.3564303562499447, -31.26562499938547646, 99.99999999999998579 ) ) ;
#4900=VERTEX_POINT ( 'NONE', #18145 ) ;
#4901=CARTESIAN_POINT ( 'NONE',  ( 234.0999999999999375, -31.44374999877096144, 97.40192378864668399 ) ) ;
#4904=ORIENTED_EDGE ( 'NONE', *, *, #18438, .T. ) ;
#4908=CYLINDRICAL_SURFACE ( 'NONE', #1632, 3.000000000000009770 ) ;
#4910=CARTESIAN_POINT ( 'NONE',  ( 231.7961524227065979, -33.45134618820330275, 103.0000000000000000 ) ) ;
#4927=CARTESIAN_POINT ( 'NONE',  ( 229.5999999999999375, -32.73749999999999716, -51.73205080756898866 ) ) ;
#4931=CARTESIAN_POINT ( 'NONE',  ( 232.5999999999999943, -32.39062499938548001, 103.1828516163667899 ) ) ;
#4933=CARTESIAN_POINT ( 'NONE',  ( 232.5999999999999375, -34.41562499938547859, -53.18285161636690361 ) ) ;
#4937=DIRECTION ( 'NONE',  ( 1.000000000000000000, 0.000000000000000000, 0.000000000000000000 ) ) ;
#4941=CARTESIAN_POINT ( 'NONE',  ( 229.8306817459156832, -31.99999999999998579, -49.76128878215637741 ) ) ;
#4949=CARTESIAN_POINT ( 'NONE',  ( 235.3564303562499447, -30.32812499938548001, -51.59142580818350865 ) ) ;
#4952=EDGE_LOOP ( 'NONE', ( #13798, #16150, #7809, #347 ) ) ;
#4954=CARTESIAN_POINT ( 'NONE',  ( 231.7961524227065695, -32.15759618943231857, 102.9999999999999858 ) ) ;
#4955=VECTOR ( 'NONE', #15894, 1000.000000000000000 ) ;
#4959=ORIENTED_EDGE ( 'NONE', *, *, #15335, .F. ) ;
#4962=CARTESIAN_POINT ( 'NONE',  ( 105.2000000000000739, -32.00000000000002842, 147.7999999999999829 ) ) ;
#4967=CARTESIAN_POINT ( 'NONE',  ( 231.2217848218749339, -33.47812499938547859, 97.61286128772489690 ) ) ;
#4971=CARTESIAN_POINT ( 'NONE',  ( 99.99999999999997158, -29.80000000000000071, 150.0000000000000000 ) ) ;
#4973=FACE_OUTER_BOUND ( 'NONE', #16895, .T. ) ;
#4975=PLANE ( 'NONE',  #2756 ) ;
#4981=CARTESIAN_POINT ( 'NONE',  ( 229.8435696437499871, -32.91562499938547859, 101.5914258081833879 ) ) ;
#4982=CARTESIAN_POINT ( 'NONE',  ( 235.3564303562499447, -31.41562499938548214, -48.40857419181671162 ) ) ;
#4986=ORIENTED_EDGE ( 'NONE', *, *, #13211, .T. ) ;
#4988=LINE ( 'NONE', #10931, #19105 ) ;
#4998=CARTESIAN_POINT ( 'NONE',  ( 231.7961524227065695, -33.90134618820329138, -47.00000000000009948 ) ) ;
#5000=CARTESIAN_POINT ( 'NONE',  ( 232.5999999999999375, -33.85312499938547859, 96.81714838363319586 ) ) ;
#5003=ADVANCED_FACE ( 'NONE', ( #10802 ), #16766, .F. ) ;
#5004=CARTESIAN_POINT ( 'NONE',  ( 232.5999999999999375, -31.18124999877096215, 103.4641016151377499 ) ) ;
#5005=CARTESIAN_POINT ( 'NONE',  ( 229.5999999999999375, -32.23124999877096286, 98.26794919243111792 ) ) ;
#5009=CARTESIAN_POINT ( 'NONE',  ( 229.8377951939018828, -35.00000000000002132, -51.08685357171012242 ) ) ;
#5011=CARTESIAN_POINT ( 'NONE',  ( 232.5999999999999375, -34.52812499938548285, -46.81714838363331666 ) ) ;
#5016=DIRECTION ( 'NONE',  ( 4.415659757031858318E-14, 0.000000000000000000, -1.000000000000000000 ) ) ;
#5025=CARTESIAN_POINT ( 'NONE',  ( 234.0999999999999375, -32.39999999999999858, -52.59807621135342970 ) ) ;
#5028=CARTESIAN_POINT ( 'NONE',  ( 235.3564303562499447, -33.14062499938548001, 98.40857419181659793 ) ) ;
#5030=CARTESIAN_POINT ( 'NONE',  ( 231.2217848218749339, -32.57812499938548001, -52.38713871227520968 ) ) ;
#5034=CARTESIAN_POINT ( 'NONE',  ( 233.4038475772933339, -33.91740381056766296, -47.00000000000011369 ) ) ;
#5042=CARTESIAN_POINT ( 'NONE',  ( 232.5999999999999091, -33.03749999999998721, -47.00000000000011369 ) ) ;
#5058=CARTESIAN_POINT ( 'NONE',  ( 231.2217848218749339, -34.67812499938548143, 102.3871387122750889 ) ) ;
#5063=DIRECTION ( 'NONE',  ( -1.000000000000000000, 0.000000000000000000, 0.000000000000000000 ) ) ;
#5066=EDGE_CURVE ( 'NONE', #4350, #6967, #14212, .T. ) ;
#5067=CARTESIAN_POINT ( 'NONE',  ( 231.0999999999999375, -34.87499999999999289, 102.5980762113533018 ) ) ;
#5073=CARTESIAN_POINT ( 'NONE',  ( 235.3564303562499447, -33.62812499938547717, 99.99999999999998579 ) ) ;
#5074=EDGE_CURVE ( 'NONE', #17889, #15031, #8977, .T. ) ;
#5075=CARTESIAN_POINT ( 'NONE',  ( 232.5999999999999375, -30.59062499938547930, -46.81714838363331666 ) ) ;
#5077=LINE ( 'NONE', #17082, #15230 ) ;
#5082=CARTESIAN_POINT ( 'NONE',  ( 105.2000000000000455, -29.80000000000002203, 147.7999999999999829 ) ) ;
#5085=VECTOR ( 'NONE', #3634, 1000.000000000000000 ) ;
#5092=CARTESIAN_POINT ( 'NONE',  ( 235.3564303562499447, -33.96562499938547575, 99.99999999999998579 ) ) ;
#5096=CARTESIAN_POINT ( 'NONE',  ( 234.0999999999999375, -30.69374999877096499, 102.5980762113533018 ) ) ;
#5114=UNCERTAINTY_MEASURE_WITH_UNIT (LENGTH_MEASURE( 1.000000000000000082E-05 ), #17999, 'distance_accuracy_value', 'NONE');
#5121=CARTESIAN_POINT ( 'NONE',  ( 232.5999999999999375, -34.61249999999999716, 97.00000000000000000 ) ) ;
#5125=CARTESIAN_POINT ( 'NONE',  ( 233.9782151781249411, -33.10312499938547859, -52.38713871227520968 ) ) ;
#5129=CARTESIAN_POINT ( 'NONE',  ( 235.5999999999999375, -33.82499999999999574, -50.00000000000011369 ) ) ;
#5136=CARTESIAN_POINT ( 'NONE',  ( 232.5999999999999375, -30.47812499938547859, -46.81714838363331666 ) ) ;
#5150=CARTESIAN_POINT ( 'NONE',  ( 231.2217848218749339, -34.37812499938547717, 97.61286128772489690 ) ) ;
#5159=DIRECTION ( 'NONE',  ( 0.000000000000000000, 0.000000000000000000, -1.000000000000000000 ) ) ;
#5160=VECTOR ( 'NONE', #15747, 1000.000000000000000 ) ;
#5164=CARTESIAN_POINT ( 'NONE',  ( 229.8435696437499303, -33.40312499938547575, 99.99999999999998579 ) ) ;
#5165=CARTESIAN_POINT ( 'NONE',  ( 233.9782151781249411, -33.25312499938547717, -47.61286128772501769 ) ) ;
#5167=CARTESIAN_POINT ( 'NONE',  ( 105.2000000000001307, -29.80000000000002203, 153.0000000000000000 ) ) ;
#5169=ORIENTED_EDGE ( 'NONE', *, *, #9337, .T. ) ;
#5184=CARTESIAN_POINT ( 'NONE',  ( 231.2217848218749339, -33.21562499938547575, 102.3871387122750889 ) ) ;
#5186=EDGE_LOOP ( 'NONE', ( #12551, #1376, #18250, #5684 ) ) ;
#5191=AXIS2_PLACEMENT_3D ( 'NONE', #3440, #18490, #2171 ) ;
#5195=VERTEX_POINT ( 'NONE', #4063 ) ;
#5198=VERTEX_POINT ( 'NONE', #1042 ) ;
#5199=LINE ( 'NONE', #6767, #6350 ) ;
#5202=FACE_OUTER_BOUND ( 'NONE', #5186, .T. ) ;
#5208=CARTESIAN_POINT ( 'NONE',  ( 229.8435696437499303, -35.09062499938547575, 99.99999999999998579 ) ) ;
#5209=ADVANCED_FACE ( 'NONE', ( #17158 ), #849, .T. ) ;
#5214=ORIENTED_EDGE ( 'NONE', *, *, #13730, .T. ) ;
#5215=CARTESIAN_POINT ( 'NONE',  ( 232.5999999999999375, -33.93750000000000000, -46.53589838486234953 ) ) ;
#5217=CARTESIAN_POINT ( 'NONE',  ( 232.5999999999999375, -29.99999999999999645, 99.99999999999998579 ) ) ;
#5218=CARTESIAN_POINT ( 'NONE',  ( 233.9782151781249411, -32.35312499938547859, 102.3871387122750889 ) ) ;
#5221=CARTESIAN_POINT ( 'NONE',  ( 235.3564303562499447, -30.36562499938547788, -50.00000000000011369 ) ) ;
#5226=FACE_OUTER_BOUND ( 'NONE', #12395, .T. ) ;
#5236=CARTESIAN_POINT ( 'NONE',  ( 232.5999999999999375, -33.40312499938547575, -53.18285161636690361 ) ) ;
#5239=ORIENTED_EDGE ( 'NONE', *, *, #12059, .F. ) ;
#5249=B_SPLINE_CURVE_WITH_KNOTS ( 'NONE', 3,
 ( #11094, #17063, #3678, #15603, #2210, #14120, #759, #12658, #11198, #11772 ),
 .UNSPECIFIED., .F., .F.,
 ( 4, 2, 2, 2, 4 ),
 ( 0.3612006186103786654, 0.3925526867148934063, 0.4239047548194081472, 0.4552568229239228881, 0.4866088910284376290 ),
 .UNSPECIFIED. ) ;
#5250=VECTOR ( 'NONE', #17752, 1000.000000000000000 ) ;
#5254=CARTESIAN_POINT ( 'NONE',  ( 231.2217848218749339, -32.46562499938547575, 97.61286128772489690 ) ) ;
#5256=AXIS2_PLACEMENT_3D ( 'NONE', #6926, #11413, #2512 ) ;
#5260=CARTESIAN_POINT ( 'NONE',  ( 249.9999999999999716, -29.80000000000000426, -100.0000000000000000 ) ) ;
#5265=VECTOR ( 'NONE', #18444, 1000.000000000000000 ) ;
#5270=CARTESIAN_POINT ( 'NONE',  ( 231.2217848218749339, -32.57812499938548001, 97.61286128772489690 ) ) ;
#5271=CARTESIAN_POINT ( 'NONE',  ( 233.9782151781249411, -32.80312499938548143, -47.61286128772501769 ) ) ;
#5279=AXIS2_PLACEMENT_3D ( 'NONE', #5360, #19024, #7006 ) ;
#5284=PLANE ( 'NONE',  #17254 ) ;
#5285=DIRECTION ( 'NONE',  ( 0.000000000000000000, 1.000000000000000000, 0.000000000000000000 ) ) ;
#5286=CARTESIAN_POINT ( 'NONE',  ( 230.5523683116323355, -32.00000000000000000, 101.8452947671440540 ) ) ;
#5287=CARTESIAN_POINT ( 'NONE',  ( 235.3564303562499447, -33.06562499938547717, 99.99999999999998579 ) ) ;
#5288=ORIENTED_EDGE ( 'NONE', *, *, #4451, .T. ) ;
#5291=CARTESIAN_POINT ( 'NONE',  ( 244.7999999999999545, -32.00000000000000000, -100.0000000000000000 ) ) ;
#5292=CARTESIAN_POINT ( 'NONE',  ( 229.5999999999999375, -31.78124999877096357, -51.73205080756898866 ) ) ;
#5300=CARTESIAN_POINT ( 'NONE',  ( 231.0999999999999375, -33.16874999877095576, 97.40192378864668399 ) ) ;
#5303=CARTESIAN_POINT ( 'NONE',  ( 99.99999999999997158, -5.200000000000008171, -100.0000000000000000 ) ) ;
#5305=PLANE ( 'NONE',  #8608 ) ;
#5318=CARTESIAN_POINT ( 'NONE',  ( 234.0999999999999375, -33.89999999999999147, -47.40192378864679768 ) ) ;
#5322=CARTESIAN_POINT ( 'NONE',  ( 235.3564303562499447, -33.17812499938548143, 99.99999999999998579 ) ) ;
#5325=CARTESIAN_POINT ( 'NONE',  ( 229.8435696437499871, -30.55312499938547788, -48.40857419181671162 ) ) ;
#5333=CARTESIAN_POINT ( 'NONE',  ( 232.5999999999999943, -32.72812499938547859, -46.81714838363331666 ) ) ;
#5340=CARTESIAN_POINT ( 'NONE',  ( 229.8435696437499871, -32.42812499938548143, -51.59142580818350865 ) ) ;
#5344=CARTESIAN_POINT ( 'NONE',  ( 235.5999999999999375, -34.21874999877096002, -50.00000000000011369 ) ) ;
#5351=CARTESIAN_POINT ( 'NONE',  ( 232.5999999999999375, -34.33124999877097139, -47.00000000000011369 ) ) ;
#5352=CARTESIAN_POINT ( 'NONE',  ( 229.5999999999999375, -34.04999999999999716, -50.00000000000011369 ) ) ;
#5354=CARTESIAN_POINT ( 'NONE',  ( 105.2000000000001307, -29.80000000000002203, 147.7999999999999829 ) ) ;
#5355=ADVANCED_FACE ( 'NONE', ( #16364 ), #7088, .F. ) ;
#5360=CARTESIAN_POINT ( 'NONE',  ( 232.5999999999999375, -29.99999999999999645, -50.00000000000011369 ) ) ;
#5365=CARTESIAN_POINT ( 'NONE',  ( 235.3564303562499447, -34.11562499938548143, 101.5914258081833879 ) ) ;
#5366=CARTESIAN_POINT ( 'NONE',  ( 231.2217848218749339, -33.32812499938548001, -47.61286128772501769 ) ) ;
#5369=CARTESIAN_POINT ( 'NONE',  ( 229.5999999999999375, -32.66249999999999432, -48.26794919243123161 ) ) ;
#5383=CARTESIAN_POINT ( 'NONE',  ( 231.0999999999999375, -32.32499999999999574, -52.59807621135342970 ) ) ;
#5384=PLANE ( 'NONE',  #12556 ) ;
#5385=CARTESIAN_POINT ( 'NONE',  ( 232.5999999999999375, -30.11249999999999716, 96.53589838486223584 ) ) ;
#5386=ORIENTED_EDGE ( 'NONE', *, *, #10187, .T. ) ;
#5388=CARTESIAN_POINT ( 'NONE',  ( 229.5999999999999375, -32.60624999877096997, 101.7320508075688679 ) ) ;
#5389=CARTESIAN_POINT ( 'NONE',  ( 229.5999999999999375, -32.19374999877096144, -50.00000000000011369 ) ) ;
#5399=CARTESIAN_POINT ( 'NONE',  ( 231.7961524227065695, -33.00134618820329990, 103.0000000000000000 ) ) ;
#5408=DIRECTION ( 'NONE',  ( -1.000000000000000000, 9.941108744852765039E-17, 0.000000000000000000 ) ) ;
#5412=AXIS2_PLACEMENT_3D ( 'NONE', #12997, #10448, #13381 ) ;
#5414=VERTEX_POINT ( 'NONE', #2974 ) ;
#5420=CARTESIAN_POINT ( 'NONE',  ( 231.2217848218749339, -34.22812499938548569, 102.3871387122750889 ) ) ;
#5422=CARTESIAN_POINT ( 'NONE',  ( 229.8435696437499303, -30.59062499938547575, -50.00000000000011369 ) ) ;
#5430=CARTESIAN_POINT ( 'NONE',  ( 244.7999999999999545, -32.00000000000002842, 147.7999999999999829 ) ) ;
#5432=CARTESIAN_POINT ( 'NONE',  ( 235.3564303562499447, -32.16562499938547859, -50.00000000000011369 ) ) ;
#5437=CARTESIAN_POINT ( 'NONE',  ( 232.5999999999999375, -33.17812499938548143, -46.81714838363331666 ) ) ;
#5443=CARTESIAN_POINT ( 'NONE',  ( 234.0999999999999375, -34.29374999877096286, -47.40192378864679768 ) ) ;
#5450=CARTESIAN_POINT ( 'NONE',  ( 229.8435696437499303, -32.84062499938547575, 99.99999999999998579 ) ) ;
#5451=CARTESIAN_POINT ( 'NONE',  ( 231.7961524227065695, -33.95759618943232283, -47.00000000000011369 ) ) ;
#5456=CARTESIAN_POINT ( 'NONE',  ( 233.4038475772933054, -33.01740381056766438, 103.0000000000000142 ) ) ;
#5457=CARTESIAN_POINT ( 'NONE',  ( 230.4677467024383191, -31.99999999999999289, 98.24409948398863435 ) ) ;
#5462=CARTESIAN_POINT ( 'NONE',  ( 232.5999999999999375, -33.93749999999999289, 103.0000000000000000 ) ) ;
#5465=CARTESIAN_POINT ( 'NONE',  ( 235.3564303562499447, -34.94062499938547717, 98.40857419181659793 ) ) ;
#5466=CARTESIAN_POINT ( 'NONE',  ( 229.8435696437499303, -32.05312499938548143, -50.00000000000011369 ) ) ;
#5472=ORIENTED_EDGE ( 'NONE', *, *, #2325, .T. ) ;
#5481=CARTESIAN_POINT ( 'NONE',  ( 230.4285530052381716, -35.00000000000000000, 97.92073041325133431 ) ) ;
#5483=CARTESIAN_POINT ( 'NONE',  ( 235.5999999999999943, -31.53749999999999432, 98.26794919243110371 ) ) ;
#5484=( BOUNDED_CURVE ( )  B_SPLINE_CURVE ( 2, ( #2285, #14199, #3945, #5522, #10104, #17437, #5432, #15962, #2664, #17143, #1027, #17529, #8342, #6798, #6889, #933, #8625, #14578, #17336, #12744, #7171, #5333, #14298, #9911, #4048, #19091, #5712, #3748, #9715, #8249, #1602, #8825, #4631, #10484, #10297, #13217, #14979, #8916, #7263, #45, #2961, #4526, #11851, #10584, #14877, #19188, #5805, #16258, #16160, #11756, #18019, #14679, #13415, #1506, #7457, #2866, #7643, #17727, #8726, #19291, #5996, #7360, #14781, #10196, #1314, #6096, #16350, #4337, #11948, #17625, #15072, #17918, #7549, #5905, #16447, #13599, #9019, #10389, #3148, #2771, #16549, #1407, #239 ),
 .UNSPECIFIED., .F., .F. ) 
 B_SPLINE_CURVE_WITH_KNOTS ( ( 3, 2, 2, 2, 2, 2, 2, 2, 2, 2, 2, 2, 2, 2, 2, 2, 2, 2, 2, 2, 2, 2, 2, 2, 2, 2, 2, 2, 2, 2, 2, 2, 2, 2, 2, 2, 2, 2, 2, 2, 2, 3 ),
 ( 0.3716916592826016719, 0.3750191855951751085, 0.3900199530189821240, 0.4050207204427891394, 0.4200214878665962104, 0.4350222552904032258, 0.4500230227142102413, 0.4650237901380172567, 0.4800245575618242166, 0.4950253249856312321, 0.5100260924094381920, 0.5250268598332452630, 0.5400276272570523339, 0.5550283946808592939, 0.5700291621046663648, 0.5850299295284733248, 0.6000306969522803957, 0.6150314643760873556, 0.6300322317998944266, 0.6450329992237013865, 0.6600337666475084575, 0.6750345340713154174, 0.6900353014951223773, 0.7050360689189294483, 0.7200368363427364082, 0.7350376037665435902, 0.7500383711903504391, 0.7650391386141575101, 0.7800399060379645810, 0.7950406734617716520, 0.8100414408855785009, 0.8250422083093855719, 0.8400429757331926428, 0.8550437431569996027, 0.8700445105808065627, 0.8850452780046136336, 0.9000460454284207046, 0.9150468128522275535, 0.9300475802760346244, 0.9450483476998416954, 0.9600491151236485443, 0.9717223562348840105 ),
 .UNSPECIFIED. ) 
 CURVE ( )  GEOMETRIC_REPRESENTATION_ITEM ( )  RATIONAL_B_SPLINE_CURVE ( ( 0.9537471549767071455, 0.9702812541832913640, 1.000000000000000000, 0.8660254037844387076, 1.000000000000000000, 0.8660254037844387076, 1.000000000000000000, 0.8660254037844387076, 1.000000000000000000, 0.8660254037844387076, 1.000000000000000000, 0.8660254037844387076, 1.000000000000000000, 0.8660254037844387076, 1.000000000000000000, 0.8660254037844387076, 1.000000000000000000, 0.8660254037844387076, 1.000000000000000000, 0.8660254037844387076, 1.000000000000000000, 0.8660254037844387076, 1.000000000000000000, 0.8660254037844387076, 1.000000000000000000, 0.8660254037844387076, 1.000000000000000000, 0.8660254037844387076, 1.000000000000000000, 0.8660254037844387076, 1.000000000000000000, 0.8660254037844387076, 1.000000000000000000, 0.8660254037844387076, 1.000000000000000000, 0.8660254037844387076, 1.000000000000000000, 0.8660254037844387076, 1.000000000000000000, 0.8660254037844387076, 1.000000000000000000, 0.8660254037844387076, 1.000000000000000000, 0.8660254037844387076, 1.000000000000000000, 0.8660254037844387076, 1.000000000000000000, 0.8660254037844387076, 1.000000000000000000, 0.8660254037844387076, 1.000000000000000000, 0.8660254037844387076, 1.000000000000000000, 0.8660254037844387076, 1.000000000000000000, 0.8660254037844387076, 1.000000000000000000, 0.8660254037844387076, 1.000000000000000000, 0.8660254037844387076, 1.000000000000000000, 0.8660254037844387076, 1.000000000000000000, 0.8660254037844387076, 1.000000000000000000, 0.8660254037844387076, 1.000000000000000000, 0.8660254037844387076, 1.000000000000000000, 0.8660254037844387076, 1.000000000000000000, 0.8660254037844387076, 1.000000000000000000, 0.8660254037844387076, 1.000000000000000000, 0.8660254037844387076, 1.000000000000000000, 0.8660254037844387076, 1.000000000000000000, 0.8660254037844387076, 1.000000000000000000, 0.8957441496011311344, 0.9537471549767251311 ) ) 
 REPRESENTATION_ITEM ( '' )  );
#5488=CARTESIAN_POINT ( 'NONE',  ( 232.5999999999999375, -32.08124999877095718, 103.4641016151377499 ) ) ;
#5492=ORIENTED_EDGE ( 'NONE', *, *, #5896, .T. ) ;
#5495=CARTESIAN_POINT ( 'NONE',  ( 232.5999999999999375, -33.65624999877096002, -53.00000000000011369 ) ) ;
#5496=VERTEX_POINT ( 'NONE', #18223 ) ;
#5505=DIRECTION ( 'NONE',  ( 0.000000000000000000, 1.000000000000000000, 0.000000000000000000 ) ) ;
#5509=ORIENTED_EDGE ( 'NONE', *, *, #9593, .T. ) ;
#5510=CARTESIAN_POINT ( 'NONE',  ( 231.6691923799541826, -35.05289549976082952, -53.55789078125459923 ) ) ;
#5512=LINE ( 'NONE', #4130, #5853 ) ;
#5513=CARTESIAN_POINT ( 'NONE',  ( 0.000000000000000000, 0.000000000000000000, 150.0000000000000000 ) ) ;
#5515=CARTESIAN_POINT ( 'NONE',  ( 232.5999999999999375, -30.47812499938547859, -46.81714838363331666 ) ) ;
#5516=EDGE_LOOP ( 'NONE', ( #2348, #4717, #11356, #462 ) ) ;
#5522=CARTESIAN_POINT ( 'NONE',  ( 232.5999999999999943, -32.05312499938548143, -53.18285161636690361 ) ) ;
#5527=CARTESIAN_POINT ( 'NONE',  ( 229.8435696437499303, -32.84062499938547575, -50.00000000000011369 ) ) ;
#5532=CARTESIAN_POINT ( 'NONE',  ( 232.5999999999999659, -32.58749999999999858, -47.00000000000011369 ) ) ;
#5534=( BOUNDED_CURVE ( )  B_SPLINE_CURVE ( 2, ( #5351, #14315, #7972, #17062, #2012, #14029, #15698, #15501, #2209 ),
 .UNSPECIFIED., .F., .F. ) 
 B_SPLINE_CURVE_WITH_KNOTS ( ( 3, 2, 2, 2, 3 ),
 ( 0.7291666666666665186, 0.7361111111111111605, 0.7500000000000000000, 0.7638888888888888395, 0.7708333333333332593 ),
 .UNSPECIFIED. ) 
 CURVE ( )  GEOMETRIC_REPRESENTATION_ITEM ( )  RATIONAL_B_SPLINE_CURVE ( ( 0.9330127018922194093, 0.9330127018922177440, 1.000000000000000000, 0.8660254037844387076, 1.000000000000000000, 0.8660254037844387076, 1.000000000000000000, 0.9330127018922198534, 0.9330127018922192983 ) ) 
 REPRESENTATION_ITEM ( '' )  );
#5537=ADVANCED_BREP_SHAPE_REPRESENTATION ( '', ( #3102, #10540 ), #13638 ) ;
#5542=CARTESIAN_POINT ( 'NONE',  ( 233.9782151781249411, -33.44062499938547717, 97.61286128772489690 ) ) ;
#5549=CARTESIAN_POINT ( 'NONE',  ( 99.99999999999997158, -34.99999999999999289, -100.0000000000000000 ) ) ;
#5557=CARTESIAN_POINT ( 'NONE',  ( 233.9782151781249411, -34.00312499938547717, 97.61286128772489690 ) ) ;
#5558=CARTESIAN_POINT ( 'NONE',  ( 231.2217848218749339, -32.42812499938548143, -47.61286128772501769 ) ) ;
#5568=VERTEX_POINT ( 'NONE', #832 ) ;
#5569=CARTESIAN_POINT ( 'NONE',  ( 231.0999999999999375, -33.67499999999999716, -52.59807621135342970 ) ) ;
#5573=CARTESIAN_POINT ( 'NONE',  ( 235.3564303562499447, -30.47812499938547859, 99.99999999999998579 ) ) ;
#5578=CARTESIAN_POINT ( 'NONE',  ( 232.6775203606193543, -35.00000000000000711, 102.7610832838413728 ) ) ;
#5580=CARTESIAN_POINT ( 'NONE',  ( 231.0999999999999375, -32.17499999999999716, 102.5980762113533018 ) ) ;
#5584=CARTESIAN_POINT ( 'NONE',  ( 229.5999999999999375, -33.13124999877096144, 98.26794919243111792 ) ) ;
#5589=ORIENTED_EDGE ( 'NONE', *, *, #18015, .T. ) ;
#5593=VERTEX_POINT ( 'NONE', #3938 ) ;
#5594=LINE ( 'NONE', #5303, #17269 ) ;
#5600=CARTESIAN_POINT ( 'NONE',  ( 234.6787480663869587, -35.00000000000000000, -52.02344717699244825 ) ) ;
#5601=CARTESIAN_POINT ( 'NONE',  ( 244.7999999999999545, -29.80000000000000782, -100.0000000000000000 ) ) ;
#5602=DIRECTION ( 'NONE',  ( 0.000000000000000000, 0.000000000000000000, 1.000000000000000000 ) ) ;
#5609=CARTESIAN_POINT ( 'NONE',  ( 234.1461053235294116, -35.00000000000001421, 97.51091559654268792 ) ) ;
#5611=CARTESIAN_POINT ( 'NONE',  ( 233.9782151781249411, -34.15312499938547575, 102.3871387122750889 ) ) ;
#5613=CYLINDRICAL_SURFACE ( 'NONE', #11292, 3.000000000000002665 ) ;
#5614=CARTESIAN_POINT ( 'NONE',  ( 232.5999999999999375, -34.64062499938548001, -46.81714838363331666 ) ) ;
#5615=ORIENTED_EDGE ( 'NONE', *, *, #11611, .F. ) ;
#5620=CARTESIAN_POINT ( 'NONE',  ( 229.8435696437499303, -30.59062499938547575, 99.99999999999998579 ) ) ;
#5625=CARTESIAN_POINT ( 'NONE',  ( 232.5999999999999375, -31.01249999999999218, -53.46410161513786363 ) ) ;
#5636=FACE_OUTER_BOUND ( 'NONE', #4016, .T. ) ;
#5651=CARTESIAN_POINT ( 'NONE',  ( 231.2217848218749339, -34.67812499938548143, 102.3871387122750889 ) ) ;
#5652=CARTESIAN_POINT ( 'NONE',  ( 231.2217848218749339, -34.67812499938548143, -47.61286128772501769 ) ) ;
#5660=ORIENTED_EDGE ( 'NONE', *, *, #12059, .T. ) ;
#5667=EDGE_CURVE ( 'NONE', #16293, #11985, #4795, .T. ) ;
#5670=CARTESIAN_POINT ( 'NONE',  ( 234.8201511961208610, -35.00000000000002842, 101.6434491389464085 ) ) ;
#5672=CARTESIAN_POINT ( 'NONE',  ( 235.5999999999999375, -30.67499999999999361, 99.99999999999998579 ) ) ;
#5676=CARTESIAN_POINT ( 'NONE',  ( 235.5999999999999943, -32.00624999877096144, 101.7320508075688537 ) ) ;
#5677=CARTESIAN_POINT ( 'NONE',  ( 235.5999999999999375, -31.51874999877096073, -50.00000000000011369 ) ) ;
#5681=VERTEX_POINT ( 'NONE', #7710 ) ;
#5684=ORIENTED_EDGE ( 'NONE', *, *, #2906, .F. ) ;
#5692=DIRECTION ( 'NONE',  ( 1.000000000000000000, 0.000000000000000000, 0.000000000000000000 ) ) ;
#5698=CARTESIAN_POINT ( 'NONE',  ( 233.9782151781249411, -34.45312499938548001, 97.61286128772489690 ) ) ;
#5701=CARTESIAN_POINT ( 'NONE',  ( 229.8435696437499871, -33.32812499938548001, -51.59142580818350865 ) ) ;
#5711=CARTESIAN_POINT ( 'NONE',  ( 235.3564303562499447, -32.57812499938547290, 98.40857419181659793 ) ) ;
#5712=CARTESIAN_POINT ( 'NONE',  ( 231.2217848218749339, -32.91562499938547148, -52.38713871227520968 ) ) ;
#5716=CARTESIAN_POINT ( 'NONE',  ( 231.0999999999999375, -31.42499999999999361, -52.59807621135342970 ) ) ;
#5719=VERTEX_POINT ( 'NONE', #10355 ) ;
#5723=CARTESIAN_POINT ( 'NONE',  ( 229.8435696437499303, -30.70312499938548001, -50.00000000000011369 ) ) ;
#5728=CARTESIAN_POINT ( 'NONE',  ( 235.3564303562499447, -33.47812499938547859, 98.40857419181659793 ) ) ;
#5732=CARTESIAN_POINT ( 'NONE',  ( 231.2583267490322783, -32.00000000000000000, -47.53412486788969460 ) ) ;
#5739=ORIENTED_EDGE ( 'NONE', *, *, #2325, .F. ) ;
#5741=CARTESIAN_POINT ( 'NONE',  ( 234.4730806518346924, -35.00000000000004263, -47.94626448418657105 ) ) ;
#5743=CARTESIAN_POINT ( 'NONE',  ( 234.0999999999999375, -34.29374999877096286, 102.5980762113533018 ) ) ;
#5745=ORIENTED_EDGE ( 'NONE', *, *, #13934, .T. ) ;
#5748=ORIENTED_EDGE ( 'NONE', *, *, #15939, .F. ) ;
#5753=CARTESIAN_POINT ( 'NONE',  ( 233.9782151781249411, -31.45312499938548356, 102.3871387122750889 ) ) ;
#5758=CARTESIAN_POINT ( 'NONE',  ( 231.7961524227065695, -32.15759618943231857, -47.00000000000010658 ) ) ;
#5760=CARTESIAN_POINT ( 'NONE',  ( 229.5999999999999375, -32.21249999999999858, 101.7320508075688679 ) ) ;
#5763=CARTESIAN_POINT ( 'NONE',  ( 232.5999999999999375, -33.65624999877096002, 96.53589838486223584 ) ) ;
#5764=CARTESIAN_POINT ( 'NONE',  ( 234.0999999999999375, -32.79374999877096286, -52.59807621135342970 ) ) ;
#5766=VERTEX_POINT ( 'NONE', #11822 ) ;
#5767=VERTEX_POINT ( 'NONE', #8883 ) ;
#5769=ADVANCED_FACE ( 'NONE', ( #14842 ), #8101, .T. ) ;
#5771=CARTESIAN_POINT ( 'NONE',  ( 233.4038475772933339, -34.18259618943231715, -53.00000000000011369 ) ) ;
#5772=EDGE_LOOP ( 'NONE', ( #13611, #15376, #12036, #11824, #17883, #13763, #14671, #14544, #10950, #1539, #4530, #13500, #356, #18146, #2833, #4485, #16249 ) ) ;
#5775=DIRECTION ( 'NONE',  ( 0.000000000000000000, 0.000000000000000000, 1.000000000000000000 ) ) ;
#5786=CARTESIAN_POINT ( 'NONE',  ( 232.5999999999999375, -33.43124999877096570, -47.00000000000011369 ) ) ;
#5788=CARTESIAN_POINT ( 'NONE',  ( 102.9999999999999858, -5.200000000000008171, 150.0000000000000000 ) ) ;
#5789=CARTESIAN_POINT ( 'NONE',  ( 235.3564303562499447, -33.62812499938547717, 99.99999999999998579 ) ) ;
#5793=CARTESIAN_POINT ( 'NONE',  ( 235.3564303562499447, -33.51562499938548001, -50.00000000000011369 ) ) ;
#5803=CARTESIAN_POINT ( 'NONE',  ( 229.8435696437499303, -31.49062499938547788, 99.99999999999998579 ) ) ;
#5805=CARTESIAN_POINT ( 'NONE',  ( 231.2217848218749339, -33.66562499938547859, -47.61286128772501769 ) ) ;
#5806=FACE_OUTER_BOUND ( 'NONE', #783, .T. ) ;
#5810=CARTESIAN_POINT ( 'NONE',  ( 232.5999999999999375, -30.33749999999999503, -46.53589838486234953 ) ) ;
#5816=CARTESIAN_POINT ( 'NONE',  ( 234.0999999999999375, -32.94374999877096144, 102.5980762113533018 ) ) ;
#5817=CARTESIAN_POINT ( 'NONE',  ( 232.5999999999999375, -31.94062499938548072, -46.81714838363331666 ) ) ;
#5820=VERTEX_POINT ( 'NONE', #9267 ) ;
#5822=CARTESIAN_POINT ( 'NONE',  ( 231.2217848218749339, -32.31562499938547717, 102.3871387122750889 ) ) ;
#5826=DIRECTION ( 'NONE',  ( 0.000000000000000000, 2.001604010742465719E-15, -1.000000000000000000 ) ) ;
#5832=CARTESIAN_POINT ( 'NONE',  ( 231.0999999999999375, -33.22499999999999432, -52.59807621135342970 ) ) ;
#5838=FACE_OUTER_BOUND ( 'NONE', #10290, .T. ) ;
#5839=CARTESIAN_POINT ( 'NONE',  ( 231.7961524227065979, -34.85759618943232852, -47.00000000000011369 ) ) ;
#5842=ORIENTED_EDGE ( 'NONE', *, *, #8076, .F. ) ;
#5845=DIRECTION ( 'NONE',  ( -1.000000000000000000, -0.000000000000000000, -0.000000000000000000 ) ) ;
#5846=ORIENTED_EDGE ( 'NONE', *, *, #4830, .F. ) ;
#5847=CARTESIAN_POINT ( 'NONE',  ( 232.5999999999999375, -33.48749999999999716, -47.00000000000011369 ) ) ;
#5851=CARTESIAN_POINT ( 'NONE',  ( 235.3564303562499447, -32.69062499938547717, 98.40857419181659793 ) ) ;
#5853=VECTOR ( 'NONE', #8425, 1000.000000000000000 ) ;
#5857=LINE ( 'NONE', #6051, #9262 ) ;
#5860=CARTESIAN_POINT ( 'NONE',  ( 231.0999999999999375, -34.57499999999999574, 97.40192378864668399 ) ) ;
#5862=CARTESIAN_POINT ( 'NONE',  ( 234.0999999999999375, -34.59374999877096002, 97.40192378864668399 ) ) ;
#5864=CARTESIAN_POINT ( 'NONE',  ( 229.5999999999999375, -34.40624999877096002, 101.7320508075688679 ) ) ;
#5865=CARTESIAN_POINT ( 'NONE',  ( 231.0999999999999375, -34.51874999877096428, -52.59807621135342970 ) ) ;
#5868=ORIENTED_EDGE ( 'NONE', *, *, #7452, .F. ) ;
#5876=AXIS2_PLACEMENT_3D ( 'NONE', #7777, #3275, #6320 ) ;
#5877=VECTOR ( 'NONE', #8821, 1000.000000000000000 ) ;
#5881=CARTESIAN_POINT ( 'NONE',  ( 235.3193635794330589, -31.99999999999998579, -51.26521311181414831 ) ) ;
#5884=CARTESIAN_POINT ( 'NONE',  ( 244.7999999999999545, -34.51168759575592304, 150.0000000000000000 ) ) ;
#5885=CARTESIAN_POINT ( 'NONE',  ( 232.5999999999999375, -30.92812499938547433, 103.1828516163667899 ) ) ;
#5886=ORIENTED_EDGE ( 'NONE', *, *, #8993, .F. ) ;
#5893=CARTESIAN_POINT ( 'NONE',  ( 105.1999999999999744, -31.99999999999999289, -100.0000000000000000 ) ) ;
#5894=CARTESIAN_POINT ( 'NONE',  ( 229.8435696437499871, -32.35312499938547859, -48.40857419181671162 ) ) ;
#5895=ADVANCED_FACE ( 'NONE', ( #3698 ), #6737, .F. ) ;
#5896=EDGE_CURVE ( 'NONE', #10687, #13854, #4988, .T. ) ;
#5904=CARTESIAN_POINT ( 'NONE',  ( 231.2217848218749339, -32.91562499938547148, 97.61286128772489690 ) ) ;
#5905=CARTESIAN_POINT ( 'NONE',  ( 229.8435696437499587, -34.67812499938547433, -51.59142580818350154 ) ) ;
#5909=CARTESIAN_POINT ( 'NONE',  ( 231.2217848218749339, -35.01562499938548001, -47.61286128772501769 ) ) ;
#5914=CARTESIAN_POINT ( 'NONE',  ( 249.9999999999999716, -5.000000000000004441, -100.0000000000000000 ) ) ;
#5918=EDGE_LOOP ( 'NONE', ( #1075, #10488, #9411, #4582 ) ) ;
#5920=CARTESIAN_POINT ( 'NONE',  ( 233.9782151781249411, -34.34062499938547575, 97.61286128772489690 ) ) ;
#5924=PLANE ( 'NONE',  #7657 ) ;
#5925=CARTESIAN_POINT ( 'NONE',  ( 232.8441546701661480, -32.00000000000000000, -47.13032736203121686 ) ) ;
#5936=CARTESIAN_POINT ( 'NONE',  ( 233.9782151781249411, -34.90312499938547575, -52.38713871227520968 ) ) ;
#5943=ADVANCED_FACE ( 'NONE', ( #17377 ), #15720, .F. ) ;
#5945=CARTESIAN_POINT ( 'NONE',  ( 229.5999999999999375, -33.58124999877096428, -51.73205080756898866 ) ) ;
#5947=CARTESIAN_POINT ( 'NONE',  ( 231.2217848218749339, -33.02812499938547575, 97.61286128772489690 ) ) ;
#5952=( BOUNDED_CURVE ( )  B_SPLINE_CURVE ( 2, ( #16300, #8674, #4282, #7500, #10526, #3001, #2910, #2815, #186 ),
 .UNSPECIFIED., .F., .F. ) 
 B_SPLINE_CURVE_WITH_KNOTS ( ( 3, 2, 2, 2, 3 ),
 ( 0.8125000000000000000, 0.8194444444444444198, 0.8333333333333333703, 0.8472222222222222099, 0.8541666666666668517 ),
 .UNSPECIFIED. ) 
 CURVE ( )  GEOMETRIC_REPRESENTATION_ITEM ( )  RATIONAL_B_SPLINE_CURVE ( ( 0.9330127018922194093, 0.9330127018922194093, 1.000000000000000000, 0.8660254037844387076, 1.000000000000000000, 0.8660254037844387076, 1.000000000000000000, 0.9330127018922177440, 0.9330127018922194093 ) ) 
 REPRESENTATION_ITEM ( '' )  );
#5955=CARTESIAN_POINT ( 'NONE',  ( 229.5999999999999375, -33.60000000000000142, 99.99999999999998579 ) ) ;
#5959=CARTESIAN_POINT ( 'NONE',  ( 229.5999999999999375, -34.89374999877096428, 99.99999999999998579 ) ) ;
#5960=CARTESIAN_POINT ( 'NONE',  ( 229.5999999999999375, -32.60624999877096997, -48.26794919243123161 ) ) ;
#5964=ORIENTED_EDGE ( 'NONE', *, *, #14175, .F. ) ;
#5967=CYLINDRICAL_SURFACE ( 'NONE', #15983, 3.000000000000002665 ) ;
#5979=ORIENTED_EDGE ( 'NONE', *, *, #16290, .F. ) ;
#5983=DIRECTION ( 'NONE',  ( -0.000000000000000000, -1.000000000000000000, -0.000000000000000000 ) ) ;
#5986=CARTESIAN_POINT ( 'NONE',  ( 235.3564303562499447, -32.57812499938547290, -51.59142580818350865 ) ) ;
#5987=( BOUNDED_CURVE ( )  B_SPLINE_CURVE ( 2, ( #11639, #6870, #17600, #4213, #10172, #11730, #16135, #2745, #8706 ),
 .UNSPECIFIED., .F., .F. ) 
 B_SPLINE_CURVE_WITH_KNOTS ( ( 3, 2, 2, 2, 3 ),
 ( 0.3541666666666666852, 0.3611111111111111049, 0.3750000000000000000, 0.3888888888888888951, 0.3958333333333333703 ),
 .UNSPECIFIED. ) 
 CURVE ( )  GEOMETRIC_REPRESENTATION_ITEM ( )  RATIONAL_B_SPLINE_CURVE ( ( 0.9330127018922194093, 0.9330127018922196314, 1.000000000000000000, 0.8660254037844387076, 1.000000000000000000, 0.8660254037844387076, 1.000000000000000000, 0.9330127018922190762, 0.9330127018922194093 ) ) 
 REPRESENTATION_ITEM ( '' )  );
#5988=ORIENTED_EDGE ( 'NONE', *, *, #19190, .T. ) ;
#5995=CARTESIAN_POINT ( 'NONE',  ( 233.9782151781249411, -34.04062499938547859, 102.3871387122750889 ) ) ;
#5996=CARTESIAN_POINT ( 'NONE',  ( 229.8435696437499303, -34.19062499938547717, -50.00000000000011369 ) ) ;
#6002=CARTESIAN_POINT ( 'NONE',  ( 231.2217848218749339, -34.56562499938547717, -47.61286128772501769 ) ) ;
#6006=CARTESIAN_POINT ( 'NONE',  ( 229.8435696437499871, -32.01562499938548001, -48.40857419181671162 ) ) ;
#6035=( BOUNDED_SURFACE ( )  B_SPLINE_SURFACE ( 1, 2, ( 
 ( #11531, #2446, #14165, #11435, #8305, #4104, #15642, #14446, #17396, #18767, #13086, #7036, #15834, #8588, #12991, #3906, #18963, #4011, #14541, #798, #9974, #19055, #17494, #15928, #2530, #17201, #1177, #10065, #3715, #2626, #5677, #9680, #8491, #8217, #12701, #18675, #9776, #5292, #14353, #11238, #8401, #2344, #14258, #9872, #896, #989, #6855, #12801, #5389, #11335, #17300, #17786, #11, #17976, #3017, #10546, #16122, #4489, #14738, #5960, #16508, #17586, #11908, #8692, #5764, #3111, #15034, #4198, #13469, #1657, #1462, #8784, #16407, #6059, #14941, #9070, #7416, #2830, #1566, #7609, #10159, #14642, #12005, #16315, #1276, #17881, #1373, #4586, #2730, #8975, #13377, #13273, #13561, #7512, #10350, #202, #108, #4393, #11621, #10443, #7223, #13178, #19151, #11716, #17684, #4297, #10261, #16224, #7320, #19248, #5865, #11817, #2924, #8876, #14836, #8094, #10636, #16602, #12197, #2137, #3405, #15519, #16795, #3207, #302, #18264, #9166, #9359, #15130, #15420, #1843, #9454, #1746, #12298, #13846 ),
 ( #394, #14047, #13756, #15319, #6153, #18167, #4789, #13947, #12103, #5075, #7704, #13662, #7801, #6252, #15228, #16892, #16694, #10731, #7896, #2031, #3303, #6440, #12484, #18453, #6346, #7991, #1935, #10923, #18077, #4685, #3495, #4982, #9261, #4880, #10823, #487, #12391, #18360, #588, #6538, #11015, #16981, #3593, #9553, #17370, #11111, #6728, #10042, #5466, #2510, #14140, #775, #2416, #11508, #11216, #8467, #17079, #682, #5558, #12967, #3982, #9948, #18844, #8380, #3884, #9848, #18648, #14232, #5271, #1058, #15811, #870, #4080, #11410, #6835, #12779, #15905, #17181, #18748, #14424, #5165, #9659, #5366, #7014, #6924, #8190, #6633, #18938, #12872, #3785, #12675, #14331, #969, #12582, #17469, #16000, #2319, #9751, #2604, #15715, #8565, #2224, #18548, #3693, #15619, #8283, #11314, #17279, #7200, #13352, #16381, #13445, #2806, #11691, #2703, #19030, #1249, #10516, #5652, #14913, #2900, #10137, #14810, #13617, #5936, #17851, #11979, #1436, #7109, #17762, #16097, #4369, #8661, #2991, #8759 ) ),
 .UNSPECIFIED., .F., .F., .F. ) 
 B_SPLINE_SURFACE_WITH_KNOTS ( ( 2, 2 ),
 ( 3, 2, 2, 2, 2, 2, 2, 2, 2, 2, 2, 2, 2, 2, 2, 2, 2, 2, 2, 2, 2, 2, 2, 2, 2, 2, 2, 2, 2, 2, 2, 2, 2, 2, 2, 2, 2, 2, 2, 2, 2, 2, 2, 2, 2, 2, 2, 2, 2, 2, 2, 2, 2, 2, 2, 2, 2, 2, 2, 2, 2, 2, 2, 2, 2, 2, 2, 3 ),
 ( 0.000000000000000000, 1.000000000000000000 ),
 ( 0.000000000000000000, 0.01388888888888888812, 0.02777777777777777624, 0.04166666666666666435, 0.05555555555555555247, 0.06944444444444444753, 0.08333333333333332871, 0.09722222222222222376, 0.1111111111111111049, 0.1250000000000000000, 0.1388888888888888951, 0.1527777777777777901, 0.1666666666666666574, 0.1805555555555555525, 0.1944444444444444475, 0.2083333333333333426, 0.2222222222222222099, 0.2361111111111111049, 0.2500000000000000000, 0.2638888888888888951, 0.2777777777777777901, 0.2916666666666666852, 0.3055555555555555802, 0.3194444444444444198, 0.3333333333333333148, 0.3472222222222222099, 0.3611111111111111049, 0.3750000000000000000, 0.3888888888888888951, 0.4027777777777777901, 0.4166666666666666852, 0.4305555555555555802, 0.4444444444444444198, 0.4583333333333333148, 0.4722222222222222099, 0.4861111111111111049, 0.5000000000000000000, 0.5138888888888888395, 0.5277777777777777901, 0.5416666666666666297, 0.5555555555555555802, 0.5694444444444444198, 0.5833333333333333703, 0.5972222222222222099, 0.6111111111111111605, 0.6250000000000000000, 0.6388888888888888395, 0.6527777777777777901, 0.6666666666666666297, 0.6805555555555555802, 0.6944444444444444198, 0.7083333333333333703, 0.7222222222222222099, 0.7361111111111111605, 0.7500000000000000000, 0.7638888888888888395, 0.7777777777777777901, 0.7916666666666666297, 0.8055555555555555802, 0.8194444444444444198, 0.8333333333333333703, 0.8472222222222222099, 0.8611111111111111605, 0.8750000000000000000, 0.8888888888888888395, 0.9027777777777777901, 0.9166666666666666297, 0.9258785144422092550 ),
 .UNSPECIFIED. ) 
 GEOMETRIC_REPRESENTATION_ITEM ( )  RATIONAL_B_SPLINE_SURFACE ( (
 ( 1.000000000000000000, 0.8660254037844387076, 1.000000000000000000, 0.8660254037844387076, 1.000000000000000000, 0.8660254037844387076, 1.000000000000000000, 0.8660254037844387076, 1.000000000000000000, 0.8660254037844387076, 1.000000000000000000, 0.8660254037844387076, 1.000000000000000000, 0.8660254037844387076, 1.000000000000000000, 0.8660254037844387076, 1.000000000000000000, 0.8660254037844387076, 1.000000000000000000, 0.8660254037844387076, 1.000000000000000000, 0.8660254037844387076, 1.000000000000000000, 0.8660254037844387076, 1.000000000000000000, 0.8660254037844387076, 1.000000000000000000, 0.8660254037844387076, 1.000000000000000000, 0.8660254037844387076, 1.000000000000000000, 0.8660254037844387076, 1.000000000000000000, 0.8660254037844387076, 1.000000000000000000, 0.8660254037844387076, 1.000000000000000000, 0.8660254037844387076, 1.000000000000000000, 0.8660254037844387076, 1.000000000000000000, 0.8660254037844387076, 1.000000000000000000, 0.8660254037844387076, 1.000000000000000000, 0.8660254037844387076, 1.000000000000000000, 0.8660254037844387076, 1.000000000000000000, 0.8660254037844387076, 1.000000000000000000, 0.8660254037844387076, 1.000000000000000000, 0.8660254037844387076, 1.000000000000000000, 0.8660254037844387076, 1.000000000000000000, 0.8660254037844387076, 1.000000000000000000, 0.8660254037844387076, 1.000000000000000000, 0.8660254037844387076, 1.000000000000000000, 0.8660254037844387076, 1.000000000000000000, 0.8660254037844387076, 1.000000000000000000, 0.8660254037844387076, 1.000000000000000000, 0.8660254037844387076, 1.000000000000000000, 0.8660254037844387076, 1.000000000000000000, 0.8660254037844387076, 1.000000000000000000, 0.8660254037844387076, 1.000000000000000000, 0.8660254037844387076, 1.000000000000000000, 0.8660254037844387076, 1.000000000000000000, 0.8660254037844387076, 1.000000000000000000, 0.8660254037844387076, 1.000000000000000000, 0.8660254037844387076, 1.000000000000000000, 0.8660254037844387076, 1.000000000000000000, 0.8660254037844387076, 1.000000000000000000, 0.8660254037844387076, 1.000000000000000000, 0.8660254037844387076, 1.000000000000000000, 0.8660254037844387076, 1.000000000000000000, 0.8660254037844387076, 1.000000000000000000, 0.8660254037844387076, 1.000000000000000000, 0.8660254037844387076, 1.000000000000000000, 0.8660254037844387076, 1.000000000000000000, 0.8660254037844387076, 1.000000000000000000, 0.8660254037844387076, 1.000000000000000000, 0.8660254037844387076, 1.000000000000000000, 0.8660254037844387076, 1.000000000000000000, 0.8660254037844387076, 1.000000000000000000, 0.8660254037844387076, 1.000000000000000000, 0.8660254037844387076, 1.000000000000000000, 0.8660254037844387076, 1.000000000000000000, 0.8660254037844387076, 1.000000000000000000, 0.8660254037844387076, 1.000000000000000000, 0.8660254037844387076, 1.000000000000000000, 0.8660254037844387076, 1.000000000000000000, 0.8660254037844387076, 1.000000000000000000, 0.8660254037844387076, 1.000000000000000000, 0.9111409417988175496, 0.9401539645359766606),
 ( 1.000000000000000000, 0.8660254037844387076, 1.000000000000000000, 0.8660254037844387076, 1.000000000000000000, 0.8660254037844387076, 1.000000000000000000, 0.8660254037844387076, 1.000000000000000000, 0.8660254037844387076, 1.000000000000000000, 0.8660254037844387076, 1.000000000000000000, 0.8660254037844387076, 1.000000000000000000, 0.8660254037844387076, 1.000000000000000000, 0.8660254037844387076, 1.000000000000000000, 0.8660254037844387076, 1.000000000000000000, 0.8660254037844387076, 1.000000000000000000, 0.8660254037844387076, 1.000000000000000000, 0.8660254037844387076, 1.000000000000000000, 0.8660254037844387076, 1.000000000000000000, 0.8660254037844387076, 1.000000000000000000, 0.8660254037844387076, 1.000000000000000000, 0.8660254037844387076, 1.000000000000000000, 0.8660254037844387076, 1.000000000000000000, 0.8660254037844387076, 1.000000000000000000, 0.8660254037844387076, 1.000000000000000000, 0.8660254037844387076, 1.000000000000000000, 0.8660254037844387076, 1.000000000000000000, 0.8660254037844387076, 1.000000000000000000, 0.8660254037844387076, 1.000000000000000000, 0.8660254037844387076, 1.000000000000000000, 0.8660254037844387076, 1.000000000000000000, 0.8660254037844387076, 1.000000000000000000, 0.8660254037844387076, 1.000000000000000000, 0.8660254037844387076, 1.000000000000000000, 0.8660254037844387076, 1.000000000000000000, 0.8660254037844387076, 1.000000000000000000, 0.8660254037844387076, 1.000000000000000000, 0.8660254037844387076, 1.000000000000000000, 0.8660254037844387076, 1.000000000000000000, 0.8660254037844387076, 1.000000000000000000, 0.8660254037844387076, 1.000000000000000000, 0.8660254037844387076, 1.000000000000000000, 0.8660254037844387076, 1.000000000000000000, 0.8660254037844387076, 1.000000000000000000, 0.8660254037844387076, 1.000000000000000000, 0.8660254037844387076, 1.000000000000000000, 0.8660254037844387076, 1.000000000000000000, 0.8660254037844387076, 1.000000000000000000, 0.8660254037844387076, 1.000000000000000000, 0.8660254037844387076, 1.000000000000000000, 0.8660254037844387076, 1.000000000000000000, 0.8660254037844387076, 1.000000000000000000, 0.8660254037844387076, 1.000000000000000000, 0.8660254037844387076, 1.000000000000000000, 0.8660254037844387076, 1.000000000000000000, 0.8660254037844387076, 1.000000000000000000, 0.8660254037844387076, 1.000000000000000000, 0.8660254037844387076, 1.000000000000000000, 0.8660254037844387076, 1.000000000000000000, 0.8660254037844387076, 1.000000000000000000, 0.8660254037844387076, 1.000000000000000000, 0.8660254037844387076, 1.000000000000000000, 0.8660254037844387076, 1.000000000000000000, 0.8660254037844387076, 1.000000000000000000, 0.8660254037844387076, 1.000000000000000000, 0.8660254037844387076, 1.000000000000000000, 0.8660254037844387076, 1.000000000000000000, 0.8660254037844387076, 1.000000000000000000, 0.8660254037844387076, 1.000000000000000000, 0.8660254037844387076, 1.000000000000000000, 0.8660254037844387076, 1.000000000000000000, 0.9111409417988175496, 0.9401539645359766606) ) ) 
 REPRESENTATION_ITEM ( '' )  SURFACE ( )  );
#6044=CARTESIAN_POINT ( 'NONE',  ( 229.5999999999999375, -33.54374999877096286, -50.00000000000011369 ) ) ;
#6045=CARTESIAN_POINT ( 'NONE',  ( 229.8435696437499871, -30.66562499938547859, 101.5914258081833879 ) ) ;
#6048=CARTESIAN_POINT ( 'NONE',  ( 235.5999999999999375, -33.76874999877096428, 99.99999999999998579 ) ) ;
#6050=DIRECTION ( 'NONE',  ( 1.788378118793198438E-31, 3.597944987211154374E-15, 1.000000000000000000 ) ) ;
#6051=CARTESIAN_POINT ( 'NONE',  ( 232.5999999999999375, -29.99999999999999645, 103.0000000000000000 ) ) ;
#6053=CARTESIAN_POINT ( 'NONE',  ( 234.0999999999999375, -32.39999999999999858, 97.40192378864668399 ) ) ;
#6055=CARTESIAN_POINT ( 'NONE',  ( 229.8435696437499303, -34.30312499938548143, -50.00000000000011369 ) ) ;
#6058=CARTESIAN_POINT ( 'NONE',  ( 229.8435696437499871, -30.74062499938547433, 98.40857419181659793 ) ) ;
#6059=CARTESIAN_POINT ( 'NONE',  ( 229.5999999999999375, -33.13124999877096144, -51.73205080756898866 ) ) ;
#6063=LINE ( 'NONE', #18268, #16320 ) ;
#6068=CARTESIAN_POINT ( 'NONE',  ( 234.0999999999999375, -32.39999999999999858, 97.40192378864668399 ) ) ;
#6071=( BOUNDED_CURVE ( )  B_SPLINE_CURVE ( 2, ( #5847, #17861, #11800, #11698, #17769, #4472, #5569, #10243, #14817 ),
 .UNSPECIFIED., .F., .F. ) 
 B_SPLINE_CURVE_WITH_KNOTS ( ( 3, 2, 2, 2, 3 ),
 ( 0.6458333333333332593, 0.6527777777777777901, 0.6666666666666666297, 0.6805555555555555802, 0.6875000000000000000 ),
 .UNSPECIFIED. ) 
 CURVE ( )  GEOMETRIC_REPRESENTATION_ITEM ( )  RATIONAL_B_SPLINE_CURVE ( ( 0.9330127018922192983, 0.9330127018922187432, 1.000000000000000000, 0.8660254037844387076, 1.000000000000000000, 0.8660254037844387076, 1.000000000000000000, 0.9330127018922194093, 0.9330127018922194093 ) ) 
 REPRESENTATION_ITEM ( '' )  );
#6072=EDGE_CURVE ( 'NONE', #5766, #15452, #14239, .T. ) ;
#6074=CYLINDRICAL_SURFACE ( 'NONE', #9761, 2.200000000000007283 ) ;
#6078=CARTESIAN_POINT ( 'NONE',  ( 229.8435696437499871, -31.07812499938548001, 98.40857419181659793 ) ) ;
#6082=CARTESIAN_POINT ( 'NONE',  ( 235.5999999999999943, -32.43749999999999289, -51.73205080756900287 ) ) ;
#6083=CARTESIAN_POINT ( 'NONE',  ( 234.0999999999999375, -34.59374999877096002, -52.59807621135342970 ) ) ;
#6087=CARTESIAN_POINT ( 'NONE',  ( 232.5999999999999375, -31.82812499938547290, -46.81714838363331666 ) ) ;
#6089=ORIENTED_EDGE ( 'NONE', *, *, #16819, .T. ) ;
#6095=CARTESIAN_POINT ( 'NONE',  ( 235.3564303562499447, -34.82812499938548001, 98.40857419181659793 ) ) ;
#6096=CARTESIAN_POINT ( 'NONE',  ( 235.3564303562499447, -34.37812499938547717, -51.59142580818350154 ) ) ;
#6101=CARTESIAN_POINT ( 'NONE',  ( 231.0999999999999375, -33.22499999999999432, -52.59807621135342970 ) ) ;
#6103=( BOUNDED_SURFACE ( )  B_SPLINE_SURFACE ( 1, 2, ( 
 ( #1296, #11644, #8804, #19267, #17605, #17800, #2942, #16429, #14761, #12024, #10176, #7438, #14958, #14661, #7243, #7339, #10368, #19171, #8895, #7531, #1197, #5885, #16333, #8609, #128, #6078, #14558, #13395, #28, #4707, #4899, #4609, #16816, #10565, #15249, #15148, #12127, #6365, #16528, #16621, #18098, #3226, #3129, #417, #12218, #9375, #7627, #3425, #9088, #15052, #9185, #1675, #1862, #13581, #221, #6175, #10654, #1766, #7725, #9282, #13682, #325, #6273, #18187, #4809, #10750, #16714, #3321, #12316, #13777, #10844, #7822, #18283, #14065, #6655, #794, #3802, #700, #5287, #9676, #6458, #12411, #5184, #2155, #7820, #18472, #10843, #17099, #12315, #9573, #10941, #18671, #3710, #4898, #2242, #13968, #608, #16908, #13864, #5000, #18282, #11234, #5092, #16815, #3517, #12600, #18380, #17197, #14160, #6363, #8210, #17000, #18570, #6751, #6557, #506, #3612, #15540, #8112, #12502, #9475, #1861, #1955, #15439, #11131, #15637, #11036, #12696, #2050, #416, #15248, #13775, #3424, #9374, #15339, #7915, #8009 ),
 ( #2441, #16116, #14254, #5385, #2725, #12796, #12986, #10061, #16019, #3901, #891, #6851, #15732, #8396, #1074, #14349, #8687, #6941, #5672, #17296, #2621, #4004, #17678, #4097, #11429, #19049, #8583, #14637, #13174, #11527, #17582, #14537, #12891, #15829, #985, #4193, #9770, #14441, #7129, #18862, #18763, #5483, #17392, #1271, #11615, #9969, #11331, #7218, #1172, #9867, #15923, #2526, #7032, #8486, #13081, #18957, #10155, #19144, #5580, #5760, #17490, #11711, #2339, #8301, #6053, #1652, #3202, #13373, #14936, #4681, #6, #7604, #4389, #9161, #14830, #13269, #3011, #13465, #7313, #12000, #16504, #12098, #4484, #6245, #19242, #9065, #18070, #16311, #1457, #8970, #17969, #17781, #3107, #16596, #14733, #7411, #5955, #16219, #7698, #6146, #12192, #10345, #11904, #17875, #15125, #4293, #13655, #10257, #15030, #10437, #2919, #10631, #2824, #16403, #8872, #1561, #297, #13555, #7508, #1740, #1368, #8780, #5860, #103, #11813, #4581, #10538, #197, #14041, #8089, #5067, #11106, #18259, #6723, #14134, #15514, #2131 ) ),
 .UNSPECIFIED., .F., .F., .F. ) 
 B_SPLINE_SURFACE_WITH_KNOTS ( ( 2, 2 ),
 ( 3, 2, 2, 2, 2, 2, 2, 2, 2, 2, 2, 2, 2, 2, 2, 2, 2, 2, 2, 2, 2, 2, 2, 2, 2, 2, 2, 2, 2, 2, 2, 2, 2, 2, 2, 2, 2, 2, 2, 2, 2, 2, 2, 2, 2, 2, 2, 2, 2, 2, 2, 2, 2, 2, 2, 2, 2, 2, 2, 2, 2, 2, 2, 2, 2, 2, 2, 2, 3 ),
 ( 0.000000000000000000, 1.000000000000000000 ),
 ( 0.000000000000000000, 0.01388888888888888812, 0.02777777777777777624, 0.04166666666666666435, 0.05555555555555555247, 0.06944444444444444753, 0.08333333333333332871, 0.09722222222222222376, 0.1111111111111111049, 0.1250000000000000000, 0.1388888888888888951, 0.1527777777777777901, 0.1666666666666666574, 0.1805555555555555525, 0.1944444444444444475, 0.2083333333333333426, 0.2222222222222222099, 0.2361111111111111049, 0.2500000000000000000, 0.2638888888888888951, 0.2777777777777777901, 0.2916666666666666852, 0.3055555555555555802, 0.3194444444444444198, 0.3333333333333333148, 0.3472222222222222099, 0.3611111111111111049, 0.3750000000000000000, 0.3888888888888888951, 0.4027777777777777901, 0.4166666666666666852, 0.4305555555555555802, 0.4444444444444444198, 0.4583333333333333148, 0.4722222222222222099, 0.4861111111111111049, 0.5000000000000000000, 0.5138888888888888395, 0.5277777777777777901, 0.5416666666666666297, 0.5555555555555555802, 0.5694444444444444198, 0.5833333333333333703, 0.5972222222222222099, 0.6111111111111111605, 0.6250000000000000000, 0.6388888888888888395, 0.6527777777777777901, 0.6666666666666666297, 0.6805555555555555802, 0.6944444444444444198, 0.7083333333333333703, 0.7222222222222222099, 0.7361111111111111605, 0.7500000000000000000, 0.7638888888888888395, 0.7777777777777777901, 0.7916666666666666297, 0.8055555555555555802, 0.8194444444444444198, 0.8333333333333333703, 0.8472222222222222099, 0.8611111111111111605, 0.8750000000000000000, 0.8888888888888888395, 0.9027777777777777901, 0.9166666666666666297, 0.9258785066912882389, 0.9351372917582011501 ),
 .UNSPECIFIED. ) 
 GEOMETRIC_REPRESENTATION_ITEM ( )  RATIONAL_B_SPLINE_SURFACE ( (
 ( 1.000000000000000000, 0.8660254037844387076, 1.000000000000000000, 0.8660254037844387076, 1.000000000000000000, 0.8660254037844387076, 1.000000000000000000, 0.8660254037844387076, 1.000000000000000000, 0.8660254037844387076, 1.000000000000000000, 0.8660254037844387076, 1.000000000000000000, 0.8660254037844387076, 1.000000000000000000, 0.8660254037844387076, 1.000000000000000000, 0.8660254037844387076, 1.000000000000000000, 0.8660254037844387076, 1.000000000000000000, 0.8660254037844387076, 1.000000000000000000, 0.8660254037844387076, 1.000000000000000000, 0.8660254037844387076, 1.000000000000000000, 0.8660254037844387076, 1.000000000000000000, 0.8660254037844387076, 1.000000000000000000, 0.8660254037844387076, 1.000000000000000000, 0.8660254037844387076, 1.000000000000000000, 0.8660254037844387076, 1.000000000000000000, 0.8660254037844387076, 1.000000000000000000, 0.8660254037844387076, 1.000000000000000000, 0.8660254037844387076, 1.000000000000000000, 0.8660254037844387076, 1.000000000000000000, 0.8660254037844387076, 1.000000000000000000, 0.8660254037844387076, 1.000000000000000000, 0.8660254037844387076, 1.000000000000000000, 0.8660254037844387076, 1.000000000000000000, 0.8660254037844387076, 1.000000000000000000, 0.8660254037844387076, 1.000000000000000000, 0.8660254037844387076, 1.000000000000000000, 0.8660254037844387076, 1.000000000000000000, 0.8660254037844387076, 1.000000000000000000, 0.8660254037844387076, 1.000000000000000000, 0.8660254037844387076, 1.000000000000000000, 0.8660254037844387076, 1.000000000000000000, 0.8660254037844387076, 1.000000000000000000, 0.8660254037844387076, 1.000000000000000000, 0.8660254037844387076, 1.000000000000000000, 0.8660254037844387076, 1.000000000000000000, 0.8660254037844387076, 1.000000000000000000, 0.8660254037844387076, 1.000000000000000000, 0.8660254037844387076, 1.000000000000000000, 0.8660254037844387076, 1.000000000000000000, 0.8660254037844387076, 1.000000000000000000, 0.8660254037844387076, 1.000000000000000000, 0.8660254037844387076, 1.000000000000000000, 0.8660254037844387076, 1.000000000000000000, 0.8660254037844387076, 1.000000000000000000, 0.8660254037844387076, 1.000000000000000000, 0.8660254037844387076, 1.000000000000000000, 0.8660254037844387076, 1.000000000000000000, 0.8660254037844387076, 1.000000000000000000, 0.8660254037844387076, 1.000000000000000000, 0.8660254037844387076, 1.000000000000000000, 0.8660254037844387076, 1.000000000000000000, 0.8660254037844387076, 1.000000000000000000, 0.8660254037844387076, 1.000000000000000000, 0.8660254037844387076, 1.000000000000000000, 0.8660254037844387076, 1.000000000000000000, 0.8660254037844387076, 1.000000000000000000, 0.8660254037844387076, 1.000000000000000000, 0.8660254037844387076, 1.000000000000000000, 0.8660254037844387076, 1.000000000000000000, 0.8660254037844387076, 1.000000000000000000, 0.8660254037844387076, 1.000000000000000000, 0.8660254037844387076, 1.000000000000000000, 0.8660254037844387076, 1.000000000000000000, 0.9111410165655264848, 0.9401539157124900736, 0.9401539157124900736, 0.9401539157124900736),
 ( 1.000000000000000000, 0.8660254037844387076, 1.000000000000000000, 0.8660254037844387076, 1.000000000000000000, 0.8660254037844387076, 1.000000000000000000, 0.8660254037844387076, 1.000000000000000000, 0.8660254037844387076, 1.000000000000000000, 0.8660254037844387076, 1.000000000000000000, 0.8660254037844387076, 1.000000000000000000, 0.8660254037844387076, 1.000000000000000000, 0.8660254037844387076, 1.000000000000000000, 0.8660254037844387076, 1.000000000000000000, 0.8660254037844387076, 1.000000000000000000, 0.8660254037844387076, 1.000000000000000000, 0.8660254037844387076, 1.000000000000000000, 0.8660254037844387076, 1.000000000000000000, 0.8660254037844387076, 1.000000000000000000, 0.8660254037844387076, 1.000000000000000000, 0.8660254037844387076, 1.000000000000000000, 0.8660254037844387076, 1.000000000000000000, 0.8660254037844387076, 1.000000000000000000, 0.8660254037844387076, 1.000000000000000000, 0.8660254037844387076, 1.000000000000000000, 0.8660254037844387076, 1.000000000000000000, 0.8660254037844387076, 1.000000000000000000, 0.8660254037844387076, 1.000000000000000000, 0.8660254037844387076, 1.000000000000000000, 0.8660254037844387076, 1.000000000000000000, 0.8660254037844387076, 1.000000000000000000, 0.8660254037844387076, 1.000000000000000000, 0.8660254037844387076, 1.000000000000000000, 0.8660254037844387076, 1.000000000000000000, 0.8660254037844387076, 1.000000000000000000, 0.8660254037844387076, 1.000000000000000000, 0.8660254037844387076, 1.000000000000000000, 0.8660254037844387076, 1.000000000000000000, 0.8660254037844387076, 1.000000000000000000, 0.8660254037844387076, 1.000000000000000000, 0.8660254037844387076, 1.000000000000000000, 0.8660254037844387076, 1.000000000000000000, 0.8660254037844387076, 1.000000000000000000, 0.8660254037844387076, 1.000000000000000000, 0.8660254037844387076, 1.000000000000000000, 0.8660254037844387076, 1.000000000000000000, 0.8660254037844387076, 1.000000000000000000, 0.8660254037844387076, 1.000000000000000000, 0.8660254037844387076, 1.000000000000000000, 0.8660254037844387076, 1.000000000000000000, 0.8660254037844387076, 1.000000000000000000, 0.8660254037844387076, 1.000000000000000000, 0.8660254037844387076, 1.000000000000000000, 0.8660254037844387076, 1.000000000000000000, 0.8660254037844387076, 1.000000000000000000, 0.8660254037844387076, 1.000000000000000000, 0.8660254037844387076, 1.000000000000000000, 0.8660254037844387076, 1.000000000000000000, 0.8660254037844387076, 1.000000000000000000, 0.8660254037844387076, 1.000000000000000000, 0.8660254037844387076, 1.000000000000000000, 0.8660254037844387076, 1.000000000000000000, 0.8660254037844387076, 1.000000000000000000, 0.8660254037844387076, 1.000000000000000000, 0.8660254037844387076, 1.000000000000000000, 0.8660254037844387076, 1.000000000000000000, 0.8660254037844387076, 1.000000000000000000, 0.8660254037844387076, 1.000000000000000000, 0.8660254037844387076, 1.000000000000000000, 0.8660254037844387076, 1.000000000000000000, 0.9111410165655264848, 0.9401539157124900736, 0.9401539157124900736, 0.9401539157124900736) ) ) 
 REPRESENTATION_ITEM ( '' )  SURFACE ( )  );
#6106=CARTESIAN_POINT ( 'NONE',  ( 235.3564303562499447, -30.51562499938548001, -48.40857419181671162 ) ) ;
#6111=FACE_OUTER_BOUND ( 'NONE', #11719, .T. ) ;
#6115=CARTESIAN_POINT ( 'NONE',  ( 244.7999999999999545, -5.000000000000000888, -103.0000000000000995 ) ) ;
#6119=LINE ( 'NONE', #11784, #17716 ) ;
#6129=DIRECTION ( 'NONE',  ( -0.000000000000000000, -1.000000000000000000, -0.000000000000000000 ) ) ;
#6132=EDGE_CURVE ( 'NONE', #804, #2622, #11513, .T. ) ;
#6138=CARTESIAN_POINT ( 'NONE',  ( 231.2217848218749339, -31.07812499938548001, 102.3871387122750889 ) ) ;
#6143=FACE_OUTER_BOUND ( 'NONE', #16668, .T. ) ;
#6146=CARTESIAN_POINT ( 'NONE',  ( 232.5999999999999375, -33.71249999999999147, 96.53589838486223584 ) ) ;
#6149=CARTESIAN_POINT ( 'NONE',  ( 235.3564303562499447, -32.24062499938548143, -51.59142580818350154 ) ) ;
#6151=CARTESIAN_POINT ( 'NONE',  ( 232.5999999999999375, -31.26562499938548356, 96.81714838363319586 ) ) ;
#6153=CARTESIAN_POINT ( 'NONE',  ( 233.9782151781249411, -30.40312499938547930, -52.38713871227520968 ) ) ;
#6160=( BOUNDED_CURVE ( )  B_SPLINE_CURVE ( 2, ( #764, #11205, #4168, #2307, #8457, #8271, #9835, #5456, #6717 ),
 .UNSPECIFIED., .F., .F. ) 
 B_SPLINE_CURVE_WITH_KNOTS ( ( 3, 2, 2, 2, 3 ),
 ( 0.5208333333333333703, 0.5277777777777777901, 0.5416666666666666297, 0.5555555555555555802, 0.5625000000000002220 ),
 .UNSPECIFIED. ) 
 CURVE ( )  GEOMETRIC_REPRESENTATION_ITEM ( )  RATIONAL_B_SPLINE_CURVE ( ( 0.9330127018922192983, 0.9330127018922198534, 1.000000000000000000, 0.8660254037844387076, 1.000000000000000000, 0.8660254037844387076, 1.000000000000000000, 0.9330127018922171889, 0.9330127018922194093 ) ) 
 REPRESENTATION_ITEM ( '' )  );
#6165=CIRCLE ( 'NONE', #4286, 5.200000000000009948 ) ;
#6171=CARTESIAN_POINT ( 'NONE',  ( 229.5999999999999375, -33.63749999999999574, 98.26794919243111792 ) ) ;
#6172=DIRECTION ( 'NONE',  ( -0.000000000000000000, -1.000000000000000000, -0.000000000000000000 ) ) ;
#6175=CARTESIAN_POINT ( 'NONE',  ( 235.3564303562499447, -32.20312499938548001, 101.5914258081833879 ) ) ;
#6180=EDGE_CURVE ( 'NONE', #6661, #19103, #17852, .T. ) ;
#6183=EDGE_CURVE ( 'NONE', #18941, #11625, #14816, .T. ) ;
#6196=CARTESIAN_POINT ( 'NONE',  ( 233.9782151781249411, -33.89062499938548001, 97.61286128772489690 ) ) ;
#6200=VECTOR ( 'NONE', #10716, 1000.000000000000000 ) ;
#6202=ORIENTED_EDGE ( 'NONE', *, *, #13663, .F. ) ;
#6203=CARTESIAN_POINT ( 'NONE',  ( 235.5999999999999375, -33.37499999999999289, -50.00000000000011369 ) ) ;
#6206=CARTESIAN_POINT ( 'NONE',  ( 232.5999999999999091, -32.08124999877096428, -47.00000000000011369 ) ) ;
#6208=CARTESIAN_POINT ( 'NONE',  ( 231.2217848218749339, -33.77812499938547575, -47.61286128772501769 ) ) ;
#6210=ORIENTED_EDGE ( 'NONE', *, *, #13630, .F. ) ;
#6212=CIRCLE ( 'NONE', #7763, 5.200000000000009948 ) ;
#6213=CARTESIAN_POINT ( 'NONE',  ( 235.3564303562499447, -34.37812499938547717, 98.40857419181659793 ) ) ;
#6220=DIRECTION ( 'NONE',  ( -0.000000000000000000, -1.000000000000000000, -0.000000000000000000 ) ) ;
#6221=CARTESIAN_POINT ( 'NONE',  ( 234.0999999999999375, -32.84999999999999432, -52.59807621135342970 ) ) ;
#6224=ORIENTED_EDGE ( 'NONE', *, *, #16768, .F. ) ;
#6230=ORIENTED_EDGE ( 'NONE', *, *, #13934, .F. ) ;
#6235=CARTESIAN_POINT ( 'NONE',  ( 232.5999999999999375, -32.75624999877096144, -53.00000000000010658 ) ) ;
#6236=CARTESIAN_POINT ( 'NONE',  ( 231.2217848218749339, -33.92812499938548143, 97.61286128772489690 ) ) ;
#6238=ORIENTED_EDGE ( 'NONE', *, *, #2545, .F. ) ;
#6239=FACE_OUTER_BOUND ( 'NONE', #3596, .T. ) ;
#6245=CARTESIAN_POINT ( 'NONE',  ( 229.5999999999999375, -33.11249999999999716, 101.7320508075688679 ) ) ;
#6249=CARTESIAN_POINT ( 'NONE',  ( 231.2217848218749339, -33.92812499938548143, -52.38713871227520968 ) ) ;
#6251=CARTESIAN_POINT ( 'NONE',  ( 235.5999999999999943, -34.25624999877096855, 101.7320508075688537 ) ) ;
#6252=CARTESIAN_POINT ( 'NONE',  ( 229.8435696437499871, -30.74062499938547433, -51.59142580818350865 ) ) ;
#6256=CARTESIAN_POINT ( 'NONE',  ( 229.5999999999999375, -32.68124999877096570, -51.73205080756898866 ) ) ;
#6262=CARTESIAN_POINT ( 'NONE',  ( 231.0999999999999375, -34.06874999877096144, 97.40192378864668399 ) ) ;
#6271=DIRECTION ( 'NONE',  ( -0.000000000000000000, -0.000000000000000000, 1.000000000000000000 ) ) ;
#6272=EDGE_CURVE ( 'NONE', #11529, #5414, #7235, .T. ) ;
#6273=CARTESIAN_POINT ( 'NONE',  ( 231.2217848218749339, -32.46562499938547575, 97.61286128772489690 ) ) ;
#6276=DIRECTION ( 'NONE',  ( 0.000000000000000000, 0.000000000000000000, 1.000000000000000000 ) ) ;
#6281=CARTESIAN_POINT ( 'NONE',  ( 231.3449744686915324, -35.00000000000002842, -47.51146709331043638 ) ) ;
#6290=CARTESIAN_POINT ( 'NONE',  ( 229.8435696437499303, -33.74062499938548143, 99.99999999999998579 ) ) ;
#6294=ORIENTED_EDGE ( 'NONE', *, *, #14251, .T. ) ;
#6295=CARTESIAN_POINT ( 'NONE',  ( 229.5999999999999375, -33.14999999999999147, -50.00000000000011369 ) ) ;
#6301=CARTESIAN_POINT ( 'NONE',  ( 232.5999999999999375, -34.19062499938547717, -46.81714838363331666 ) ) ;
#6303=ORIENTED_EDGE ( 'NONE', *, *, #10300, .T. ) ;
#6305=CARTESIAN_POINT ( 'NONE',  ( 105.2000000000000739, -32.00000000000002842, 147.7999999999999829 ) ) ;
#6307=VECTOR ( 'NONE', #1205, 1000.000000000000000 ) ;
#6314=CARTESIAN_POINT ( 'NONE',  ( 232.5999999999999375, -30.70312499938548001, -53.18285161636690361 ) ) ;
#6320=DIRECTION ( 'NONE',  ( 1.000000000000000000, 0.000000000000000000, 0.000000000000000000 ) ) ;
#6332=CARTESIAN_POINT ( 'NONE',  ( 233.9782151781249411, -33.55312499938548143, 97.61286128772489690 ) ) ;
#6339=VECTOR ( 'NONE', #17827, 1000.000000000000000 ) ;
#6343=ORIENTED_EDGE ( 'NONE', *, *, #16183, .T. ) ;
#6344=CARTESIAN_POINT ( 'NONE',  ( 229.8435696437499587, -32.46562499938548285, -48.40857419181671162 ) ) ;
#6345=CARTESIAN_POINT ( 'NONE',  ( 231.2217848218749339, -33.47812499938547859, 97.61286128772489690 ) ) ;
#6346=CARTESIAN_POINT ( 'NONE',  ( 229.8435696437499303, -31.15312499938548285, -50.00000000000011369 ) ) ;
#6350=VECTOR ( 'NONE', #4112, 1000.000000000000000 ) ;
#6354=CLOSED_SHELL ( 'NONE', ( #6749, #1822, #4744, #8034, #18829, #12235, #814, #15320, #3866, #5895, #9215, #7370, #6724, #2200, #1002, #318, #3849, #14658, #14370, #16957, #15924, #15133, #587, #12718, #16400, #6634, #3535, #13764, #7959, #12214, #4012, #11741, #3758, #11062, #17708, #11661, #13242, #18123, #15016, #2674, #5769, #17488, #10444, #14485, #16566, #4722, #4588, #4209, #9849, #5209, #529, #10787, #6729, #7835, #2575, #16518, #17879, #3977, #5943, #8855, #1255, #1593, #1837, #5003, #303, #4387, #17484, #16408, #7802, #15895, #7331, #16275, #5355, #19259, #8436, #3749 ) ) ;
#6363=CARTESIAN_POINT ( 'NONE',  ( 229.8435696437499871, -34.22812499938547148, 98.40857419181659793 ) ) ;
#6364=B_SPLINE_CURVE_WITH_KNOTS ( 'NONE', 3,
 ( #9570, #17097, #3708, #12693, #3420, #13172, #11427, #17388, #5481, #1269 ),
 .UNSPECIFIED., .F., .F.,
 ( 4, 2, 2, 2, 4 ),
 ( 0.3612006186103786654, 0.3925526867148934063, 0.4239047548194081472, 0.4552568229239228881, 0.4866088910284376290 ),
 .UNSPECIFIED. ) ;
#6365=CARTESIAN_POINT ( 'NONE',  ( 229.8435696437499871, -31.52812499938547575, 98.40857419181659793 ) ) ;
#6373=ORIENTED_EDGE ( 'NONE', *, *, #13926, .T. ) ;
#6377=CARTESIAN_POINT ( 'NONE',  ( 235.5999999999999943, -33.33749999999999147, -51.73205080756900287 ) ) ;
#6382=DIRECTION ( 'NONE',  ( -0.000000000000000000, -1.000000000000000000, -0.000000000000000000 ) ) ;
#6387=CARTESIAN_POINT ( 'NONE',  ( 232.5999999999999375, -32.13749999999998863, -46.53589838486234953 ) ) ;
#6392=CARTESIAN_POINT ( 'NONE',  ( 231.2217848218749339, -32.87812499938547717, 102.3871387122750889 ) ) ;
#6394=CARTESIAN_POINT ( 'NONE',  ( 232.5999999999999375, -33.96562499938547575, -53.18285161636690361 ) ) ;
#6395=EDGE_CURVE ( 'NONE', #2004, #18744, #5534, .T. ) ;
#6401=CARTESIAN_POINT ( 'NONE',  ( 230.7186334667984227, -32.00000000000000711, -52.01453922190813728 ) ) ;
#6407=CARTESIAN_POINT ( 'NONE',  ( 235.5999999999999375, -32.92499999999999716, -50.00000000000011369 ) ) ;
#6416=ORIENTED_EDGE ( 'NONE', *, *, #4540, .T. ) ;
#6422=CARTESIAN_POINT ( 'NONE',  ( 229.5999999999999375, -33.05624999877096570, -48.26794919243123161 ) ) ;
#6423=CARTESIAN_POINT ( 'NONE',  ( 235.3564303562499447, -35.01562499938548001, 101.5914258081833879 ) ) ;
#6428=CARTESIAN_POINT ( 'NONE',  ( 105.1999999999999744, -31.99999999999999289, -100.0000000000000000 ) ) ;
#6437=CARTESIAN_POINT ( 'NONE',  ( 233.9782151781249411, -32.80312499938548143, -47.61286128772501769 ) ) ;
#6439=CARTESIAN_POINT ( 'NONE',  ( 235.3564303562499447, -31.82812499938547646, 99.99999999999998579 ) ) ;
#6440=CARTESIAN_POINT ( 'NONE',  ( 232.5999999999999375, -31.04062499938547859, -46.81714838363331666 ) ) ;
#6449=EDGE_LOOP ( 'NONE', ( #2140, #994, #2516, #4904 ) ) ;
#6456=CARTESIAN_POINT ( 'NONE',  ( 235.5999999999999375, -32.41874999877096286, 99.99999999999998579 ) ) ;
#6458=CARTESIAN_POINT ( 'NONE',  ( 233.9782151781249411, -33.14062499938548001, 102.3871387122750889 ) ) ;
#6460=CARTESIAN_POINT ( 'NONE',  ( 231.0999999999999375, -30.91874999877096286, 97.40192378864668399 ) ) ;
#6462=EDGE_LOOP ( 'NONE', ( #12193, #10512, #15866, #9856 ) ) ;
#6465=VECTOR ( 'NONE', #9875, 1000.000000000000000 ) ;
#6469=CARTESIAN_POINT ( 'NONE',  ( 229.5999999999999375, -33.54374999877096286, 99.99999999999998579 ) ) ;
#6471=EDGE_LOOP ( 'NONE', ( #17015, #13132, #850, #11070 ) ) ;
#6475=VECTOR ( 'NONE', #11498, 1000.000000000000000 ) ;
#6485=CARTESIAN_POINT ( 'NONE',  ( 229.5999999999999375, -33.18749999999999289, -51.73205080756898866 ) ) ;
#6489=EDGE_CURVE ( 'NONE', #6967, #15345, #2116, .T. ) ;
#6491=CARTESIAN_POINT ( 'NONE',  ( 231.2217848218749339, -32.42812499938548143, 102.3871387122750889 ) ) ;
#6493=CARTESIAN_POINT ( 'NONE',  ( 233.9782151781249411, -33.25312499938547717, -47.61286128772501769 ) ) ;
#6498=CARTESIAN_POINT ( 'NONE',  ( 233.4038475772933054, -33.73259618943232852, -53.00000000000010658 ) ) ;
#6510=CARTESIAN_POINT ( 'NONE',  ( 231.2217848218749339, -31.11562499938547788, -52.38713871227520968 ) ) ;
#6515=CARTESIAN_POINT ( 'NONE',  ( 229.5999999999999375, -32.24999999999999289, 99.99999999999998579 ) ) ;
#6519=CARTESIAN_POINT ( 'NONE',  ( 232.5999999999999659, -32.13749999999999574, -47.00000000000011369 ) ) ;
#6525=CARTESIAN_POINT ( 'NONE',  ( 233.9782151781249411, -34.00312499938547717, 97.61286128772489690 ) ) ;
#6527=ORIENTED_EDGE ( 'NONE', *, *, #14610, .F. ) ;
#6532=DIRECTION ( 'NONE',  ( 0.000000000000000000, 0.000000000000000000, -1.000000000000000000 ) ) ;
#6535=ORIENTED_EDGE ( 'NONE', *, *, #12971, .T. ) ;
#6536=CARTESIAN_POINT ( 'NONE',  ( 229.8435696437499303, -34.75312499938547717, -50.00000000000011369 ) ) ;
#6537=CARTESIAN_POINT ( 'NONE',  ( 232.5999999999999375, -31.71562499938547930, 96.81714838363319586 ) ) ;
#6538=CARTESIAN_POINT ( 'NONE',  ( 232.5999999999999375, -31.71562499938547930, -53.18285161636690361 ) ) ;
#6542=EDGE_CURVE ( 'NONE', #6661, #12219, #8171, .T. ) ;
#6556=CARTESIAN_POINT ( 'NONE',  ( 232.5999999999999375, -33.48749999999999716, 103.0000000000000000 ) ) ;
#6557=CARTESIAN_POINT ( 'NONE',  ( 235.3564303562499447, -34.41562499938547859, 99.99999999999998579 ) ) ;
#6563=DIRECTION ( 'NONE',  ( 0.000000000000000000, -1.000000000000000000, 3.597944987211154374E-15 ) ) ;
#6566=CARTESIAN_POINT ( 'NONE',  ( 231.2217848218749339, -34.26562499938548001, -52.38713871227520968 ) ) ;
#6567=CARTESIAN_POINT ( 'NONE',  ( 235.5999999999999943, -33.80624999877096570, -48.26794919243124582 ) ) ;
#6568=ORIENTED_EDGE ( 'NONE', *, *, #10099, .T. ) ;
#6569=CARTESIAN_POINT ( 'NONE',  ( 235.5999999999999943, -33.41249999999999432, -48.26794919243124582 ) ) ;
#6575=CARTESIAN_POINT ( 'NONE',  ( 232.5999999999999375, -29.99999999999999645, -53.00000000000012079 ) ) ;
#6580=( BOUNDED_CURVE ( )  B_SPLINE_CURVE ( 2, ( #14460, #14181, #6961, #12621, #3924, #2264, #4120, #2546, #15945 ),
 .UNSPECIFIED., .F., .F. ) 
 B_SPLINE_CURVE_WITH_KNOTS ( ( 3, 2, 2, 2, 3 ),
 ( 0.3125000000000000555, 0.3194444444444444198, 0.3333333333333333148, 0.3472222222222222099, 0.3541666666666666852 ),
 .UNSPECIFIED. ) 
 CURVE ( )  GEOMETRIC_REPRESENTATION_ITEM ( )  RATIONAL_B_SPLINE_CURVE ( ( 0.9330127018922192983, 0.9330127018922198534, 1.000000000000000000, 0.8660254037844387076, 1.000000000000000000, 0.8660254037844387076, 1.000000000000000000, 0.9330127018922190762, 0.9330127018922194093 ) ) 
 REPRESENTATION_ITEM ( '' )  );
#6582=EDGE_LOOP ( 'NONE', ( #7515, #6831, #7449, #4622 ) ) ;
#6586=CARTESIAN_POINT ( 'NONE',  ( 235.3564303562499447, -32.76562499938548001, 101.5914258081833879 ) ) ;
#6588=CARTESIAN_POINT ( 'NONE',  ( 235.3564303562499447, -34.07812499938548001, -50.00000000000011369 ) ) ;
#6593=DIRECTION ( 'NONE',  ( -0.000000000000000000, -1.000000000000000000, -0.000000000000000000 ) ) ;
#6603=EDGE_LOOP ( 'NONE', ( #6373, #11688, #306 ) ) ;
#6615=DIRECTION ( 'NONE',  ( -1.000000000000000000, 0.000000000000000000, -0.000000000000000000 ) ) ;
#6617=CARTESIAN_POINT ( 'NONE',  ( 229.8435696437499871, -34.26562499938548001, 101.5914258081833879 ) ) ;
#6620=CARTESIAN_POINT ( 'NONE',  ( 229.5999999999999375, -32.66249999999999432, 101.7320508075688821 ) ) ;
#6631=SHAPE_DEFINITION_REPRESENTATION ( #15920, #4499 ) ;
#6632=CARTESIAN_POINT ( 'NONE',  ( 232.5999999999999375, -33.29062499938547859, 103.1828516163667899 ) ) ;
#6633=CARTESIAN_POINT ( 'NONE',  ( 231.2217848218749339, -33.47812499938547859, -52.38713871227520968 ) ) ;
#6634=ADVANCED_FACE ( 'NONE', ( #5636 ), #15984, .F. ) ;
#6636=CARTESIAN_POINT ( 'NONE',  ( 234.0999999999999375, -34.79999999999999716, -47.40192378864679768 ) ) ;
#6637=VERTEX_POINT ( 'NONE', #14694 ) ;
#6640=EDGE_CURVE ( 'NONE', #138, #15818, #14760, .T. ) ;
#6655=CARTESIAN_POINT ( 'NONE',  ( 231.2217848218749339, -32.91562499938547148, 97.61286128772489690 ) ) ;
#6661=VERTEX_POINT ( 'NONE', #6305 ) ;
#6663=DIRECTION ( 'NONE',  ( 0.000000000000000000, -0.000000000000000000, -1.000000000000000000 ) ) ;
#6664=CARTESIAN_POINT ( 'NONE',  ( 105.1999999999999886, -4.999999999999993783, -103.0000000000000995 ) ) ;
#6669=( BOUNDED_CURVE ( )  B_SPLINE_CURVE ( 2, ( #3521, #9578, #2159, #12320, #17006, #5005, #8012, #15151, #18576 ),
 .UNSPECIFIED., .F., .F. ) 
 B_SPLINE_CURVE_WITH_KNOTS ( ( 3, 2, 2, 2, 3 ),
 ( 0.3125000000000000555, 0.3194444444444444198, 0.3333333333333333148, 0.3472222222222222099, 0.3541666666666666852 ),
 .UNSPECIFIED. ) 
 CURVE ( )  GEOMETRIC_REPRESENTATION_ITEM ( )  RATIONAL_B_SPLINE_CURVE ( ( 0.9330127018922192983, 0.9330127018922198534, 1.000000000000000000, 0.8660254037844387076, 1.000000000000000000, 0.8660254037844387076, 1.000000000000000000, 0.9330127018922190762, 0.9330127018922194093 ) ) 
 REPRESENTATION_ITEM ( '' )  );
#6677=CARTESIAN_POINT ( 'NONE',  ( 232.3466685930879123, -34.99995246259152282, -52.98928446312130802 ) ) ;
#6678=LINE ( 'NONE', #6575, #5085 ) ;
#6683=CARTESIAN_POINT ( 'NONE',  ( 229.5999999999999375, -34.49999999999999289, -50.00000000000011369 ) ) ;
#6688=CARTESIAN_POINT ( 'NONE',  ( 232.5999999999999375, -31.37812499938547717, -46.81714838363331666 ) ) ;
#6697=LINE ( 'NONE', #4845, #9545 ) ;
#6700=CARTESIAN_POINT ( 'NONE',  ( 233.9782151781249411, -32.09062499938547575, -52.38713871227520968 ) ) ;
#6709=VERTEX_POINT ( 'NONE', #16465 ) ;
#6711=DIRECTION ( 'NONE',  ( -4.415659757031858318E-14, 1.577021341797092166E-14, 1.000000000000000000 ) ) ;
#6714=CARTESIAN_POINT ( 'NONE',  ( 229.8435696437499871, -31.07812499938548001, 98.40857419181659793 ) ) ;
#6717=CARTESIAN_POINT ( 'NONE',  ( 232.5999999999999091, -33.03749999999998721, 102.9999999999999858 ) ) ;
#6720=CARTESIAN_POINT ( 'NONE',  ( 249.9999999999999716, -35.00000000000000000, -100.0000000000000000 ) ) ;
#6721=CARTESIAN_POINT ( 'NONE',  ( 229.5999999999999375, -34.93124999877095860, -51.73205080756898866 ) ) ;
#6723=CARTESIAN_POINT ( 'NONE',  ( 229.5999999999999659, -34.97364041986482874, 98.90809577818232867 ) ) ;
#6724=ADVANCED_FACE ( 'NONE', ( #6111 ), #12061, .F. ) ;
#6726=CARTESIAN_POINT ( 'NONE',  ( 232.5999999999999943, -34.86562499938548143, -53.18285161636690361 ) ) ;
#6727=CARTESIAN_POINT ( 'NONE',  ( 233.9782151781249411, -32.20312499938548001, 97.61286128772489690 ) ) ;
#6728=CARTESIAN_POINT ( 'NONE',  ( 231.2217848218749339, -31.97812499938548214, -47.61286128772501769 ) ) ;
#6729=ADVANCED_FACE ( 'NONE', ( #5226 ), #18709, .T. ) ;
#6737=CYLINDRICAL_SURFACE ( 'NONE', #4748, 3.000000000000009770 ) ;
#6745=CARTESIAN_POINT ( 'NONE',  ( 244.7999999999999545, -32.00000000000000711, -97.80000000000002558 ) ) ;
#6746=EDGE_CURVE ( 'NONE', #15232, #11798, #16759, .T. ) ;
#6749=ADVANCED_FACE ( 'NONE', ( #6794 ), #13810, .F. ) ;
#6750=CARTESIAN_POINT ( 'NONE',  ( 233.5451393107506135, -32.00000000000000711, 102.7533691519571164 ) ) ;
#6751=CARTESIAN_POINT ( 'NONE',  ( 235.3564303562499447, -34.37812499938547717, 98.40857419181659793 ) ) ;
#6756=CARTESIAN_POINT ( 'NONE',  ( 235.5999999999999375, -31.51874999877096073, 99.99999999999998579 ) ) ;
#6760=CARTESIAN_POINT ( 'NONE',  ( 229.5999999999999375, -32.60624999877096286, 101.7320508075688821 ) ) ;
#6765=DIRECTION ( 'NONE',  ( 4.625929269271485174E-17, 1.000000000000000000, -0.000000000000000000 ) ) ;
#6767=CARTESIAN_POINT ( 'NONE',  ( 249.9999999999999716, -29.80000000000000426, -100.0000000000000000 ) ) ;
#6781=CARTESIAN_POINT ( 'NONE',  ( 235.5999999999999943, -34.68749999999999289, -51.73205080756900287 ) ) ;
#6783=CARTESIAN_POINT ( 'NONE',  ( 234.0999999999999375, -33.24374999877096570, -52.59807621135342970 ) ) ;
#6784=B_SPLINE_CURVE_WITH_KNOTS ( 'NONE', 3,
 ( #13527, #1710, #7665, #10506, #19316, #13721, #17754, #13621, #14903, #16473, #3078, #9038, #15003, #2889, #8845, #165, #16752, #11181 ),
 .UNSPECIFIED., .F., .F.,
 ( 4, 2, 2, 2, 2, 2, 2, 2, 4 ),
 ( 0.000000000000000000, 0.0007089252359871075744, 0.001417850471974215149, 0.002126775707961322832, 0.002835700943948430298, 0.003544626179935537764, 0.004253551415922645663, 0.004962476651909753129, 0.005671401887896860596 ),
 .UNSPECIFIED. ) ;
#6786=CARTESIAN_POINT ( 'NONE',  ( 233.9782151781249411, -32.65312499938548285, 97.61286128772489690 ) ) ;
#6788=CARTESIAN_POINT ( 'NONE',  ( 235.3564303562499447, -30.32812499938548001, -51.59142580818350865 ) ) ;
#6794=FACE_OUTER_BOUND ( 'NONE', #2629, .T. ) ;
#6797=CARTESIAN_POINT ( 'NONE',  ( 231.0999999999999375, -33.01874999877096428, -47.40192378864679768 ) ) ;
#6798=CARTESIAN_POINT ( 'NONE',  ( 229.8435696437499587, -32.42812499938548143, -51.59142580818350154 ) ) ;
#6804=CARTESIAN_POINT ( 'NONE',  ( 231.2217848218749339, -33.21562499938547575, -47.61286128772501769 ) ) ;
#6815=AXIS2_PLACEMENT_3D ( 'NONE', #18017, #9106, #16730 ) ;
#6831=ORIENTED_EDGE ( 'NONE', *, *, #4115, .T. ) ;
#6832=CARTESIAN_POINT ( 'NONE',  ( 229.8435696437499587, -34.71562499938547575, -48.40857419181671162 ) ) ;
#6834=CARTESIAN_POINT ( 'NONE',  ( 233.7151113960924818, -35.00000000000002842, -47.47285052570518360 ) ) ;
#6835=CARTESIAN_POINT ( 'NONE',  ( 231.2217848218749339, -33.02812499938547575, -52.38713871227520968 ) ) ;
#6838=ORIENTED_EDGE ( 'NONE', *, *, #19299, .T. ) ;
#6849=CARTESIAN_POINT ( 'NONE',  ( 234.4730806518346924, -35.00000000000001421, 102.0537355158135568 ) ) ;
#6850=CARTESIAN_POINT ( 'NONE',  ( 231.9083760470965103, -32.00000000000000711, 102.7516965079134081 ) ) ;
#6851=CARTESIAN_POINT ( 'NONE',  ( 229.5999999999999375, -30.41249999999999076, 101.7320508075688679 ) ) ;
#6854=CARTESIAN_POINT ( 'NONE',  ( 234.0999999999999375, -30.99374999877096215, 97.40192378864668399 ) ) ;
#6855=CARTESIAN_POINT ( 'NONE',  ( 231.0999999999999375, -32.11874999877096570, -47.40192378864679768 ) ) ;
#6856=ORIENTED_EDGE ( 'NONE', *, *, #11503, .T. ) ;
#6870=CARTESIAN_POINT ( 'NONE',  ( 233.4038475772933623, -32.32634618820329564, -53.00000000000011369 ) ) ;
#6871=CARTESIAN_POINT ( 'NONE',  ( 233.7735609739809490, -31.99999999999998579, -52.66365949829813786 ) ) ;
#6877=CARTESIAN_POINT ( 'NONE',  ( 232.5999999999999091, -32.08124999877096428, -47.00000000000011369 ) ) ;
#6878=CARTESIAN_POINT ( 'NONE',  ( 235.4063471324517991, -34.99999999999999289, 99.92898555286095075 ) ) ;
#6880=CARTESIAN_POINT ( 'NONE',  ( 233.9782151781249411, -34.60312499938548569, 102.3871387122750889 ) ) ;
#6882=CARTESIAN_POINT ( 'NONE',  ( 229.8435696437499303, -31.49062499938547788, -50.00000000000011369 ) ) ;
#6883=ORIENTED_EDGE ( 'NONE', *, *, #6072, .F. ) ;
#6888=CARTESIAN_POINT ( 'NONE',  ( 244.7999999999999545, -29.80000000000002203, 147.7999999999999829 ) ) ;
#6889=CARTESIAN_POINT ( 'NONE',  ( 231.2217848218749339, -32.46562499938547575, -52.38713871227520968 ) ) ;
#6894=EDGE_CURVE ( 'NONE', #1370, #9344, #18898, .T. ) ;
#6895=CARTESIAN_POINT ( 'NONE',  ( 229.8435696437499303, -32.39062499938548001, -50.00000000000011369 ) ) ;
#6900=CARTESIAN_POINT ( 'NONE',  ( 231.7961524227065695, -32.34240381056765301, 96.99999999999998579 ) ) ;
#6902=( BOUNDED_CURVE ( )  B_SPLINE_CURVE ( 2, ( #9433, #660, #12371, #9332, #7679, #562, #6519 ),
 .UNSPECIFIED., .F., .F. ) 
 B_SPLINE_CURVE_WITH_KNOTS ( ( 3, 2, 2, 3 ),
 ( 0.3702305174531566045, 0.3750000000000000000, 0.3888888888888888951, 0.3958333333333333148 ),
 .UNSPECIFIED. ) 
 CURVE ( )  GEOMETRIC_REPRESENTATION_ITEM ( )  RATIONAL_B_SPLINE_CURVE ( ( 0.9395835397633047759, 0.9539927561173232595, 1.000000000000000000, 0.8660254037844387076, 1.000000000000000000, 0.9330127018922196314, 0.9330127018922194093 ) ) 
 REPRESENTATION_ITEM ( '' )  );
#6909=CARTESIAN_POINT ( 'NONE',  ( 232.5999999999999375, -32.81249999999999289, -53.00000000000011369 ) ) ;
#6913=LINE ( 'NONE', #17359, #2742 ) ;
#6917=CARTESIAN_POINT ( 'NONE',  ( 230.8850348010513471, -31.99999999999999289, 97.81539907810714851 ) ) ;
#6918=CARTESIAN_POINT ( 'NONE',  ( 232.5999999999999375, -32.98124999877095576, -47.00000000000011369 ) ) ;
#6923=CARTESIAN_POINT ( 'NONE',  ( 229.8435696437499871, -33.89062499938548001, 98.40857419181659793 ) ) ;
#6924=CARTESIAN_POINT ( 'NONE',  ( 229.8435696437499303, -33.40312499938547575, -50.00000000000011369 ) ) ;
#6925=CARTESIAN_POINT ( 'NONE',  ( 232.5999999999999091, -34.10624999877096286, 96.99999999999998579 ) ) ;
#6926=CARTESIAN_POINT ( 'NONE',  ( 246.9999999999999716, -35.00000000000000000, -100.0000000000000000 ) ) ;
#6930=VERTEX_POINT ( 'NONE', #2766 ) ;
#6934=CARTESIAN_POINT ( 'NONE',  ( 235.3564303562499447, -30.44062499938548072, 98.40857419181659793 ) ) ;
#6941=CARTESIAN_POINT ( 'NONE',  ( 235.5999999999999943, -30.63749999999999574, 98.26794919243110371 ) ) ;
#6944=CARTESIAN_POINT ( 'NONE',  ( 231.0999999999999375, -33.91874999877096286, 102.5980762113533018 ) ) ;
#6946=EDGE_LOOP ( 'NONE', ( #2390, #8409, #18294, #7255 ) ) ;
#6949=DIRECTION ( 'NONE',  ( 0.000000000000000000, 0.000000000000000000, -1.000000000000000000 ) ) ;
#6961=CARTESIAN_POINT ( 'NONE',  ( 231.0999999999999375, -32.11874999877096570, -47.40192378864679768 ) ) ;
#6967=VERTEX_POINT ( 'NONE', #16056 ) ;
#6968=CARTESIAN_POINT ( 'NONE',  ( 232.5999999999999375, -34.61249999999999716, -53.46410161513786363 ) ) ;
#6972=CARTESIAN_POINT ( 'NONE',  ( 229.8435696437499303, -35.20312499938548001, -50.00000000000011369 ) ) ;
#6985=CARTESIAN_POINT ( 'NONE',  ( 231.2217848218749339, -32.46562499938547575, -52.38713871227520968 ) ) ;
#6989=ORIENTED_EDGE ( 'NONE', *, *, #13471, .F. ) ;
#6991=CARTESIAN_POINT ( 'NONE',  ( 232.5999999999999375, -32.36249999999999716, 97.00000000000000000 ) ) ;
#6995=DIRECTION ( 'NONE',  ( 0.000000000000000000, 0.000000000000000000, 1.000000000000000000 ) ) ;
#6996=CARTESIAN_POINT ( 'NONE',  ( 229.8435696437499587, -32.87812499938547717, 98.40857419181659793 ) ) ;
#7005=CARTESIAN_POINT ( 'NONE',  ( 235.4117376914898045, -31.99999999999999289, 98.95399275611721635 ) ) ;
#7006=DIRECTION ( 'NONE',  ( 0.000000000000000000, 0.000000000000000000, -1.000000000000000000 ) ) ;
#7009=ORIENTED_EDGE ( 'NONE', *, *, #7442, .T. ) ;
#7012=LINE ( 'NONE', #10041, #3658 ) ;
#7014=CARTESIAN_POINT ( 'NONE',  ( 229.8435696437499871, -33.36562499938548143, -48.40857419181671162 ) ) ;
#7017=ORIENTED_EDGE ( 'NONE', *, *, #14847, .T. ) ;
#7025=CARTESIAN_POINT ( 'NONE',  ( 229.8435696437499303, -30.25312499938548072, 99.99999999999998579 ) ) ;
#7030=CARTESIAN_POINT ( 'NONE',  ( 233.2099102960629011, -35.00000000000001421, 102.6939647107543010 ) ) ;
#7032=CARTESIAN_POINT ( 'NONE',  ( 234.0999999999999375, -31.94999999999999218, 97.40192378864668399 ) ) ;
#7034=CYLINDRICAL_SURFACE ( 'NONE', #15365, 5.199999999999996625 ) ;
#7035=CARTESIAN_POINT ( 'NONE',  ( 231.0999999999999375, -33.01874999877096428, 102.5980762113533018 ) ) ;
#7036=CARTESIAN_POINT ( 'NONE',  ( 229.5999999999999375, -30.80624999877096215, -48.26794919243123161 ) ) ;
#7037=CARTESIAN_POINT ( 'NONE',  ( 229.5999999999999375, -34.53749999999999432, 98.26794919243111792 ) ) ;
#7040=ORIENTED_EDGE ( 'NONE', *, *, #8764, .T. ) ;
#7049=CARTESIAN_POINT ( 'NONE',  ( 230.8850348010514892, -31.99999999999999289, -52.18460092189305755 ) ) ;
#7055=EDGE_LOOP ( 'NONE', ( #2733, #15053, #5964, #16151 ) ) ;
#7059=CARTESIAN_POINT ( 'NONE',  ( 235.3564303562499447, -33.59062499938547575, 98.40857419181659793 ) ) ;
#7062=CARTESIAN_POINT ( 'NONE',  ( 233.9782151781249411, -30.44062499938548072, -47.61286128772501769 ) ) ;
#7069=CARTESIAN_POINT ( 'NONE',  ( 235.3564303562499447, -32.61562499938548143, 99.99999999999998579 ) ) ;
#7078=CARTESIAN_POINT ( 'NONE',  ( 229.8435696437499871, -34.22812499938547148, -51.59142580818350865 ) ) ;
#7083=CARTESIAN_POINT ( 'NONE',  ( 233.4038475772933054, -34.12634618820329280, -53.00000000000012790 ) ) ;
#7088=CYLINDRICAL_SURFACE ( 'NONE', #17431, 3.000000000000009770 ) ;
#7091=CARTESIAN_POINT ( 'NONE',  ( 233.9782151781249411, -33.14062499938548001, 102.3871387122750889 ) ) ;
#7094=AXIS2_PLACEMENT_3D ( 'NONE', #16482, #3086, #10328 ) ;
#7101=CARTESIAN_POINT ( 'NONE',  ( 232.5999999999999091, -32.08124999877096428, 102.9999999999999858 ) ) ;
#7105=CARTESIAN_POINT ( 'NONE',  ( 231.7961524227065695, -34.14240381056765017, 96.99999999999998579 ) ) ;
#7108=CARTESIAN_POINT ( 'NONE',  ( 231.2217848218749339, -34.37812499938547717, 97.61286128772489690 ) ) ;
#7109=CARTESIAN_POINT ( 'NONE',  ( 233.9782151781249411, -35.05312499938548143, -47.61286128772501769 ) ) ;
#7119=AXIS2_PLACEMENT_3D ( 'NONE', #15789, #9730, #15694 ) ;
#7129=CARTESIAN_POINT ( 'NONE',  ( 231.0999999999999375, -31.42499999999999361, 97.40192378864668399 ) ) ;
#7134=CARTESIAN_POINT ( 'NONE',  ( 231.0999999999999375, -33.16874999877095576, 97.40192378864668399 ) ) ;
#7138=ORIENTED_EDGE ( 'NONE', *, *, #14831, .F. ) ;
#7140=LINE ( 'NONE', #16412, #12255 ) ;
#7149=LINE ( 'NONE', #9987, #16485 ) ;
#7151=B_SPLINE_CURVE_WITH_KNOTS ( 'NONE', 3,
 ( #9220, #17044, #12262, #15582, #13907, #545, #4941, #1898, #12355, #15283, #15184, #15482, #7860, #18322, #646, #6401 ),
 .UNSPECIFIED., .F., .F.,
 ( 4, 2, 2, 2, 2, 2, 2, 4 ),
 ( 0.000000000000000000, 0.0005391024520904644192, 0.001078204904180928838, 0.002156409808361877192, 0.002695512260452351695, 0.003234614712542825329, 0.003773717164633299398, 0.004312819616723773467 ),
 .UNSPECIFIED. ) ;
#7152=CARTESIAN_POINT ( 'NONE',  ( 232.5999999999999375, -33.26249999999999574, 97.00000000000000000 ) ) ;
#7155=ORIENTED_EDGE ( 'NONE', *, *, #6894, .T. ) ;
#7158=CARTESIAN_POINT ( 'NONE',  ( 232.3466685930879123, -34.99995246259152282, 97.01071553687879145 ) ) ;
#7160=CARTESIAN_POINT ( 'NONE',  ( 232.5999999999999943, -34.64062499938548001, 103.1828516163667899 ) ) ;
#7163=CARTESIAN_POINT ( 'NONE',  ( 235.3564303562499447, -32.16562499938547859, -50.00000000000011369 ) ) ;
#7164=ORIENTED_EDGE ( 'NONE', *, *, #6746, .T. ) ;
#7170=CARTESIAN_POINT ( 'NONE',  ( 233.9782151781249411, -30.29062499938547859, 97.61286128772489690 ) ) ;
#7171=CARTESIAN_POINT ( 'NONE',  ( 233.9782151781249411, -32.69062499938547717, -47.61286128772501769 ) ) ;
#7175=CARTESIAN_POINT ( 'NONE',  ( 229.5999999999999375, -30.41249999999999076, -48.26794919243123161 ) ) ;
#7179=FACE_OUTER_BOUND ( 'NONE', #8186, .T. ) ;
#7180=LINE ( 'NONE', #15975, #10856 ) ;
#7181=CARTESIAN_POINT ( 'NONE',  ( 231.2217848218749339, -31.22812499938547859, -52.38713871227520968 ) ) ;
#7185=CARTESIAN_POINT ( 'NONE',  ( 232.5999999999999943, -32.27812499938547575, 103.1828516163667899 ) ) ;
#7186=CARTESIAN_POINT ( 'NONE',  ( 105.1999999999999602, -35.00000000000000711, -97.80000000000002558 ) ) ;
#7189=CARTESIAN_POINT ( 'NONE',  ( 234.5796347213265278, -32.00000000000000000, -47.80162405160952233 ) ) ;
#7194=CARTESIAN_POINT ( 'NONE',  ( 231.0999999999999375, -34.96874999877096002, 97.40192378864668399 ) ) ;
#7199=CARTESIAN_POINT ( 'NONE',  ( 229.8435696437499303, -34.75312499938547717, 99.99999999999998579 ) ) ;
#7200=CARTESIAN_POINT ( 'NONE',  ( 229.8435696437499303, -34.30312499938548143, -50.00000000000011369 ) ) ;
#7201=DIRECTION ( 'NONE',  ( 0.000000000000000000, 0.000000000000000000, -1.000000000000000000 ) ) ;
#7202=ORIENTED_EDGE ( 'NONE', *, *, #10300, .F. ) ;
#7209=CARTESIAN_POINT ( 'NONE',  ( 231.0999999999999375, -33.61874999877096570, -52.59807621135342970 ) ) ;
#7211=CARTESIAN_POINT ( 'NONE',  ( 232.5999999999999375, -32.39062499938548001, 103.1828516163667899 ) ) ;
#7218=CARTESIAN_POINT ( 'NONE',  ( 229.5999999999999375, -31.76249999999999218, 101.7320508075688679 ) ) ;
#7222=CARTESIAN_POINT ( 'NONE',  ( 235.5999999999999375, -31.96874999877096002, 99.99999999999998579 ) ) ;
#7223=CARTESIAN_POINT ( 'NONE',  ( 234.0999999999999375, -34.14374999877096428, -52.59807621135342970 ) ) ;
#7226=EDGE_LOOP ( 'NONE', ( #3886, #5660, #2633, #7202, #5509 ) ) ;
#7230=DIRECTION ( 'NONE',  ( 1.735459783503185124E-31, 0.000000000000000000, 1.000000000000000000 ) ) ;
#7231=VERTEX_POINT ( 'NONE', #14153 ) ;
#7235=CIRCLE ( 'NONE', #16612, 2.199999999999993516 ) ;
#7240=CARTESIAN_POINT ( 'NONE',  ( 234.5119179762160684, -35.00000000000002132, -52.19519922920401456 ) ) ;
#7243=CARTESIAN_POINT ( 'NONE',  ( 231.2217848218749339, -30.66562499938547859, 97.61286128772489690 ) ) ;
#7246=CARTESIAN_POINT ( 'NONE',  ( 235.5999999999999375, -33.31874999877096144, -50.00000000000011369 ) ) ;
#7248=CARTESIAN_POINT ( 'NONE',  ( 233.4038475772933054, -33.73259618943232852, 96.99999999999998579 ) ) ;
#7253=CARTESIAN_POINT ( 'NONE',  ( 231.2217848218749339, -33.81562499938547717, -52.38713871227520968 ) ) ;
#7254=VERTEX_POINT ( 'NONE', #2520 ) ;
#7255=ORIENTED_EDGE ( 'NONE', *, *, #1016, .F. ) ;
#7261=CARTESIAN_POINT ( 'NONE',  ( 233.9782151781249411, -31.79062499938548214, 102.3871387122750889 ) ) ;
#7263=CARTESIAN_POINT ( 'NONE',  ( 231.2217848218749339, -33.36562499938548143, -52.38713871227520968 ) ) ;
#7267=CARTESIAN_POINT ( 'NONE',  ( 231.0999999999999375, -30.82499999999999574, -47.40192378864679768 ) ) ;
#7268=CARTESIAN_POINT ( 'NONE',  ( 232.5999999999999659, -32.58749999999999858, 103.0000000000000000 ) ) ;
#7270=ORIENTED_EDGE ( 'NONE', *, *, #3489, .T. ) ;
#7272=CARTESIAN_POINT ( 'NONE',  ( 232.5999999999999375, -33.71249999999999147, 96.99999999999998579 ) ) ;
#7278=CARTESIAN_POINT ( 'NONE',  ( 233.9782151781249411, -32.09062499938547575, 97.61286128772489690 ) ) ;
#7285=LINE ( 'NONE', #14412, #18301 ) ;
#7287=LINE ( 'NONE', #13530, #4587 ) ;
#7288=CARTESIAN_POINT ( 'NONE',  ( 232.5999999999999091, -33.03749999999998721, -47.00000000000011369 ) ) ;
#7296=ORIENTED_EDGE ( 'NONE', *, *, #12684, .F. ) ;
#7304=CARTESIAN_POINT ( 'NONE',  ( 229.8435696437499871, -32.01562499938548001, 101.5914258081833879 ) ) ;
#7313=CARTESIAN_POINT ( 'NONE',  ( 235.5999999999999375, -32.92499999999999716, 99.99999999999998579 ) ) ;
#7319=CARTESIAN_POINT ( 'NONE',  ( 229.5999999999999375, -32.23124999877096286, 98.26794919243111792 ) ) ;
#7320=CARTESIAN_POINT ( 'NONE',  ( 229.5999999999999375, -34.44374999877096144, -50.00000000000011369 ) ) ;
#7326=CARTESIAN_POINT ( 'NONE',  ( 235.5999999999999943, -34.23749999999999716, -51.73205080756900287 ) ) ;
#7331=ADVANCED_FACE ( 'NONE', ( #12789 ), #15393, .F. ) ;
#7336=FACE_OUTER_BOUND ( 'NONE', #19147, .T. ) ;
#7339=CARTESIAN_POINT ( 'NONE',  ( 232.5999999999999375, -30.70312499938548001, 96.81714838363319586 ) ) ;
#7341=CARTESIAN_POINT ( 'NONE',  ( 0.000000000000000000, 0.000000000000000000, 0.000000000000000000 ) ) ;
#7343=CARTESIAN_POINT ( 'NONE',  ( 232.5999999999999375, -32.36249999999999716, -53.00000000000011369 ) ) ;
#7345=DIRECTION ( 'NONE',  ( 0.000000000000000000, 0.000000000000000000, 1.000000000000000000 ) ) ;
#7349=CARTESIAN_POINT ( 'NONE',  ( 229.8435696437499871, -32.87812499938547717, -51.59142580818350865 ) ) ;
#7358=CARTESIAN_POINT ( 'NONE',  ( 235.3564303562499447, -31.71562499938547575, 99.99999999999998579 ) ) ;
#7360=CARTESIAN_POINT ( 'NONE',  ( 229.8435696437499587, -34.22812499938547859, -51.59142580818350154 ) ) ;
#7363=CARTESIAN_POINT ( 'NONE',  ( 229.8435696437499871, -34.67812499938547433, -51.59142580818350865 ) ) ;
#7367=ORIENTED_EDGE ( 'NONE', *, *, #1723, .F. ) ;
#7370=ADVANCED_FACE ( 'NONE', ( #15657 ), #816, .F. ) ;
#7371=FACE_OUTER_BOUND ( 'NONE', #3481, .T. ) ;
#7375=CARTESIAN_POINT ( 'NONE',  ( 229.8435696437499587, -32.80312499938548143, 101.5914258081833879 ) ) ;
#7379=CARTESIAN_POINT ( 'NONE',  ( 232.6092389720419646, -31.99999999999999289, -47.13047754280724178 ) ) ;
#7381=CARTESIAN_POINT ( 'NONE',  ( 235.5999999999999943, -32.06249999999999289, 101.7320508075688537 ) ) ;
#7384=EDGE_CURVE ( 'NONE', #14449, #15949, #6678, .T. ) ;
#7385=CARTESIAN_POINT ( 'NONE',  ( 229.5999999999999375, -33.18749999999999289, -51.73205080756898866 ) ) ;
#7390=CYLINDRICAL_SURFACE ( 'NONE', #15520, 3.000000000000002665 ) ;
#7391=CARTESIAN_POINT ( 'NONE',  ( 232.5999999999999375, -29.99999999999999645, 99.99999999999998579 ) ) ;
#7397=CARTESIAN_POINT ( 'NONE',  ( 244.7999999999999545, -29.80000000000000426, -100.0000000000000000 ) ) ;
#7399=( BOUNDED_CURVE ( )  B_SPLINE_CURVE ( 2, ( #10732, #9457, #11018, #16695, #2033, #8097, #6636, #13848, #15522 ),
 .UNSPECIFIED., .F., .F. ) 
 B_SPLINE_CURVE_WITH_KNOTS ( ( 3, 2, 2, 2, 3 ),
 ( 0.8541666666666668517, 0.8611111111111111605, 0.8750000000000000000, 0.8888888888888888395, 0.8958333333333332593 ),
 .UNSPECIFIED. ) 
 CURVE ( )  GEOMETRIC_REPRESENTATION_ITEM ( )  RATIONAL_B_SPLINE_CURVE ( ( 0.9330127018922194093, 0.9330127018922209636, 1.000000000000000000, 0.8660254037844387076, 1.000000000000000000, 0.8660254037844387076, 1.000000000000000000, 0.9330127018922198534, 0.9330127018922192983 ) ) 
 REPRESENTATION_ITEM ( '' )  );
#7400=CARTESIAN_POINT ( 'NONE',  ( 232.5999999999999375, -33.43124999877096570, -47.00000000000011369 ) ) ;
#7402=CARTESIAN_POINT ( 'NONE',  ( 229.8435696437499871, -32.91562499938547859, 101.5914258081833879 ) ) ;
#7408=CARTESIAN_POINT ( 'NONE',  ( 232.5999999999999375, -33.20624999877097139, 97.00000000000000000 ) ) ;
#7411=CARTESIAN_POINT ( 'NONE',  ( 229.5999999999999375, -33.56249999999999289, 101.7320508075688679 ) ) ;
#7415=CARTESIAN_POINT ( 'NONE',  ( 235.5999999999999943, -34.18124999877096570, 98.26794919243110371 ) ) ;
#7416=CARTESIAN_POINT ( 'NONE',  ( 234.0999999999999375, -33.24374999877096570, -52.59807621135342970 ) ) ;
#7418=AXIS2_PLACEMENT_3D ( 'NONE', #7490, #14710, #16741 ) ;
#7421=FACE_OUTER_BOUND ( 'NONE', #19250, .T. ) ;
#7438=CARTESIAN_POINT ( 'NONE',  ( 229.8435696437499871, -30.55312499938547788, 101.5914258081833879 ) ) ;
#7441=CARTESIAN_POINT ( 'NONE',  ( 246.9999999999999716, -35.00000000000000000, -100.0000000000000000 ) ) ;
#7442=EDGE_CURVE ( 'NONE', #5820, #18598, #10267, .T. ) ;
#7447=CARTESIAN_POINT ( 'NONE',  ( 235.3564303562499447, -31.71562499938547575, -50.00000000000011369 ) ) ;
#7449=ORIENTED_EDGE ( 'NONE', *, *, #7742, .T. ) ;
#7452=EDGE_CURVE ( 'NONE', #8905, #7231, #14084, .T. ) ;
#7456=CARTESIAN_POINT ( 'NONE',  ( 233.9782151781249411, -34.34062499938547575, 97.61286128772489690 ) ) ;
#7457=CARTESIAN_POINT ( 'NONE',  ( 235.3564303562499447, -33.96562499938547575, -50.00000000000011369 ) ) ;
#7461=CARTESIAN_POINT ( 'NONE',  ( 229.5999999999999375, -30.86249999999999361, -48.26794919243123161 ) ) ;
#7469=CARTESIAN_POINT ( 'NONE',  ( 235.3564303562499447, -30.89062499938548001, -51.59142580818350865 ) ) ;
#7474=CARTESIAN_POINT ( 'NONE',  ( 231.2217848218749339, -34.11562499938548143, 102.3871387122750889 ) ) ;
#7477=CARTESIAN_POINT ( 'NONE',  ( 99.99999999999997158, -29.80000000000000071, 150.0000000000000000 ) ) ;
#7484=CARTESIAN_POINT ( 'NONE',  ( 232.5999999999999375, -33.26249999999999574, -53.00000000000011369 ) ) ;
#7489=FACE_OUTER_BOUND ( 'NONE', #17202, .T. ) ;
#7490=CARTESIAN_POINT ( 'NONE',  ( 105.1999999999999744, -34.99999999999999289, -100.0000000000000000 ) ) ;
#7495=EDGE_CURVE ( 'NONE', #5414, #927, #2073, .T. ) ;
#7500=CARTESIAN_POINT ( 'NONE',  ( 229.5999999999999375, -34.46249999999999147, -48.26794919243123161 ) ) ;
#7501=CARTESIAN_POINT ( 'NONE',  ( 231.2217848218749339, -32.87812499938547717, 102.3871387122750889 ) ) ;
#7508=CARTESIAN_POINT ( 'NONE',  ( 231.0999999999999375, -34.42499999999999716, 102.5980762113533018 ) ) ;
#7510=CARTESIAN_POINT ( 'NONE',  ( 229.8435696437499303, -32.95312499938548001, -50.00000000000011369 ) ) ;
#7511=CARTESIAN_POINT ( 'NONE',  ( 229.8435696437499303, -30.25312499938548072, 99.99999999999998579 ) ) ;
#7512=CARTESIAN_POINT ( 'NONE',  ( 232.5999999999999375, -33.88124999877096144, -46.53589838486234953 ) ) ;
#7515=ORIENTED_EDGE ( 'NONE', *, *, #8590, .F. ) ;
#7521=ORIENTED_EDGE ( 'NONE', *, *, #19036, .T. ) ;
#7530=EDGE_CURVE ( 'NONE', #8610, #5766, #12523, .T. ) ;
#7531=CARTESIAN_POINT ( 'NONE',  ( 235.3564303562499447, -30.85312499938547859, 101.5914258081833879 ) ) ;
#7533=( LENGTH_UNIT ( ) NAMED_UNIT ( * ) SI_UNIT ( .MILLI., .METRE. ) );
#7538=CARTESIAN_POINT ( 'NONE',  ( 105.1999999999999886, -4.999999999999993783, -103.0000000000000995 ) ) ;
#7540=CARTESIAN_POINT ( 'NONE',  ( 232.5999999999999375, -32.05312499938548143, -53.18285161636690361 ) ) ;
#7541=ORIENTED_EDGE ( 'NONE', *, *, #13926, .F. ) ;
#7548=CARTESIAN_POINT ( 'NONE',  ( 229.8435696437499303, -34.64062499938548001, 99.99999999999998579 ) ) ;
#7549=CARTESIAN_POINT ( 'NONE',  ( 229.8435696437499303, -34.64062499938548001, -50.00000000000011369 ) ) ;
#7556=CARTESIAN_POINT ( 'NONE',  ( 232.5999999999999375, -34.52812499938548285, -46.81714838363331666 ) ) ;
#7561=DIRECTION ( 'NONE',  ( -0.000000000000000000, -1.000000000000000000, -0.000000000000000000 ) ) ;
#7562=CARTESIAN_POINT ( 'NONE',  ( 235.3564303562499447, -30.92812499938547788, -50.00000000000011369 ) ) ;
#7568=CARTESIAN_POINT ( 'NONE',  ( 229.8435696437499587, -34.15312499938547575, 101.5914258081833879 ) ) ;
#7571=EDGE_CURVE ( 'NONE', #5414, #484, #1006, .T. ) ;
#7574=CARTESIAN_POINT ( 'NONE',  ( 230.2961164517930968, -35.00002705695778360, 98.07851859032987818 ) ) ;
#7583=ORIENTED_EDGE ( 'NONE', *, *, #17371, .F. ) ;
#7595=CARTESIAN_POINT ( 'NONE',  ( 232.5999999999999375, -31.26562499938548356, 96.81714838363319586 ) ) ;
#7600=PLANE ( 'NONE',  #10537 ) ;
#7604=CARTESIAN_POINT ( 'NONE',  ( 229.5999999999999375, -32.66249999999999432, 101.7320508075688679 ) ) ;
#7606=CARTESIAN_POINT ( 'NONE',  ( 233.9782151781249411, -34.00312499938547717, -52.38713871227520968 ) ) ;
#7608=CARTESIAN_POINT ( 'NONE',  ( 234.0999999999999375, -34.14374999877096428, 97.40192378864668399 ) ) ;
#7609=CARTESIAN_POINT ( 'NONE',  ( 235.5999999999999943, -33.35624999877096997, -48.26794919243124582 ) ) ;
#7612=EDGE_CURVE ( 'NONE', #13878, #11119, #14575, .T. ) ;
#7617=ORIENTED_EDGE ( 'NONE', *, *, #15618, .T. ) ;
#7619=CARTESIAN_POINT ( 'NONE',  ( 232.5999999999999375, -29.99999999999999645, -47.00000000000010658 ) ) ;
#7623=CARTESIAN_POINT ( 'NONE',  ( 231.0999999999999375, -33.67499999999999716, 97.40192378864668399 ) ) ;
#7627=CARTESIAN_POINT ( 'NONE',  ( 231.2217848218749339, -31.86562499938547788, 102.3871387122750889 ) ) ;
#7628=ORIENTED_EDGE ( 'NONE', *, *, #2560, .F. ) ;
#7635=CARTESIAN_POINT ( 'NONE',  ( 232.5999999999999375, -34.30312499938547433, -53.18285161636690361 ) ) ;
#7636=ORIENTED_EDGE ( 'NONE', *, *, #6072, .T. ) ;
#7642=CARTESIAN_POINT ( 'NONE',  ( 233.9782151781249411, -32.69062499938547717, 102.3871387122750889 ) ) ;
#7643=CARTESIAN_POINT ( 'NONE',  ( 233.9782151781249411, -34.04062499938547859, -47.61286128772501769 ) ) ;
#7648=CARTESIAN_POINT ( 'NONE',  ( 229.5999999999999375, -33.11249999999999716, -48.26794919243123161 ) ) ;
#7653=CARTESIAN_POINT ( 'NONE',  ( 235.3564303562499447, -32.76562499938548001, -48.40857419181671162 ) ) ;
#7657=AXIS2_PLACEMENT_3D ( 'NONE', #7477, #16568, #17837 ) ;
#7665=CARTESIAN_POINT ( 'NONE',  ( 231.3449744686888891, -35.00000000000002842, 102.4885329066886470 ) ) ;
#7667=CARTESIAN_POINT ( 'NONE',  ( 232.5999999999999375, -29.99999999999999645, 96.99999999999998579 ) ) ;
#7668=CARTESIAN_POINT ( 'NONE',  ( 232.5999999999999375, -30.25312499938548072, -53.18285161636690361 ) ) ;
#7677=EDGE_CURVE ( 'NONE', #3788, #11929, #9082, .T. ) ;
#7679=CARTESIAN_POINT ( 'NONE',  ( 234.0999999999999375, -32.09999999999999432, -47.40192378864679768 ) ) ;
#7680=EDGE_LOOP ( 'NONE', ( #17686, #3322, #10353, #12158 ) ) ;
#7683=DIRECTION ( 'NONE',  ( 0.000000000000000000, 0.000000000000000000, 1.000000000000000000 ) ) ;
#7688=CARTESIAN_POINT ( 'NONE',  ( 229.8435696437499871, -33.36562499938548143, 101.5914258081833879 ) ) ;
#7695=DIRECTION ( 'NONE',  ( -0.000000000000000000, -1.000000000000000000, -0.000000000000000000 ) ) ;
#7698=CARTESIAN_POINT ( 'NONE',  ( 231.0999999999999375, -33.67499999999999716, 97.40192378864668399 ) ) ;
#7701=CARTESIAN_POINT ( 'NONE',  ( 233.9782151781249411, -32.35312499938547859, -47.61286128772501769 ) ) ;
#7703=CARTESIAN_POINT ( 'NONE',  ( 231.2217848218749339, -30.62812499938548072, 102.3871387122750889 ) ) ;
#7704=CARTESIAN_POINT ( 'NONE',  ( 231.2217848218749339, -30.62812499938548072, -47.61286128772501769 ) ) ;
#7707=ORIENTED_EDGE ( 'NONE', *, *, #19145, .F. ) ;
#7710=CARTESIAN_POINT ( 'NONE',  ( 232.5999999999999375, -33.93749999999999289, 103.0000000000000000 ) ) ;
#7714=CARTESIAN_POINT ( 'NONE',  ( 233.4038475772933339, -32.56740381056765443, 102.9999999999999858 ) ) ;
#7718=CARTESIAN_POINT ( 'NONE',  ( 232.5999999999999375, -29.99999999999999645, 99.99999999999998579 ) ) ;
#7720=DIRECTION ( 'NONE',  ( 1.000000000000000000, -0.000000000000000000, -0.000000000000000000 ) ) ;
#7723=LINE ( 'NONE', #12314, #14598 ) ;
#7725=CARTESIAN_POINT ( 'NONE',  ( 231.2217848218749339, -32.31562499938547717, 102.3871387122750889 ) ) ;
#7726=ORIENTED_EDGE ( 'NONE', *, *, #8279, .F. ) ;
#7727=VECTOR ( 'NONE', #13871, 1000.000000000000000 ) ;
#7735=VECTOR ( 'NONE', #1426, 1000.000000000000000 ) ;
#7739=B_SPLINE_CURVE_WITH_KNOTS ( 'NONE', 3,
 ( #7158, #18986, #15860, #3932, #8613, #11358, #5609, #15760, #14564, #17516, #8329, #17323, #4035, #9995, #6878, #11553, #2647, #19077 ),
 .UNSPECIFIED., .F., .F.,
 ( 4, 2, 2, 2, 2, 2, 2, 2, 4 ),
 ( 0.000000000000000000, 0.0007106627595359582506, 0.001421325519071916501, 0.002131988278607874644, 0.002842651038143833003, 0.003553313797679791362, 0.004263976557215749287, 0.004974639316751707646, 0.005685302076287666005 ),
 .UNSPECIFIED. ) ;
#7742=EDGE_CURVE ( 'NONE', #4852, #17012, #12256, .T. ) ;
#7744=AXIS2_PLACEMENT_3D ( 'NONE', #1352, #13356, #7201 ) ;
#7746=CARTESIAN_POINT ( 'NONE',  ( 233.9782151781249411, -34.79062499938547859, 97.61286128772489690 ) ) ;
#7753=CARTESIAN_POINT ( 'NONE',  ( 234.0999999999999375, -33.74999999999999289, -52.59807621135342970 ) ) ;
#7758=CARTESIAN_POINT ( 'NONE',  ( 231.2217848218749339, -32.42812499938548143, -47.61286128772501769 ) ) ;
#7763=AXIS2_PLACEMENT_3D ( 'NONE', #2597, #15897, #9939 ) ;
#7764=CARTESIAN_POINT ( 'NONE',  ( 232.5999999999999943, -33.85312499938547859, 96.81714838363319586 ) ) ;
#7766=CARTESIAN_POINT ( 'NONE',  ( 235.5999999999999375, -34.72499999999999432, 99.99999999999998579 ) ) ;
#7771=CARTESIAN_POINT ( 'NONE',  ( 233.4038475772933339, -32.83259618943232994, -53.00000000000011369 ) ) ;
#7775=VERTEX_POINT ( 'NONE', #16329 ) ;
#7777=CARTESIAN_POINT ( 'NONE',  ( 105.1999999999999744, -29.80000000000000071, -100.0000000000000000 ) ) ;
#7787=CARTESIAN_POINT ( 'NONE',  ( 231.2217848218749339, -33.77812499938547575, 102.3871387122750889 ) ) ;
#7798=CARTESIAN_POINT ( 'NONE',  ( 233.9782151781249411, -32.65312499938548285, -52.38713871227520968 ) ) ;
#7800=CARTESIAN_POINT ( 'NONE',  ( 229.8435696437499871, -33.44062499938547717, 98.40857419181659793 ) ) ;
#7801=CARTESIAN_POINT ( 'NONE',  ( 229.8435696437499303, -30.70312499938548001, -50.00000000000011369 ) ) ;
#7802=ADVANCED_FACE ( 'NONE', ( #7336 ), #11924, .F. ) ;
#7806=DIRECTION ( 'NONE',  ( 0.000000000000000000, -1.000000000000000000, 0.000000000000000000 ) ) ;
#7809=ORIENTED_EDGE ( 'NONE', *, *, #13883, .T. ) ;
#7820=CARTESIAN_POINT ( 'NONE',  ( 229.8435696437499303, -33.29062499938547148, 99.99999999999998579 ) ) ;
#7822=CARTESIAN_POINT ( 'NONE',  ( 229.8435696437499871, -32.80312499938548143, 101.5914258081833879 ) ) ;
#7831=CARTESIAN_POINT ( 'NONE',  ( 232.5999999999999375, -33.43124999877096570, 102.9999999999999858 ) ) ;
#7835=ADVANCED_FACE ( 'NONE', ( #123 ), #6074, .F. ) ;
#7839=CARTESIAN_POINT ( 'NONE',  ( 235.3564303562499447, -33.47812499938547148, 98.40857419181659793 ) ) ;
#7844=CARTESIAN_POINT ( 'NONE',  ( 234.0999999999999375, -31.94999999999999218, -52.59807621135342970 ) ) ;
#7848=CARTESIAN_POINT ( 'NONE',  ( 229.8435696437499587, -33.44062499938547717, 98.40857419181659793 ) ) ;
#7850=CARTESIAN_POINT ( 'NONE',  ( 229.8435696437499871, -33.36562499938548143, -48.40857419181671162 ) ) ;
#7859=AXIS2_PLACEMENT_3D ( 'NONE', #13092, #2737, #7230 ) ;
#7860=CARTESIAN_POINT ( 'NONE',  ( 230.2593261479345301, -32.00000000000000000, -51.46660719531470107 ) ) ;
#7865=CARTESIAN_POINT ( 'NONE',  ( 232.5999999999999375, -31.15312499938547930, -53.18285161636690361 ) ) ;
#7868=ORIENTED_EDGE ( 'NONE', *, *, #5074, .F. ) ;
#7870=AXIS2_PLACEMENT_3D ( 'NONE', #11253, #6382, #13886 ) ;
#7871=( NAMED_UNIT ( * ) PLANE_ANGLE_UNIT ( ) SI_UNIT ( $, .RADIAN. ) );
#7881=CARTESIAN_POINT ( 'NONE',  ( 229.8435696437499303, -30.14062499938548001, 99.99999999999998579 ) ) ;
#7886=CARTESIAN_POINT ( 'NONE',  ( 230.0213320530827730, -31.99999999999999289, 99.01001922939823885 ) ) ;
#7889=FACE_OUTER_BOUND ( 'NONE', #3139, .T. ) ;
#7891=CARTESIAN_POINT ( 'NONE',  ( 232.5999999999999375, -29.99999999999999645, 99.99999999999998579 ) ) ;
#7893=CARTESIAN_POINT ( 'NONE',  ( 235.3564303562499447, -32.31562499938547717, -48.40857419181671162 ) ) ;
#7895=CARTESIAN_POINT ( 'NONE',  ( 235.3564303562499447, -32.76562499938548001, 101.5914258081833879 ) ) ;
#7896=CARTESIAN_POINT ( 'NONE',  ( 235.3564303562499447, -30.92812499938547788, -50.00000000000011369 ) ) ;
#7898=VERTEX_POINT ( 'NONE', #9277 ) ;
#7900=CARTESIAN_POINT ( 'NONE',  ( 231.7961524227065695, -32.55134618820330417, -47.00000000000011369 ) ) ;
#7913=CARTESIAN_POINT ( 'NONE',  ( 102.9999999999999858, -5.200000000000008171, -100.0000000000000000 ) ) ;
#7914=CARTESIAN_POINT ( 'NONE',  ( 231.0999999999999375, -34.81874999877096144, -47.40192378864679768 ) ) ;
#7915=CARTESIAN_POINT ( 'NONE',  ( 231.1166048115126443, -35.16733441503057378, 97.47959136244114120 ) ) ;
#7921=CARTESIAN_POINT ( 'NONE',  ( 244.7999999999999545, -29.80000000000000426, -100.0000000000000000 ) ) ;
#7924=ORIENTED_EDGE ( 'NONE', *, *, #13883, .F. ) ;
#7925=CARTESIAN_POINT ( 'NONE',  ( 235.3564303562499447, -34.37812499938547717, -51.59142580818350865 ) ) ;
#7926=ORIENTED_EDGE ( 'NONE', *, *, #8215, .T. ) ;
#7939=( BOUNDED_CURVE ( )  B_SPLINE_CURVE ( 2, ( #6235, #16775, #18151, #13831, #4773, #18247, #3389, #9341, #15304 ),
 .UNSPECIFIED., .F., .T. ) 
 B_SPLINE_CURVE_WITH_KNOTS ( ( 3, 2, 2, 2, 3 ),
 ( 0.4375000000000001110, 0.4444444444444444198, 0.4583333333333333148, 0.4722222222222222099, 0.4791666666666666852 ),
 .UNSPECIFIED. ) 
 CURVE ( )  GEOMETRIC_REPRESENTATION_ITEM ( )  RATIONAL_B_SPLINE_CURVE ( ( 0.9330127018922194093, 0.9330127018922204085, 1.000000000000000000, 0.8660254037844387076, 1.000000000000000000, 0.8660254037844387076, 1.000000000000000000, 0.9330127018922190762, 0.9330127018922194093 ) ) 
 REPRESENTATION_ITEM ( '' )  );
#7942=CARTESIAN_POINT ( 'NONE',  ( 229.5999999999999375, -32.69999999999999574, -50.00000000000011369 ) ) ;
#7945=CARTESIAN_POINT ( 'NONE',  ( 235.3564303562499447, -33.21562499938548285, 101.5914258081833879 ) ) ;
#7947=CARTESIAN_POINT ( 'NONE',  ( 235.3564303562499447, -33.21562499938548285, -48.40857419181671162 ) ) ;
#7952=CARTESIAN_POINT ( 'NONE',  ( 244.7999999999999545, -29.80000000000002203, 147.7999999999999829 ) ) ;
#7959=ADVANCED_FACE ( 'NONE', ( #2239 ), #5284, .T. ) ;
#7960=CARTESIAN_POINT ( 'NONE',  ( 229.8435696437499871, -30.17812499938547433, -51.59142580818350865 ) ) ;
#7966=AXIS2_PLACEMENT_3D ( 'NONE', #16680, #6615, #10907 ) ;
#7972=CARTESIAN_POINT ( 'NONE',  ( 231.0999999999999375, -34.36874999877096570, -47.40192378864679768 ) ) ;
#7974=CARTESIAN_POINT ( 'NONE',  ( 232.5999999999999659, -32.53124999877096712, -47.00000000000011369 ) ) ;
#7975=CARTESIAN_POINT ( 'NONE',  ( 231.2217848218749339, -34.82812499938548001, 97.61286128772489690 ) ) ;
#7978=ORIENTED_EDGE ( 'NONE', *, *, #19168, .F. ) ;
#7980=CARTESIAN_POINT ( 'NONE',  ( 244.7999999999999545, -35.00000000000000000, -100.0000000000000000 ) ) ;
#7984=FACE_OUTER_BOUND ( 'NONE', #9771, .T. ) ;
#7987=ORIENTED_EDGE ( 'NONE', *, *, #3851, .T. ) ;
#7988=CARTESIAN_POINT ( 'NONE',  ( 233.9782151781249411, -34.60312499938548569, -47.61286128772501769 ) ) ;
#7990=CARTESIAN_POINT ( 'NONE',  ( 235.3564303562499447, -33.14062499938548001, 98.40857419181659793 ) ) ;
#7991=CARTESIAN_POINT ( 'NONE',  ( 229.8435696437499871, -31.19062499938548072, -51.59142580818350865 ) ) ;
#8007=CARTESIAN_POINT ( 'NONE',  ( 229.5999999999999375, -33.95624999877096428, -48.26794919243123161 ) ) ;
#8008=FACE_OUTER_BOUND ( 'NONE', #7226, .T. ) ;
#8009=CARTESIAN_POINT ( 'NONE',  ( 231.7447645400923193, -35.19352049914630953, 96.73097394877602540 ) ) ;
#8012=CARTESIAN_POINT ( 'NONE',  ( 231.0999999999999375, -32.26874999877096428, 97.40192378864668399 ) ) ;
#8019=CARTESIAN_POINT ( 'NONE',  ( 233.9782151781249411, -34.79062499938547859, -52.38713871227520968 ) ) ;
#8022=( BOUNDED_CURVE ( )  B_SPLINE_CURVE ( 2, ( #15275, #8240, #8141, #16938, #18408, #9706, #535, #18604, #16846, #14190, #5218, #4931, #6491, #12533, #11066, #1988, #14093, #11168, #6786, #3550, #12440, #6586, #18703, #637, #6392, #3450, #2085, #18312, #15572, #15372, #12734, #5028, #5322, #7945, #15473, #2185, #17229, #13897, #1890, #7848, #9506, #8041, #13999, #7059, #5789, #15863, #2470, #11650, #13204, #4131, #17610, #1018, #13018, #923, #12922, #14566, #14379, #18795, #5611, #13109, #5420, #1203, #19176, #17518, #14470, #12828, #5698, #4226, #19079, #18990, #6880, #7160, #11360, #15763, #9801, #17325, #10182, #14667, #3833, #16145, #3934, #8615, #2758 ),
 .UNSPECIFIED., .F., .F. ) 
 B_SPLINE_CURVE_WITH_KNOTS ( ( 3, 2, 2, 2, 2, 2, 2, 2, 2, 2, 2, 2, 2, 2, 2, 2, 2, 2, 2, 2, 2, 2, 2, 2, 2, 2, 2, 2, 2, 2, 2, 2, 2, 2, 2, 2, 2, 2, 2, 2, 2, 3 ),
 ( 0.3495698921800969305, 0.3600184345287980592, 0.3750192026341646057, 0.3900199707395312076, 0.4050207388448978096, 0.4200215069502644116, 0.4350222750556310136, 0.4500230431609976156, 0.4650238112663641621, 0.4800245793717307086, 0.4950253474770973661, 0.5100261155824639125, 0.5250268836878304590, 0.5400276517931971165, 0.5550284198985636630, 0.5700291880039303205, 0.5850299561092967560, 0.6000307242146634135, 0.6150314923200299599, 0.6300322604253966174, 0.6450330285307631639, 0.6600337966361298214, 0.6750345647414963679, 0.6900353328468629144, 0.7050361009522295719, 0.7200368690575961184, 0.7350376371629627759, 0.7500384052683293223, 0.7650391733736958688, 0.7800399414790624153, 0.7950407095844291838, 0.8100414776897956193, 0.8250422457951621658, 0.8400430139005288233, 0.8550437820058953697, 0.8700445501112620272, 0.8850453182166285737, 0.9000460863219952312, 0.9150468544273617777, 0.9300476225327284352, 0.9450483906380949817, 0.9496006163947608991 ),
 .UNSPECIFIED. ) 
 CURVE ( )  GEOMETRIC_REPRESENTATION_ITEM ( )  RATIONAL_B_SPLINE_CURVE ( ( 0.9433623850486696494, 0.9066821623815634057, 1.000000000000000000, 0.8660254037844387076, 1.000000000000000000, 0.8660254037844387076, 1.000000000000000000, 0.8660254037844387076, 1.000000000000000000, 0.8660254037844387076, 1.000000000000000000, 0.8660254037844387076, 1.000000000000000000, 0.8660254037844387076, 1.000000000000000000, 0.8660254037844387076, 1.000000000000000000, 0.8660254037844387076, 1.000000000000000000, 0.8660254037844387076, 1.000000000000000000, 0.8660254037844387076, 1.000000000000000000, 0.8660254037844387076, 1.000000000000000000, 0.8660254037844387076, 1.000000000000000000, 0.8660254037844387076, 1.000000000000000000, 0.8660254037844387076, 1.000000000000000000, 0.8660254037844387076, 1.000000000000000000, 0.8660254037844387076, 1.000000000000000000, 0.8660254037844387076, 1.000000000000000000, 0.8660254037844387076, 1.000000000000000000, 0.8660254037844387076, 1.000000000000000000, 0.8660254037844387076, 1.000000000000000000, 0.8660254037844387076, 1.000000000000000000, 0.8660254037844387076, 1.000000000000000000, 0.8660254037844387076, 1.000000000000000000, 0.8660254037844387076, 1.000000000000000000, 0.8660254037844387076, 1.000000000000000000, 0.8660254037844387076, 1.000000000000000000, 0.8660254037844387076, 1.000000000000000000, 0.8660254037844387076, 1.000000000000000000, 0.8660254037844387076, 1.000000000000000000, 0.8660254037844387076, 1.000000000000000000, 0.8660254037844387076, 1.000000000000000000, 0.8660254037844387076, 1.000000000000000000, 0.8660254037844387076, 1.000000000000000000, 0.8660254037844387076, 1.000000000000000000, 0.8660254037844387076, 1.000000000000000000, 0.8660254037844387076, 1.000000000000000000, 0.8660254037844387076, 1.000000000000000000, 0.8660254037844387076, 1.000000000000000000, 0.8660254037844387076, 1.000000000000000000, 0.9593432414028713051, 0.9433623850486665408 ) ) 
 REPRESENTATION_ITEM ( '' )  );
#8023=CARTESIAN_POINT ( 'NONE',  ( 232.5999999999999375, -33.26249999999999574, -53.00000000000011369 ) ) ;
#8026=VECTOR ( 'NONE', #12669, 1000.000000000000000 ) ;
#8030=CARTESIAN_POINT ( 'NONE',  ( 244.7999999999999545, -29.80000000000000782, -100.0000000000000000 ) ) ;
#8034=ADVANCED_FACE ( 'NONE', ( #8298 ), #14437, .F. ) ;
#8037=CARTESIAN_POINT ( 'NONE',  ( 229.5999999999999375, -32.24999999999999289, -50.00000000000011369 ) ) ;
#8039=VECTOR ( 'NONE', #9994, 1000.000000000000000 ) ;
#8041=CARTESIAN_POINT ( 'NONE',  ( 232.5999999999999943, -33.51562499938548001, 96.81714838363319586 ) ) ;
#8043=CARTESIAN_POINT ( 'NONE',  ( 229.8435696437499871, -33.44062499938547717, -51.59142580818350865 ) ) ;
#8045=EDGE_CURVE ( 'NONE', #15137, #4556, #2618, .T. ) ;
#8051=VECTOR ( 'NONE', #15050, 1000.000000000000000 ) ;
#8061=CARTESIAN_POINT ( 'NONE',  ( 229.8435696437499303, -30.14062499938548001, -50.00000000000011369 ) ) ;
#8076=EDGE_CURVE ( 'NONE', #12940, #17759, #2896, .T. ) ;
#8078=B_SPLINE_CURVE_WITH_KNOTS ( 'NONE', 3,
 ( #2020, #12768, #12476, #2126, #3774, #16972, #11300, #9347, #15310, #1923, #7886, #13837, #17460, #5457, #1338, #11683 ),
 .UNSPECIFIED., .F., .F.,
 ( 4, 2, 2, 2, 2, 2, 2, 4 ),
 ( 0.000000000000000000, 0.0005391024520905149430, 0.001078204904181029886, 0.002156409808361992118, 0.002695512260452471390, 0.003234614712542950229, 0.003773717164633429936, 0.004312819616723909642 ),
 .UNSPECIFIED. ) ;
#8079=CARTESIAN_POINT ( 'NONE',  ( 231.2217848218749339, -30.21562499938547575, 97.61286128772489690 ) ) ;
#8081=ORIENTED_EDGE ( 'NONE', *, *, #4601, .T. ) ;
#8089=CARTESIAN_POINT ( 'NONE',  ( 232.5999999999999375, -34.83749999999999147, 103.4641016151377499 ) ) ;
#8092=CARTESIAN_POINT ( 'NONE',  ( 235.3564303562499447, -32.69062499938547717, 98.40857419181659793 ) ) ;
#8094=CARTESIAN_POINT ( 'NONE',  ( 235.5999999999999943, -34.70624999877096428, -48.26794919243124582 ) ) ;
#8097=CARTESIAN_POINT ( 'NONE',  ( 235.5999999999999943, -34.76249999999999574, -48.26794919243124582 ) ) ;
#8101=CYLINDRICAL_SURFACE ( 'NONE', #4431, 5.199999999999996625 ) ;
#8112=CARTESIAN_POINT ( 'NONE',  ( 231.2217848218749339, -34.56562499938547717, 102.3871387122750889 ) ) ;
#8116=FACE_BOUND ( 'NONE', #795, .T. ) ;
#8138=CARTESIAN_POINT ( 'NONE',  ( 230.9855258467272563, -35.02670941564509377, -52.74312242118950422 ) ) ;
#8141=CARTESIAN_POINT ( 'NONE',  ( 229.8435696437499303, -32.05312499938548143, 99.99999999999998579 ) ) ;
#8143=CARTESIAN_POINT ( 'NONE',  ( 232.5999999999999375, -34.86562499938548143, -53.18285161636690361 ) ) ;
#8159=CARTESIAN_POINT ( 'NONE',  ( 231.2217848218749339, -32.01562499938548001, -52.38713871227520968 ) ) ;
#8162=ORIENTED_EDGE ( 'NONE', *, *, #19285, .T. ) ;
#8164=CARTESIAN_POINT ( 'NONE',  ( 232.5999999999999375, -34.16249999999999432, 96.99999999999997158 ) ) ;
#8168=EDGE_LOOP ( 'NONE', ( #10113, #8194, #8790, #17680 ) ) ;
#8171=LINE ( 'NONE', #4962, #10360 ) ;
#8176=CARTESIAN_POINT ( 'NONE',  ( 232.5999999999999375, -31.37812499938547717, 103.1828516163667899 ) ) ;
#8186=EDGE_LOOP ( 'NONE', ( #11019, #1207, #8081, #5748 ) ) ;
#8187=CARTESIAN_POINT ( 'NONE',  ( 233.9782151781249411, -34.90312499938547575, -52.38713871227520968 ) ) ;
#8189=CARTESIAN_POINT ( 'NONE',  ( 235.3564303562499447, -33.66562499938548569, 101.5914258081833879 ) ) ;
#8190=CARTESIAN_POINT ( 'NONE',  ( 229.8435696437499871, -33.44062499938547717, -51.59142580818350865 ) ) ;
#8193=CARTESIAN_POINT ( 'NONE',  ( 229.5999999999999375, -32.73749999999999716, -51.73205080756898866 ) ) ;
#8194=ORIENTED_EDGE ( 'NONE', *, *, #13730, .F. ) ;
#8197=DIRECTION ( 'NONE',  ( 1.000000000000000000, 0.000000000000000000, 0.000000000000000000 ) ) ;
#8202=CARTESIAN_POINT ( 'NONE',  ( 231.2217848218749339, -30.62812499938548072, 102.3871387122750889 ) ) ;
#8210=CARTESIAN_POINT ( 'NONE',  ( 231.2217848218749339, -34.26562499938548001, 97.61286128772489690 ) ) ;
#8215=EDGE_CURVE ( 'NONE', #5767, #12372, #14036, .T. ) ;
#8216=CARTESIAN_POINT ( 'NONE',  ( 232.5999999999999375, -30.50624999877096144, 96.53589838486223584 ) ) ;
#8217=CARTESIAN_POINT ( 'NONE',  ( 232.5999999999999375, -31.63124999877096144, -46.53589838486234953 ) ) ;
#8220=CARTESIAN_POINT ( 'NONE',  ( 229.5999999999999375, -34.49999999999999289, 99.99999999999998579 ) ) ;
#8226=CARTESIAN_POINT ( 'NONE',  ( 232.5999999999999375, -34.16249999999999432, -53.00000000000010658 ) ) ;
#8228=CYLINDRICAL_SURFACE ( 'NONE', #5191, 3.000000000000009770 ) ;
#8232=CARTESIAN_POINT ( 'NONE',  ( 232.5999999999999375, -33.26249999999999574, 97.00000000000000000 ) ) ;
#8240=CARTESIAN_POINT ( 'NONE',  ( 229.8435696437499303, -32.02817623523064583, 101.0587761908871443 ) ) ;
#8242=CARTESIAN_POINT ( 'NONE',  ( 233.9782151781249411, -34.45312499938548001, -52.38713871227520968 ) ) ;
#8245=CARTESIAN_POINT ( 'NONE',  ( 234.0999999999999375, -33.74999999999999289, -52.59807621135342970 ) ) ;
#8249=CARTESIAN_POINT ( 'NONE',  ( 235.3564303562499447, -33.02812499938547575, -51.59142580818350154 ) ) ;
#8254=CARTESIAN_POINT ( 'NONE',  ( 229.8435696437499871, -32.80312499938548143, -48.40857419181671162 ) ) ;
#8256=VERTEX_POINT ( 'NONE', #18349 ) ;
#8261=DIRECTION ( 'NONE',  ( 0.000000000000000000, 0.000000000000000000, 1.000000000000000000 ) ) ;
#8271=CARTESIAN_POINT ( 'NONE',  ( 235.5999999999999943, -32.96249999999999858, 101.7320508075688537 ) ) ;
#8274=CARTESIAN_POINT ( 'NONE',  ( 235.2013144571816099, -31.99999999999998579, 98.52838665780598149 ) ) ;
#8279=EDGE_CURVE ( 'NONE', #3211, #5198, #2691, .T. ) ;
#8282=CARTESIAN_POINT ( 'NONE',  ( 232.5999999999999375, -34.19062499938547717, 103.1828516163667899 ) ) ;
#8283=CARTESIAN_POINT ( 'NONE',  ( 232.5999999999999375, -34.19062499938547717, -46.81714838363331666 ) ) ;
#8293=CIRCLE ( 'NONE', #17029, 2.199999999999993516 ) ;
#8298=FACE_OUTER_BOUND ( 'NONE', #12528, .T. ) ;
#8301=CARTESIAN_POINT ( 'NONE',  ( 232.5999999999999375, -32.36249999999999716, 96.53589838486223584 ) ) ;
#8304=CARTESIAN_POINT ( 'NONE',  ( 229.5999999999999375, -30.88124999877096144, 98.26794919243111792 ) ) ;
#8305=CARTESIAN_POINT ( 'NONE',  ( 234.0999999999999375, -30.54374999877096286, -52.59807621135342970 ) ) ;
#8311=EDGE_LOOP ( 'NONE', ( #2953, #5169, #7270, #7617 ) ) ;
#8317=CARTESIAN_POINT ( 'NONE',  ( 244.7999999999999545, -34.51168759575591594, -100.0000000000000000 ) ) ;
#8320=EDGE_CURVE ( 'NONE', #4792, #5820, #6160, .T. ) ;
#8322=DIRECTION ( 'NONE',  ( -0.000000000000000000, -0.000000000000000000, -1.000000000000000000 ) ) ;
#8329=CARTESIAN_POINT ( 'NONE',  ( 235.0804598586379939, -35.00000000000002132, 98.55723758691048886 ) ) ;
#8331=PLANE ( 'NONE',  #9909 ) ;
#8333=CARTESIAN_POINT ( 'NONE',  ( 235.3564303562499447, -31.30312499938547788, -48.40857419181671162 ) ) ;
#8342=CARTESIAN_POINT ( 'NONE',  ( 229.8435696437499303, -32.39062499938548001, -50.00000000000011369 ) ) ;
#8349=CARTESIAN_POINT ( 'NONE',  ( 233.9782151781249411, -33.89062499938548001, -52.38713871227520968 ) ) ;
#8352=ORIENTED_EDGE ( 'NONE', *, *, #4099, .F. ) ;
#8358=DIRECTION ( 'NONE',  ( -1.000000000000000000, 0.000000000000000000, 0.000000000000000000 ) ) ;
#8367=DIRECTION ( 'NONE',  ( -0.000000000000000000, -1.000000000000000000, -0.000000000000000000 ) ) ;
#8374=AXIS2_PLACEMENT_3D ( 'NONE', #16163, #10585, #18401 ) ;
#8376=ORIENTED_EDGE ( 'NONE', *, *, #9704, .F. ) ;
#8377=CARTESIAN_POINT ( 'NONE',  ( 235.2218879900010506, -35.00000000000000000, -49.14934632385183733 ) ) ;
#8379=CARTESIAN_POINT ( 'NONE',  ( 231.2217848218749339, -33.77812499938547575, 102.3871387122750889 ) ) ;
#8380=CARTESIAN_POINT ( 'NONE',  ( 232.5999999999999375, -32.61562499938548143, -53.18285161636690361 ) ) ;
#8393=CARTESIAN_POINT ( 'NONE',  ( 232.5999999999999375, -29.99999999999999645, -50.00000000000011369 ) ) ;
#8395=DIRECTION ( 'NONE',  ( 1.000000000000000000, 0.000000000000000000, -0.000000000000000000 ) ) ;
#8396=CARTESIAN_POINT ( 'NONE',  ( 229.5999999999999375, -30.48749999999999005, 98.26794919243111792 ) ) ;
#8398=ORIENTED_EDGE ( 'NONE', *, *, #6894, .F. ) ;
#8400=CARTESIAN_POINT ( 'NONE',  ( 229.5999999999999375, -33.05624999877096570, 101.7320508075688679 ) ) ;
#8401=CARTESIAN_POINT ( 'NONE',  ( 234.0999999999999375, -31.89374999877096073, -52.59807621135342970 ) ) ;
#8405=CYLINDRICAL_SURFACE ( 'NONE', #18484, 3.000000000000002665 ) ;
#8408=CARTESIAN_POINT ( 'NONE',  ( 231.0999999999999375, -33.01874999877096428, 102.5980762113533018 ) ) ;
#8409=ORIENTED_EDGE ( 'NONE', *, *, #1500, .T. ) ;
#8413=EDGE_CURVE ( 'NONE', #19103, #4556, #14411, .T. ) ;
#8421=ORIENTED_EDGE ( 'NONE', *, *, #7384, .F. ) ;
#8422=LINE ( 'NONE', #18888, #8039 ) ;
#8425=DIRECTION ( 'NONE',  ( -0.000000000000000000, -1.000000000000000000, -0.000000000000000000 ) ) ;
#8429=CARTESIAN_POINT ( 'NONE',  ( 232.5999999999999375, -31.60312499938548214, -53.18285161636690361 ) ) ;
#8436=ADVANCED_FACE ( 'NONE', ( #7371 ), #10145, .F. ) ;
#8441=CARTESIAN_POINT ( 'NONE',  ( 232.5999999999999375, -32.95312499938548001, -53.18285161636690361 ) ) ;
#8452=CARTESIAN_POINT ( 'NONE',  ( 235.3564303562499447, -32.20312499938548001, 101.5914258081833879 ) ) ;
#8457=CARTESIAN_POINT ( 'NONE',  ( 235.5999999999999375, -32.92499999999999716, 99.99999999999998579 ) ) ;
#8460=CARTESIAN_POINT ( 'NONE',  ( 246.9999999999999716, -5.000000000000004441, 150.0000000000000000 ) ) ;
#8464=VERTEX_POINT ( 'NONE', #9097 ) ;
#8466=CARTESIAN_POINT ( 'NONE',  ( 233.2099102960628443, -35.00000000000002842, -47.30603528924583401 ) ) ;
#8467=CARTESIAN_POINT ( 'NONE',  ( 235.3564303562499447, -32.31562499938547717, -48.40857419181671162 ) ) ;
#8469=FACE_OUTER_BOUND ( 'NONE', #12656, .T. ) ;
#8473=ORIENTED_EDGE ( 'NONE', *, *, #3245, .F. ) ;
#8486=CARTESIAN_POINT ( 'NONE',  ( 235.5999999999999943, -31.98749999999999361, 98.26794919243110371 ) ) ;
#8490=CARTESIAN_POINT ( 'NONE',  ( 234.0999999999999375, -32.94374999877096144, 102.5980762113533018 ) ) ;
#8491=CARTESIAN_POINT ( 'NONE',  ( 234.0999999999999375, -31.59374999877096712, -47.40192378864679768 ) ) ;
#8492=CARTESIAN_POINT ( 'NONE',  ( 231.7961524227065695, -32.55134618820330417, 103.0000000000000000 ) ) ;
#8496=VECTOR ( 'NONE', #13988, 1000.000000000000000 ) ;
#8498=CARTESIAN_POINT ( 'NONE',  ( 235.5999999999999943, -33.73124999877096286, -51.73205080756900287 ) ) ;
#8499=ORIENTED_EDGE ( 'NONE', *, *, #9274, .T. ) ;
#8502=EDGE_CURVE ( 'NONE', #9169, #3491, #229, .T. ) ;
#8513=EDGE_LOOP ( 'NONE', ( #16634, #14971, #5979, #6210 ) ) ;
#8523=CARTESIAN_POINT ( 'NONE',  ( 232.5999999999999375, -30.92812499938547433, -46.81714838363331666 ) ) ;
#8530=CARTESIAN_POINT ( 'NONE',  ( 233.9782151781249411, -30.44062499938548072, 102.3871387122750889 ) ) ;
#8532=( BOUNDED_CURVE ( )  B_SPLINE_CURVE ( 2, ( #13250, #5839, #2276, #17035, #11261, #13802, #445 ),
 .UNSPECIFIED., .F., .F. ) 
 B_SPLINE_CURVE_WITH_KNOTS ( ( 3, 2, 2, 3 ),
 ( 0.8958333333333332593, 0.9027777777777777901, 0.9166666666666666297, 0.9258785066912882389 ),
 .UNSPECIFIED. ) 
 CURVE ( )  GEOMETRIC_REPRESENTATION_ITEM ( )  RATIONAL_B_SPLINE_CURVE ( ( 0.9330127018922192983, 0.9330127018922187432, 1.000000000000000000, 0.8660254037844387076, 1.000000000000000000, 0.9111410165655264848, 0.9401539157124900736 ) ) 
 REPRESENTATION_ITEM ( '' )  );
#8537=CARTESIAN_POINT ( 'NONE',  ( 229.8435696437499303, -34.19062499938547717, -50.00000000000011369 ) ) ;
#8548=CARTESIAN_POINT ( 'NONE',  ( 233.9782151781249411, -32.99062499938548143, 97.61286128772489690 ) ) ;
#8549=CARTESIAN_POINT ( 'NONE',  ( 99.99999999999997158, -5.200000000000008171, -100.0000000000000000 ) ) ;
#8553=CARTESIAN_POINT ( 'NONE',  ( 105.1999999999999744, -29.80000000000002203, 150.0000000000000000 ) ) ;
#8556=CARTESIAN_POINT ( 'NONE',  ( 234.1999394931800396, -32.00000000000002132, 97.54622936382085641 ) ) ;
#8557=LINE ( 'NONE', #9839, #18697 ) ;
#8560=( BOUNDED_CURVE ( )  B_SPLINE_CURVE ( 2, ( #119, #19258, #6068, #4598, #12114, #9176, #9078, #7714, #10555 ),
 .UNSPECIFIED., .F., .F. ) 
 B_SPLINE_CURVE_WITH_KNOTS ( ( 3, 2, 2, 2, 3 ),
 ( 0.4374999999999999445, 0.4444444444444444198, 0.4583333333333333148, 0.4722222222222222099, 0.4791666666666665186 ),
 .UNSPECIFIED. ) 
 CURVE ( )  GEOMETRIC_REPRESENTATION_ITEM ( )  RATIONAL_B_SPLINE_CURVE ( ( 0.9330127018922192983, 0.9330127018922187432, 1.000000000000000000, 0.8660254037844387076, 1.000000000000000000, 0.8660254037844387076, 1.000000000000000000, 0.9330127018922207416, 0.9330127018922194093 ) ) 
 REPRESENTATION_ITEM ( '' )  );
#8564=CARTESIAN_POINT ( 'NONE',  ( 233.9782151781249411, -35.05312499938548143, 102.3871387122750889 ) ) ;
#8565=CARTESIAN_POINT ( 'NONE',  ( 233.9782151781249411, -34.00312499938547717, -52.38713871227520968 ) ) ;
#8567=CARTESIAN_POINT ( 'NONE',  ( 232.5999999999999659, -32.58749999999999858, -47.00000000000011369 ) ) ;
#8579=CARTESIAN_POINT ( 'NONE',  ( 0.000000000000000000, -29.80000000000002203, 153.0000000000000000 ) ) ;
#8580=VECTOR ( 'NONE', #17890, 1000.000000000000000 ) ;
#8583=CARTESIAN_POINT ( 'NONE',  ( 231.0999999999999375, -30.97499999999999432, 97.40192378864668399 ) ) ;
#8587=CARTESIAN_POINT ( 'NONE',  ( 231.0999999999999375, -32.71874999877096002, 97.40192378864668399 ) ) ;
#8588=CARTESIAN_POINT ( 'NONE',  ( 229.5999999999999375, -30.88124999877096144, -51.73205080756898866 ) ) ;
#8589=CARTESIAN_POINT ( 'NONE',  ( 232.5999999999999375, -29.99999999999999645, -53.00000000000012079 ) ) ;
#8590=EDGE_CURVE ( 'NONE', #14649, #12940, #14130, .T. ) ;
#8592=ORIENTED_EDGE ( 'NONE', *, *, #3514, .F. ) ;
#8597=ORIENTED_EDGE ( 'NONE', *, *, #15566, .T. ) ;
#8601=( BOUNDED_CURVE ( )  B_SPLINE_CURVE ( 2, ( #6925, #2421, #13154, #19125, #1153, #2807, #5743, #9850, #4273 ),
 .UNSPECIFIED., .F., .F. ) 
 B_SPLINE_CURVE_WITH_KNOTS ( ( 3, 2, 2, 2, 3 ),
 ( 0.6874999999999997780, 0.6944444444444444198, 0.7083333333333333703, 0.7222222222222222099, 0.7291666666666665186 ),
 .UNSPECIFIED. ) 
 CURVE ( )  GEOMETRIC_REPRESENTATION_ITEM ( )  RATIONAL_B_SPLINE_CURVE ( ( 0.9330127018922194093, 0.9330127018922171889, 1.000000000000000000, 0.8660254037844387076, 1.000000000000000000, 0.8660254037844387076, 1.000000000000000000, 0.9330127018922209636, 0.9330127018922194093 ) ) 
 REPRESENTATION_ITEM ( '' )  );
#8608=AXIS2_PLACEMENT_3D ( 'NONE', #15749, #10862, #5016 ) ;
#8609=CARTESIAN_POINT ( 'NONE',  ( 229.8435696437499871, -31.00312499938547361, 101.5914258081833879 ) ) ;
#8610=VERTEX_POINT ( 'NONE', #11047 ) ;
#8613=CARTESIAN_POINT ( 'NONE',  ( 233.5140320577117166, -34.99999999999999289, 97.18639806692216609 ) ) ;
#8615=CARTESIAN_POINT ( 'NONE',  ( 235.3564303562499731, -34.98839802032724577, 100.4359666841262708 ) ) ;
#8618=CARTESIAN_POINT ( 'NONE',  ( 235.3564303562499447, -31.67812499938547788, -51.59142580818350865 ) ) ;
#8624=CARTESIAN_POINT ( 'NONE',  ( 233.9782151781249411, -32.09062499938547575, 97.61286128772489690 ) ) ;
#8625=CARTESIAN_POINT ( 'NONE',  ( 233.9782151781249411, -32.54062499938547859, -52.38713871227520968 ) ) ;
#8626=LINE ( 'NONE', #10198, #10206 ) ;
#8630=CARTESIAN_POINT ( 'NONE',  ( 235.5999999999999943, -30.18749999999999289, -51.73205080756900287 ) ) ;
#8642=CARTESIAN_POINT ( 'NONE',  ( 232.5999999999999943, -33.62812499938547717, 103.1828516163667899 ) ) ;
#8652=CARTESIAN_POINT ( 'NONE',  ( 232.8516854624778318, -32.00000000000002132, 97.14155664245926403 ) ) ;
#8660=CARTESIAN_POINT ( 'NONE',  ( 229.8435696437499303, -35.20312499938548001, 99.99999999999998579 ) ) ;
#8661=CARTESIAN_POINT ( 'NONE',  ( 229.8435696437499303, -35.20312499938548001, -50.00000000000011369 ) ) ;
#8663=AXIS2_PLACEMENT_3D ( 'NONE', #6428, #12187, #16780 ) ;
#8674=CARTESIAN_POINT ( 'NONE',  ( 231.7961524227065695, -34.40759618943233988, -47.00000000000011369 ) ) ;
#8676=CARTESIAN_POINT ( 'NONE',  ( 229.8435696437499871, -31.19062499938548072, 98.40857419181659793 ) ) ;
#8684=CARTESIAN_POINT ( 'NONE',  ( 232.5999999999999659, -32.13749999999999574, -47.00000000000011369 ) ) ;
#8687=CARTESIAN_POINT ( 'NONE',  ( 234.0999999999999375, -30.59999999999999432, 97.40192378864668399 ) ) ;
#8689=DIRECTION ( 'NONE',  ( 0.000000000000000000, -3.336006684570784876E-15, -1.000000000000000000 ) ) ;
#8691=CARTESIAN_POINT ( 'NONE',  ( 229.5999999999999375, -31.78124999877096357, 98.26794919243111792 ) ) ;
#8692=CARTESIAN_POINT ( 'NONE',  ( 232.5999999999999375, -32.75624999877096144, -53.46410161513786363 ) ) ;
#8699=DIRECTION ( 'NONE',  ( 0.000000000000000000, 0.000000000000000000, -1.000000000000000000 ) ) ;
#8700=ORIENTED_EDGE ( 'NONE', *, *, #3245, .T. ) ;
#8706=CARTESIAN_POINT ( 'NONE',  ( 232.5999999999999659, -32.53124999877096712, -47.00000000000011369 ) ) ;
#8709=ORIENTED_EDGE ( 'NONE', *, *, #2920, .T. ) ;
#8711=CARTESIAN_POINT ( 'NONE',  ( 233.4038475772933339, -32.38259618943233420, -53.00000000000011369 ) ) ;
#8716=CARTESIAN_POINT ( 'NONE',  ( 233.9782151781249411, -33.14062499938548001, -47.61286128772501769 ) ) ;
#8717=( BOUNDED_CURVE ( )  B_SPLINE_CURVE ( 2, ( #7408, #9159, #9253, #11901, #13371, #17873, #16687, #18068, #100 ),
 .UNSPECIFIED., .F., .F. ) 
 B_SPLINE_CURVE_WITH_KNOTS ( ( 3, 2, 2, 2, 3 ),
 ( 0.5208333333333331483, 0.5277777777777777901, 0.5416666666666666297, 0.5555555555555555802, 0.5625000000000001110 ),
 .UNSPECIFIED. ) 
 CURVE ( )  GEOMETRIC_REPRESENTATION_ITEM ( )  RATIONAL_B_SPLINE_CURVE ( ( 0.9330127018922194093, 0.9330127018922177440, 1.000000000000000000, 0.8660254037844387076, 1.000000000000000000, 0.8660254037844387076, 1.000000000000000000, 0.9330127018922182991, 0.9330127018922194093 ) ) 
 REPRESENTATION_ITEM ( '' )  );
#8718=ORIENTED_EDGE ( 'NONE', *, *, #13559, .F. ) ;
#8725=CARTESIAN_POINT ( 'NONE',  ( 235.3564303562499447, -31.75312499938547717, 101.5914258081833879 ) ) ;
#8726=CARTESIAN_POINT ( 'NONE',  ( 231.2217848218749339, -34.11562499938548143, -47.61286128772501769 ) ) ;
#8730=CARTESIAN_POINT ( 'NONE',  ( 231.0999999999999375, -30.52499999999999503, -52.59807621135342970 ) ) ;
#8734=CARTESIAN_POINT ( 'NONE',  ( 105.1999999999999602, -29.80000000000001492, -97.80000000000002558 ) ) ;
#8736=CARTESIAN_POINT ( 'NONE',  ( 235.3564303562499447, -31.82812499938547646, -50.00000000000011369 ) ) ;
#8738=VERTEX_POINT ( 'NONE', #902 ) ;
#8741=DIRECTION ( 'NONE',  ( 0.000000000000000000, 0.000000000000000000, -1.000000000000000000 ) ) ;
#8747=CARTESIAN_POINT ( 'NONE',  ( 230.7036604445367232, -32.00000000000000711, -47.97042480180352442 ) ) ;
#8759=CARTESIAN_POINT ( 'NONE',  ( 230.4884461346514968, -35.25364837475780178, -51.77179247729210942 ) ) ;
#8764=EDGE_CURVE ( 'NONE', #7775, #14052, #7140, .T. ) ;
#8768=ORIENTED_EDGE ( 'NONE', *, *, #10557, .F. ) ;
#8774=CARTESIAN_POINT ( 'NONE',  ( 233.9782151781249411, -31.30312499938547788, 97.61286128772489690 ) ) ;
#8777=DIRECTION ( 'NONE',  ( 0.000000000000000000, -1.000000000000000000, 3.597944987211154374E-15 ) ) ;
#8778=CARTESIAN_POINT ( 'NONE',  ( 229.5999999999999375, -32.21249999999999858, -48.26794919243123161 ) ) ;
#8780=CARTESIAN_POINT ( 'NONE',  ( 229.5999999999999375, -34.53749999999999432, 98.26794919243111792 ) ) ;
#8782=CARTESIAN_POINT ( 'NONE',  ( 233.4038475772933339, -34.57634618820330275, 97.00000000000000000 ) ) ;
#8783=CARTESIAN_POINT ( 'NONE',  ( 235.5999999999999375, -33.76874999877096428, 99.99999999999998579 ) ) ;
#8784=CARTESIAN_POINT ( 'NONE',  ( 229.5999999999999375, -33.05624999877096570, -48.26794919243123161 ) ) ;
#8787=ORIENTED_EDGE ( 'NONE', *, *, #15792, .F. ) ;
#8790=ORIENTED_EDGE ( 'NONE', *, *, #7384, .T. ) ;
#8804=CARTESIAN_POINT ( 'NONE',  ( 231.2217848218749339, -30.21562499938547575, 97.61286128772489690 ) ) ;
#8810=CARTESIAN_POINT ( 'NONE',  ( 233.4038475772933339, -33.91740381056766296, 103.0000000000000000 ) ) ;
#8814=CARTESIAN_POINT ( 'NONE',  ( 229.8435696437499871, -31.90312499938547575, -48.40857419181671162 ) ) ;
#8821=DIRECTION ( 'NONE',  ( -1.000000000000000000, 0.000000000000000000, 0.000000000000000000 ) ) ;
#8823=CARTESIAN_POINT ( 'NONE',  ( 233.9782151781249411, -31.34062499938548285, 102.3871387122750889 ) ) ;
#8825=CARTESIAN_POINT ( 'NONE',  ( 235.3564303562499447, -33.10312499938547859, -48.40857419181671162 ) ) ;
#8828=CARTESIAN_POINT ( 'NONE',  ( 232.5999999999999375, -30.11249999999999716, -53.46410161513786363 ) ) ;
#8833=CARTESIAN_POINT ( 'NONE',  ( 232.5999999999999375, -32.98124999877095576, 102.9999999999999858 ) ) ;
#8834=CARTESIAN_POINT ( 'NONE',  ( 229.8435696437499871, -30.74062499938547433, -51.59142580818350865 ) ) ;
#8835=CIRCLE ( 'NONE', #12014, 5.199999999999996625 ) ;
#8839=CARTESIAN_POINT ( 'NONE',  ( 231.2217848218749339, -32.76562499938548001, 102.3871387122750889 ) ) ;
#8840=DIRECTION ( 'NONE',  ( 0.000000000000000000, -0.000000000000000000, -1.000000000000000000 ) ) ;
#8845=CARTESIAN_POINT ( 'NONE',  ( 229.8377951939094714, -35.00000000000000711, 98.91314642826759496 ) ) ;
#8855=ADVANCED_FACE ( 'NONE', ( #7421 ), #4302, .T. ) ;
#8860=FACE_OUTER_BOUND ( 'NONE', #17130, .T. ) ;
#8864=CARTESIAN_POINT ( 'NONE',  ( 235.3564303562499447, -30.89062499938548001, 98.40857419181659793 ) ) ;
#8868=CARTESIAN_POINT ( 'NONE',  ( 99.99999999999997158, -5.200000000000008171, -100.0000000000000000 ) ) ;
#8872=CARTESIAN_POINT ( 'NONE',  ( 235.5999999999999375, -34.27499999999999147, 99.99999999999998579 ) ) ;
#8875=CARTESIAN_POINT ( 'NONE',  ( 233.9782151781249411, -30.40312499938547930, 97.61286128772489690 ) ) ;
#8876=CARTESIAN_POINT ( 'NONE',  ( 235.5999999999999943, -34.63124999877096144, -51.73205080756900287 ) ) ;
#8880=ORIENTED_EDGE ( 'NONE', *, *, #16819, .F. ) ;
#8883=CARTESIAN_POINT ( 'NONE',  ( 244.7999999999999545, -35.00000000000000000, -100.0000000000000000 ) ) ;
#8885=ORIENTED_EDGE ( 'NONE', *, *, #14777, .F. ) ;
#8887=CARTESIAN_POINT ( 'NONE',  ( 229.5999999999999375, -33.99374999877096570, 99.99999999999998579 ) ) ;
#8895=CARTESIAN_POINT ( 'NONE',  ( 235.3564303562499447, -30.81562499938547717, 99.99999999999998579 ) ) ;
#8900=FACE_OUTER_BOUND ( 'NONE', #18773, .T. ) ;
#8901=CARTESIAN_POINT ( 'NONE',  ( 231.0999999999999375, -34.51874999877096428, 97.40192378864668399 ) ) ;
#8904=CARTESIAN_POINT ( 'NONE',  ( 235.3564303562499447, -33.47812499938547148, -51.59142580818350865 ) ) ;
#8905=VERTEX_POINT ( 'NONE', #16127 ) ;
#8914=CARTESIAN_POINT ( 'NONE',  ( 229.8435696437499871, -33.32812499938548001, 98.40857419181659793 ) ) ;
#8916=CARTESIAN_POINT ( 'NONE',  ( 229.8435696437499587, -33.32812499938548001, -51.59142580818350154 ) ) ;
#8919=ORIENTED_EDGE ( 'NONE', *, *, #16427, .F. ) ;
#8920=CARTESIAN_POINT ( 'NONE',  ( 235.5999999999999943, -30.26249999999999218, -48.26794919243124582 ) ) ;
#8926=CARTESIAN_POINT ( 'NONE',  ( 233.9782151781249411, -31.75312499938547717, -52.38713871227520968 ) ) ;
#8927=AXIS2_PLACEMENT_3D ( 'NONE', #15610, #9741, #5063 ) ;
#8931=CARTESIAN_POINT ( 'NONE',  ( 231.7960411235079050, -35.00000000000002132, 102.6365808225362883 ) ) ;
#8954=PLANE ( 'NONE',  #4223 ) ;
#8959=CARTESIAN_POINT ( 'NONE',  ( 235.3564303562499447, -32.27812499938548285, 99.99999999999998579 ) ) ;
#8961=AXIS2_PLACEMENT_3D ( 'NONE', #13300, #14863, #1588 ) ;
#8970=CARTESIAN_POINT ( 'NONE',  ( 235.5999999999999943, -33.33749999999999147, 98.26794919243110371 ) ) ;
#8972=CARTESIAN_POINT ( 'NONE',  ( 229.8435696437499303, -33.85312499938548569, -50.00000000000011369 ) ) ;
#8974=CARTESIAN_POINT ( 'NONE',  ( 234.0999999999999375, -34.59374999877096002, 97.40192378864668399 ) ) ;
#8975=CARTESIAN_POINT ( 'NONE',  ( 235.5999999999999943, -33.73124999877096286, -51.73205080756900287 ) ) ;
#8977=CIRCLE ( 'NONE', #2121, 5.199999999999996625 ) ;
#8986=AXIS2_PLACEMENT_3D ( 'NONE', #4643, #19100, #4535 ) ;
#8993=EDGE_CURVE ( 'NONE', #12080, #12231, #6063, .T. ) ;
#8995=CARTESIAN_POINT ( 'NONE',  ( 233.4038475772933339, -33.28259618943232567, 96.99999999999998579 ) ) ;
#8999=VERTEX_POINT ( 'NONE', #12009 ) ;
#9000=FILL_AREA_STYLE ('',( #1958 ) ) ;
#9004=CARTESIAN_POINT ( 'NONE',  ( 235.5999999999999943, -34.63124999877096144, -51.73205080756900287 ) ) ;
#9008=CARTESIAN_POINT ( 'NONE',  ( 235.3564303562499447, -32.61562499938548143, -50.00000000000011369 ) ) ;
#9014=EDGE_CURVE ( 'NONE', #10754, #8256, #1438, .T. ) ;
#9018=CARTESIAN_POINT ( 'NONE',  ( 231.2217848218749339, -34.56562499938547717, 102.3871387122750889 ) ) ;
#9019=CARTESIAN_POINT ( 'NONE',  ( 233.9782151781249411, -34.79062499938547859, -52.38713871227520968 ) ) ;
#9023=VERTEX_POINT ( 'NONE', #4689 ) ;
#9024=CARTESIAN_POINT ( 'NONE',  ( 231.0999999999999375, -30.97499999999999432, -52.59807621135342970 ) ) ;
#9032=CARTESIAN_POINT ( 'NONE',  ( 235.3564303562499447, -34.82812499938548001, 98.40857419181659793 ) ) ;
#9038=CARTESIAN_POINT ( 'NONE',  ( 229.6750025474186998, -35.00000000000000711, 99.84129707245845964 ) ) ;
#9042=CARTESIAN_POINT ( 'NONE',  ( 231.7961524227065979, -33.24240381056766580, -53.00000000000011369 ) ) ;
#9045=ORIENTED_EDGE ( 'NONE', *, *, #1723, .T. ) ;
#9057=CARTESIAN_POINT ( 'NONE',  ( 233.9782151781249411, -31.90312499938548285, 102.3871387122750889 ) ) ;
#9060=CARTESIAN_POINT ( 'NONE',  ( 233.4038475772933339, -33.86115380933863150, 102.9999999999999858 ) ) ;
#9065=CARTESIAN_POINT ( 'NONE',  ( 229.5999999999999375, -33.18749999999999289, 98.26794919243111792 ) ) ;
#9067=CARTESIAN_POINT ( 'NONE',  ( 232.5999999999999943, -32.61562499938548143, -53.18285161636690361 ) ) ;
#9069=CARTESIAN_POINT ( 'NONE',  ( 229.8435696437499871, -31.19062499938548072, 98.40857419181659793 ) ) ;
#9070=CARTESIAN_POINT ( 'NONE',  ( 232.5999999999999375, -33.20624999877095718, -53.46410161513786363 ) ) ;
#9073=ORIENTED_EDGE ( 'NONE', *, *, #9358, .F. ) ;
#9078=CARTESIAN_POINT ( 'NONE',  ( 234.0999999999999375, -32.54999999999999716, 102.5980762113533018 ) ) ;
#9082=LINE ( 'NONE', #12121, #10071 ) ;
#9088=CARTESIAN_POINT ( 'NONE',  ( 229.8435696437499303, -31.94062499938547717, 99.99999999999998579 ) ) ;
#9090=SURFACE_SIDE_STYLE ('',( #12129 ) ) ;
#9097=CARTESIAN_POINT ( 'NONE',  ( 244.7999999999999545, -4.999999999999976907, 153.0000000000000000 ) ) ;
#9106=DIRECTION ( 'NONE',  ( 4.625929269271485174E-17, 1.000000000000000000, -0.000000000000000000 ) ) ;
#9107=CARTESIAN_POINT ( 'NONE',  ( 235.3564303562499447, -34.86562499938547433, 99.99999999999998579 ) ) ;
#9115=CARTESIAN_POINT ( 'NONE',  ( 232.5999999999999375, -33.03749999999999432, -46.53589838486234953 ) ) ;
#9119=FACE_OUTER_BOUND ( 'NONE', #15157, .T. ) ;
#9120=CARTESIAN_POINT ( 'NONE',  ( 235.3564303562499447, -30.96562499938547930, -48.40857419181671162 ) ) ;
#9134=CARTESIAN_POINT ( 'NONE',  ( 229.8435696437499303, -31.49062499938547788, -50.00000000000011369 ) ) ;
#9151=CARTESIAN_POINT ( 'NONE',  ( 232.5999999999999375, -34.41562499938547859, 96.81714838363319586 ) ) ;
#9158=( BOUNDED_CURVE ( )  B_SPLINE_CURVE ( 2, ( #18094, #8995, #125, #17993, #4704, #10651, #16618, #9474, #6556 ),
 .UNSPECIFIED., .F., .F. ) 
 B_SPLINE_CURVE_WITH_KNOTS ( ( 3, 2, 2, 2, 3 ),
 ( 0.6041666666666667407, 0.6111111111111111605, 0.6250000000000000000, 0.6388888888888888395, 0.6458333333333332593 ),
 .UNSPECIFIED. ) 
 CURVE ( )  GEOMETRIC_REPRESENTATION_ITEM ( )  RATIONAL_B_SPLINE_CURVE ( ( 0.9330127018922192983, 0.9330127018922198534, 1.000000000000000000, 0.8660254037844387076, 1.000000000000000000, 0.8660254037844387076, 1.000000000000000000, 0.9330127018922198534, 0.9330127018922192983 ) ) 
 REPRESENTATION_ITEM ( '' )  );
#9159=CARTESIAN_POINT ( 'NONE',  ( 233.4038475772932770, -33.22634618820329422, 96.99999999999997158 ) ) ;
#9161=CARTESIAN_POINT ( 'NONE',  ( 229.5999999999999375, -32.73749999999999716, 98.26794919243111792 ) ) ;
#9163=CARTESIAN_POINT ( 'NONE',  ( 231.2217848218749339, -33.77812499938547575, -47.61286128772501769 ) ) ;
#9165=CARTESIAN_POINT ( 'NONE',  ( 235.3564303562499447, -30.92812499938547788, 99.99999999999998579 ) ) ;
#9166=CARTESIAN_POINT ( 'NONE',  ( 235.5999999999999375, -35.11874999877095860, -50.00000000000011369 ) ) ;
#9169=VERTEX_POINT ( 'NONE', #4423 ) ;
#9172=CARTESIAN_POINT ( 'NONE',  ( 232.5999999999999375, -34.83749999999999147, 103.0000000000000000 ) ) ;
#9175=DIRECTION ( 'NONE',  ( -1.000000000000000000, 0.000000000000000000, 0.000000000000000000 ) ) ;
#9176=CARTESIAN_POINT ( 'NONE',  ( 235.5999999999999943, -32.51249999999999574, 101.7320508075688537 ) ) ;
#9183=FACE_OUTER_BOUND ( 'NONE', #11222, .T. ) ;
#9185=CARTESIAN_POINT ( 'NONE',  ( 231.2217848218749339, -32.01562499938548001, 97.61286128772489690 ) ) ;
#9186=ORIENTED_EDGE ( 'NONE', *, *, #8215, .F. ) ;
#9190=CARTESIAN_POINT ( 'NONE',  ( 234.0999999999999375, -33.89999999999999147, 102.5980762113533018 ) ) ;
#9192=CARTESIAN_POINT ( 'NONE',  ( 229.6750025474185009, -35.00000000000002132, -50.15870292752263282 ) ) ;
#9194=ORIENTED_EDGE ( 'NONE', *, *, #539, .F. ) ;
#9195=ORIENTED_EDGE ( 'NONE', *, *, #7612, .F. ) ;
#9200=PLANE ( 'NONE',  #19294 ) ;
#9201=CARTESIAN_POINT ( 'NONE',  ( 229.8435696437499871, -32.87812499938547717, 98.40857419181659793 ) ) ;
#9206=CARTESIAN_POINT ( 'NONE',  ( 229.5999999999999375, -33.60000000000000142, -50.00000000000011369 ) ) ;
#9211=CARTESIAN_POINT ( 'NONE',  ( 233.9782151781249411, -34.00312499938547717, -52.38713871227520968 ) ) ;
#9215=ADVANCED_FACE ( 'NONE', ( #13210 ), #17912, .F. ) ;
#9217=CARTESIAN_POINT ( 'NONE',  ( 229.8435696437499303, -34.64062499938548001, 99.99999999999998579 ) ) ;
#9220=CARTESIAN_POINT ( 'NONE',  ( 230.5523683116323355, -32.00000000000000000, -48.15470523285603832 ) ) ;
#9226=CARTESIAN_POINT ( 'NONE',  ( 231.2217848218749339, -30.66562499938547859, -52.38713871227520968 ) ) ;
#9231=EDGE_LOOP ( 'NONE', ( #1130, #11631, #16100, #14383 ) ) ;
#9246=CARTESIAN_POINT ( 'NONE',  ( 235.3564303562499447, -34.07812499938548001, 99.99999999999998579 ) ) ;
#9249=CARTESIAN_POINT ( 'NONE',  ( 105.1999999999999886, -34.99999999999999289, -97.80000000000002558 ) ) ;
#9253=CARTESIAN_POINT ( 'NONE',  ( 234.0999999999999375, -33.24374999877096570, 97.40192378864668399 ) ) ;
#9257=ORIENTED_EDGE ( 'NONE', *, *, #11545, .T. ) ;
#9258=CARTESIAN_POINT ( 'NONE',  ( 229.8435696437499303, -32.50312499938547717, -50.00000000000011369 ) ) ;
#9260=CARTESIAN_POINT ( 'NONE',  ( 235.5999999999999375, -35.11874999877095860, 99.99999999999998579 ) ) ;
#9261=CARTESIAN_POINT ( 'NONE',  ( 233.9782151781249411, -31.45312499938548356, -47.61286128772501769 ) ) ;
#9262=VECTOR ( 'NONE', #7695, 1000.000000000000000 ) ;
#9267=CARTESIAN_POINT ( 'NONE',  ( 232.5999999999999091, -33.03749999999998721, 102.9999999999999858 ) ) ;
#9270=CARTESIAN_POINT ( 'NONE',  ( 105.1999999999999744, -31.99999999999999289, -100.0000000000000000 ) ) ;
#9274=EDGE_CURVE ( 'NONE', #13854, #2849, #2065, .T. ) ;
#9276=VECTOR ( 'NONE', #6220, 1000.000000000000000 ) ;
#9277=CARTESIAN_POINT ( 'NONE',  ( 232.5999999999999375, -32.36249999999999716, 97.00000000000000000 ) ) ;
#9282=CARTESIAN_POINT ( 'NONE',  ( 229.8435696437499871, -32.35312499938547859, 101.5914258081833879 ) ) ;
#9286=ORIENTED_EDGE ( 'NONE', *, *, #2917, .T. ) ;
#9289=CARTESIAN_POINT ( 'NONE',  ( 232.5999999999999375, -29.99999999999999645, -50.00000000000011369 ) ) ;
#9290=CARTESIAN_POINT ( 'NONE',  ( 230.4884518427504076, -35.14114861271050216, -51.77179927996177611 ) ) ;
#9292=VECTOR ( 'NONE', #14479, 1000.000000000000000 ) ;
#9295=CARTESIAN_POINT ( 'NONE',  ( 232.5999999999999375, -29.99999999999999645, -50.00000000000011369 ) ) ;
#9301=CARTESIAN_POINT ( 'NONE',  ( 233.9782151781249411, -32.99062499938548143, 97.61286128772489690 ) ) ;
#9308=CARTESIAN_POINT ( 'NONE',  ( 232.5999999999999375, -31.46249999999999858, -53.46410161513786363 ) ) ;
#9313=CARTESIAN_POINT ( 'NONE',  ( 229.8435696437499871, -34.34062499938547575, -51.59142580818350865 ) ) ;
#9319=CARTESIAN_POINT ( 'NONE',  ( 232.5999999999999375, -34.61249999999999716, 97.00000000000000000 ) ) ;
#9324=CARTESIAN_POINT ( 'NONE',  ( 232.5999999999999375, -31.82812499938547290, -46.81714838363331666 ) ) ;
#9330=( LENGTH_UNIT ( ) NAMED_UNIT ( * ) SI_UNIT ( .MILLI., .METRE. ) );
#9332=CARTESIAN_POINT ( 'NONE',  ( 235.5999999999999943, -32.06249999999999289, -48.26794919243124582 ) ) ;
#9333=ORIENTED_EDGE ( 'NONE', *, *, #3518, .T. ) ;
#9337=EDGE_CURVE ( 'NONE', #11694, #4350, #5199, .T. ) ;
#9341=CARTESIAN_POINT ( 'NONE',  ( 233.4038475772933054, -32.96115380933862582, -47.00000000000010658 ) ) ;
#9342=CARTESIAN_POINT ( 'NONE',  ( 231.2217848218749339, -34.22812499938548569, 102.3871387122750889 ) ) ;
#9344=VERTEX_POINT ( 'NONE', #8226 ) ;
#9347=CARTESIAN_POINT ( 'NONE',  ( 229.8538686580537842, -31.99999999999998579, 99.70214005991812201 ) ) ;
#9351=DIRECTION ( 'NONE',  ( -0.000000000000000000, -1.000000000000000000, -0.000000000000000000 ) ) ;
#9352=EDGE_CURVE ( 'NONE', #8610, #3766, #5594, .T. ) ;
#9354=CARTESIAN_POINT ( 'NONE',  ( 233.9782151781249411, -32.20312499938548001, -52.38713871227520968 ) ) ;
#9357=CARTESIAN_POINT ( 'NONE',  ( 229.8435696437499871, -32.01562499938548001, 101.5914258081833879 ) ) ;
#9358=EDGE_CURVE ( 'NONE', #12231, #927, #8835, .T. ) ;
#9359=CARTESIAN_POINT ( 'NONE',  ( 235.5999999999999943, -35.15624999877096002, -48.26794919243124582 ) ) ;
#9372=DIRECTION ( 'NONE',  ( -0.000000000000000000, 0.000000000000000000, 1.000000000000000000 ) ) ;
#9374=CARTESIAN_POINT ( 'NONE',  ( 229.8435696437499587, -35.11426541925032296, 98.99674735228809652 ) ) ;
#9375=CARTESIAN_POINT ( 'NONE',  ( 232.5999999999999375, -31.82812499938547290, 103.1828516163667899 ) ) ;
#9377=CARTESIAN_POINT ( 'NONE',  ( 229.5999999999999375, -30.39374999877096428, 99.99999999999998579 ) ) ;
#9380=DIRECTION ( 'NONE',  ( 0.000000000000000000, 0.000000000000000000, 1.000000000000000000 ) ) ;
#9385=CARTESIAN_POINT ( 'NONE',  ( 229.5999999999999375, -33.50624999877096144, 101.7320508075688821 ) ) ;
#9403=ORIENTED_EDGE ( 'NONE', *, *, #14251, .F. ) ;
#9404=CARTESIAN_POINT ( 'NONE',  ( 234.0999999999999375, -32.09999999999999432, -47.40192378864679768 ) ) ;
#9405=CARTESIAN_POINT ( 'NONE',  ( 232.5999999999999091, -34.38749999999999574, 102.9999999999999858 ) ) ;
#9409=CARTESIAN_POINT ( 'NONE',  ( 233.9782151781249411, -32.65312499938548285, -52.38713871227520968 ) ) ;
#9411=ORIENTED_EDGE ( 'NONE', *, *, #11727, .T. ) ;
#9416=CARTESIAN_POINT ( 'NONE',  ( 234.0999999999999375, -34.79999999999999716, 102.5980762113533018 ) ) ;
#9422=CARTESIAN_POINT ( 'NONE',  ( 233.4038475772933054, -33.01740381056766438, -47.00000000000009237 ) ) ;
#9427=EDGE_CURVE ( 'NONE', #19103, #3788, #12712, .T. ) ;
#9433=CARTESIAN_POINT ( 'NONE',  ( 235.4117376914898898, -32.00000000000000000, -51.04600724388262023 ) ) ;
#9439=CARTESIAN_POINT ( 'NONE',  ( 235.3564303562499447, -33.17812499938548143, 99.99999999999998579 ) ) ;
#9441=ORIENTED_EDGE ( 'NONE', *, *, #18735, .F. ) ;
#9453=CARTESIAN_POINT ( 'NONE',  ( 235.3564303562499447, -31.79062499938547859, 98.40857419181659793 ) ) ;
#9454=CARTESIAN_POINT ( 'NONE',  ( 229.5999999999999375, -35.30624999877095860, -48.26794919243123161 ) ) ;
#9457=CARTESIAN_POINT ( 'NONE',  ( 233.4038475772933339, -34.63259618943233420, -53.00000000000009948 ) ) ;
#9459=ORIENTED_EDGE ( 'NONE', *, *, #7442, .F. ) ;
#9461=DIRECTION ( 'NONE',  ( -0.000000000000000000, -1.000000000000000000, -0.000000000000000000 ) ) ;
#9473=CARTESIAN_POINT ( 'NONE',  ( 232.5999999999999375, -33.88124999877096855, -47.00000000000011369 ) ) ;
#9474=CARTESIAN_POINT ( 'NONE',  ( 233.4038475772933339, -33.46740381056766012, 102.9999999999999716 ) ) ;
#9475=CARTESIAN_POINT ( 'NONE',  ( 229.8435696437499303, -34.64062499938548001, 99.99999999999998579 ) ) ;
#9482=DIRECTION ( 'NONE',  ( 1.788378118793198438E-31, 3.597944987211154374E-15, 1.000000000000000000 ) ) ;
#9485=CARTESIAN_POINT ( 'NONE',  ( 232.5999999999999375, -34.97812499938547859, -46.81714838363331666 ) ) ;
#9501=ORIENTED_EDGE ( 'NONE', *, *, #15830, .T. ) ;
#9502=CARTESIAN_POINT ( 'NONE',  ( 235.5999999999999375, -32.02499999999999858, -50.00000000000011369 ) ) ;
#9506=CARTESIAN_POINT ( 'NONE',  ( 231.2217848218749339, -33.47812499938547859, 97.61286128772489690 ) ) ;
#9509=CARTESIAN_POINT ( 'NONE',  ( 229.8435696437499303, -33.85312499938548569, -50.00000000000011369 ) ) ;
#9517=CARTESIAN_POINT ( 'NONE',  ( 233.4038475772933339, -34.81740381056766154, 102.9999999999999716 ) ) ;
#9523=CARTESIAN_POINT ( 'NONE',  ( 231.2217848218749339, -30.21562499938547575, -52.38713871227520968 ) ) ;
#9529=CIRCLE ( 'NONE', #12029, 5.199999999999996625 ) ;
#9538=CARTESIAN_POINT ( 'NONE',  ( 235.3564303562499447, -33.21562499938548285, 101.5914258081833879 ) ) ;
#9545=VECTOR ( 'NONE', #15285, 1000.000000000000000 ) ;
#9552=CARTESIAN_POINT ( 'NONE',  ( 235.3564303562499447, -32.31562499938547717, 101.5914258081833879 ) ) ;
#9553=CARTESIAN_POINT ( 'NONE',  ( 235.3564303562499447, -31.86562499938547788, -48.40857419181671162 ) ) ;
#9570=CARTESIAN_POINT ( 'NONE',  ( 232.3466685930879123, -34.99995246259152282, 97.01071553687879145 ) ) ;
#9573=CARTESIAN_POINT ( 'NONE',  ( 235.3564303562499447, -33.47812499938547148, 98.40857419181659793 ) ) ;
#9574=ORIENTED_EDGE ( 'NONE', *, *, #17389, .F. ) ;
#9578=CARTESIAN_POINT ( 'NONE',  ( 231.7961524227065695, -32.10134618820329422, 102.9999999999999716 ) ) ;
#9579=EDGE_LOOP ( 'NONE', ( #9501, #18079, #12400, #4231, #11243, #12578 ) ) ;
#9581=LINE ( 'NONE', #18478, #7727 ) ;
#9582=MECHANICAL_DESIGN_GEOMETRIC_PRESENTATION_REPRESENTATION('',(#17704),#3343);
#9588=VERTEX_POINT ( 'NONE', #10271 ) ;
#9592=VECTOR ( 'NONE', #13351, 1000.000000000000000 ) ;
#9593=EDGE_CURVE ( 'NONE', #484, #17889, #16232, .T. ) ;
#9599=VECTOR ( 'NONE', #13586, 1000.000000000000000 ) ;
#9604=CARTESIAN_POINT ( 'NONE',  ( 234.9136945297046282, -32.02340763552835057, -47.87171054440991469 ) ) ;
#9612=CARTESIAN_POINT ( 'NONE',  ( 229.8435696437499871, -32.46562499938548285, -48.40857419181671162 ) ) ;
#9615=B_SPLINE_CURVE_WITH_KNOTS ( 'NONE', 3,
 ( #18042, #16569, #14606, #1237, #7189, #13138, #2794, #19112, #19314, #5925, #7379, #13237, #11871, #11681, #5732, #17838, #8747, #14699 ),
 .UNSPECIFIED., .F., .F.,
 ( 4, 2, 2, 2, 2, 2, 2, 2, 4 ),
 ( 0.000000000000000000, 0.0007106627595359796094, 0.001421325519071959219, 0.002131988278607938828, 0.002842651038143918438, 0.003553313797679898047, 0.004263976557215877657, 0.004974639316751856832, 0.005685302076287836875 ),
 .UNSPECIFIED. ) ;
#9622=CARTESIAN_POINT ( 'NONE',  ( 232.5999999999999375, -34.83749999999999147, 103.0000000000000000 ) ) ;
#9627=CARTESIAN_POINT ( 'NONE',  ( 229.8435696437499303, -33.29062499938547148, -50.00000000000011369 ) ) ;
#9645=CARTESIAN_POINT ( 'NONE',  ( 235.3564303562499447, -32.12812499938547717, 98.40857419181659793 ) ) ;
#9650=PLANE ( 'NONE',  #8927 ) ;
#9658=CARTESIAN_POINT ( 'NONE',  ( 235.3564303562499447, -31.41562499938548214, 101.5914258081833879 ) ) ;
#9659=CARTESIAN_POINT ( 'NONE',  ( 232.5999999999999375, -33.29062499938547859, -46.81714838363331666 ) ) ;
#9666=ORIENTED_EDGE ( 'NONE', *, *, #11037, .T. ) ;
#9674=CARTESIAN_POINT ( 'NONE',  ( 231.0999999999999375, -34.06874999877096144, -52.59807621135342970 ) ) ;
#9676=CARTESIAN_POINT ( 'NONE',  ( 235.3564303562499447, -33.10312499938547859, 101.5914258081833879 ) ) ;
#9679=CARTESIAN_POINT ( 'NONE',  ( 235.5999999999999943, -31.48124999877096286, 98.26794919243110371 ) ) ;
#9680=CARTESIAN_POINT ( 'NONE',  ( 235.5999999999999943, -31.55624999877096215, -48.26794919243124582 ) ) ;
#9683=PLANE ( 'NONE',  #17089 ) ;
#9686=CARTESIAN_POINT ( 'NONE',  ( 231.7961524227065979, -33.63615380933863008, 97.00000000000000000 ) ) ;
#9691=CARTESIAN_POINT ( 'NONE',  ( 105.1999999999999744, -31.99999999999999289, 150.0000000000000000 ) ) ;
#9694=CARTESIAN_POINT ( 'NONE',  ( 232.8256241621686797, -34.99999999999999289, -52.98025757954786741 ) ) ;
#9704=EDGE_CURVE ( 'NONE', #15031, #13758, #10152, .T. ) ;
#9706=CARTESIAN_POINT ( 'NONE',  ( 232.5999999999999943, -32.16562499938547859, 96.81714838363319586 ) ) ;
#9708=CARTESIAN_POINT ( 'NONE',  ( 229.8435696437499871, -34.71562499938548285, -48.40857419181671162 ) ) ;
#9715=CARTESIAN_POINT ( 'NONE',  ( 233.9782151781249411, -32.99062499938548143, -52.38713871227520968 ) ) ;
#9720=CARTESIAN_POINT ( 'NONE',  ( 233.9782151781249411, -32.24062499938548143, -47.61286128772501769 ) ) ;
#9728=LINE ( 'NONE', #18525, #13014 ) ;
#9730=DIRECTION ( 'NONE',  ( 0.000000000000000000, 0.000000000000000000, 1.000000000000000000 ) ) ;
#9736=CARTESIAN_POINT ( 'NONE',  ( 231.0999999999999375, -34.12499999999999289, -52.59807621135342970 ) ) ;
#9741=DIRECTION ( 'NONE',  ( -0.000000000000000000, 0.000000000000000000, -1.000000000000000000 ) ) ;
#9743=CARTESIAN_POINT ( 'NONE',  ( 234.0999999999999375, -32.04374999877096286, 102.5980762113533018 ) ) ;
#9750=CARTESIAN_POINT ( 'NONE',  ( 231.2217848218749339, -33.02812499938547575, 97.61286128772489690 ) ) ;
#9751=CARTESIAN_POINT ( 'NONE',  ( 229.8435696437499871, -33.89062499938548001, -51.59142580818350865 ) ) ;
#9754=EDGE_LOOP ( 'NONE', ( #6230, #10638, #19180, #8718, #16718 ) ) ;
#9758=ORIENTED_EDGE ( 'NONE', *, *, #13051, .T. ) ;
#9761=AXIS2_PLACEMENT_3D ( 'NONE', #10939, #18378, #605 ) ;
#9768=DIRECTION ( 'NONE',  ( 1.000000000000000000, 0.000000000000000000, 0.000000000000000000 ) ) ;
#9770=CARTESIAN_POINT ( 'NONE',  ( 229.5999999999999375, -31.34999999999999432, 99.99999999999998579 ) ) ;
#9771=EDGE_LOOP ( 'NONE', ( #17474, #14881, #8162, #14771 ) ) ;
#9776=CARTESIAN_POINT ( 'NONE',  ( 229.5999999999999375, -31.74374999877096215, -50.00000000000011369 ) ) ;
#9780=CARTESIAN_POINT ( 'NONE',  ( 235.2218879900010791, -34.99999999999999289, 100.8506536761482124 ) ) ;
#9781=ORIENTED_EDGE ( 'NONE', *, *, #1639, .F. ) ;
#9790=UNCERTAINTY_MEASURE_WITH_UNIT (LENGTH_MEASURE( 1.000000000000000082E-05 ), #9330, 'distance_accuracy_value', 'NONE');
#9791=CARTESIAN_POINT ( 'NONE',  ( -2.962450405966101950E-15, -29.79999999999996163, -103.0000000000000142 ) ) ;
#9792=CARTESIAN_POINT ( 'NONE',  ( 231.7961524227065411, -33.05759618943232425, 102.9999999999999858 ) ) ;
#9799=LINE ( 'NONE', #13016, #10225 ) ;
#9801=CARTESIAN_POINT ( 'NONE',  ( 229.8435696437499303, -34.75312499938547717, 99.99999999999998579 ) ) ;
#9803=CARTESIAN_POINT ( 'NONE',  ( 229.8435696437499303, -31.04062499938547859, -50.00000000000011369 ) ) ;
#9816=CARTESIAN_POINT ( 'NONE',  ( 232.5999999999999375, -33.85312499938547859, -53.18285161636690361 ) ) ;
#9832=EDGE_CURVE ( 'NONE', #5766, #14052, #4799, .T. ) ;
#9835=CARTESIAN_POINT ( 'NONE',  ( 234.0999999999999375, -32.99999999999999289, 102.5980762113533018 ) ) ;
#9836=DIRECTION ( 'NONE',  ( -4.625929269271485791E-17, -1.000000000000000000, 0.000000000000000000 ) ) ;
#9838=CARTESIAN_POINT ( 'NONE',  ( 232.5999999999999375, -29.99999999999999645, -53.00000000000012079 ) ) ;
#9839=CARTESIAN_POINT ( 'NONE',  ( 232.5999999999999375, -29.99999999999999645, 103.0000000000000000 ) ) ;
#9847=CARTESIAN_POINT ( 'NONE',  ( 231.9680721332268547, -35.00000000000000711, -47.31096265646014842 ) ) ;
#9848=CARTESIAN_POINT ( 'NONE',  ( 235.3564303562499447, -32.69062499938547717, -51.59142580818350865 ) ) ;
#9849=ADVANCED_FACE ( 'NONE', ( #8860 ), #8954, .F. ) ;
#9850=CARTESIAN_POINT ( 'NONE',  ( 233.4038475772933339, -34.31115380933863435, 102.9999999999999858 ) ) ;
#9856=ORIENTED_EDGE ( 'NONE', *, *, #4234, .T. ) ;
#9859=AXIS2_PLACEMENT_3D ( 'NONE', #15889, #13929, #10998 ) ;
#9866=CARTESIAN_POINT ( 'NONE',  ( 235.2033360070650190, -31.99999999999999289, 101.4892189721556690 ) ) ;
#9867=CARTESIAN_POINT ( 'NONE',  ( 229.5999999999999375, -31.83749999999999858, 98.26794919243111792 ) ) ;
#9871=CARTESIAN_POINT ( 'NONE',  ( 231.0999999999999375, -34.06874999877096144, 97.40192378864668399 ) ) ;
#9872=CARTESIAN_POINT ( 'NONE',  ( 235.5999999999999943, -32.00624999877096144, -48.26794919243124582 ) ) ;
#9873=ORIENTED_EDGE ( 'NONE', *, *, #12687, .T. ) ;
#9875=DIRECTION ( 'NONE',  ( -0.000000000000000000, -1.000000000000000000, -0.000000000000000000 ) ) ;
#9882=CARTESIAN_POINT ( 'NONE',  ( 244.7999999999999545, -29.80000000000001492, -97.80000000000002558 ) ) ;
#9886=PRODUCT_DEFINITION_FORMATION_WITH_SPECIFIED_SOURCE ( 'ANY', '', #791, .NOT_KNOWN. ) ;
#9889=CARTESIAN_POINT ( 'NONE',  ( 234.9631320699430432, -35.00000000000000000, -51.64628046580102705 ) ) ;
#9895=ORIENTED_EDGE ( 'NONE', *, *, #458, .F. ) ;
#9897=CARTESIAN_POINT ( 'NONE',  ( 231.0999999999999375, -34.42499999999999716, -47.40192378864679768 ) ) ;
#9898=DIRECTION ( 'NONE',  ( -0.000000000000000000, -1.000000000000000000, -0.000000000000000000 ) ) ;
#9902=CARTESIAN_POINT ( 'NONE',  ( 229.8435696437499871, -31.00312499938547361, -48.40857419181671162 ) ) ;
#9909=AXIS2_PLACEMENT_3D ( 'NONE', #5513, #11459, #14287 ) ;
#9910=LINE ( 'NONE', #18900, #9292 ) ;
#9911=CARTESIAN_POINT ( 'NONE',  ( 229.8435696437499587, -32.80312499938548143, -48.40857419181671162 ) ) ;
#9917=CARTESIAN_POINT ( 'NONE',  ( 233.9782151781249411, -33.44062499938547717, -52.38713871227520968 ) ) ;
#9921=FACE_OUTER_BOUND ( 'NONE', #754, .T. ) ;
#9922=VECTOR ( 'NONE', #6995, 1000.000000000000000 ) ;
#9928=VECTOR ( 'NONE', #1647, 1000.000000000000000 ) ;
#9931=CARTESIAN_POINT ( 'NONE',  ( 232.5999999999999375, -34.83749999999999147, -47.00000000000011369 ) ) ;
#9937=FACE_BOUND ( 'NONE', #8513, .T. ) ;
#9938=CARTESIAN_POINT ( 'NONE',  ( 231.0723800503074870, -32.00000000000002132, 97.66884955414398917 ) ) ;
#9939=DIRECTION ( 'NONE',  ( 0.000000000000000000, -2.001604010742465719E-15, -1.000000000000000000 ) ) ;
#9944=ORIENTED_EDGE ( 'NONE', *, *, #7495, .F. ) ;
#9947=CARTESIAN_POINT ( 'NONE',  ( 234.9210568921013476, -34.99999999999997868, -48.50261820439528293 ) ) ;
#9948=CARTESIAN_POINT ( 'NONE',  ( 229.8435696437499871, -32.54062499938547859, -51.59142580818350865 ) ) ;
#9949=EDGE_CURVE ( 'NONE', #2849, #15232, #6071, .T. ) ;
#9966=DIRECTION ( 'NONE',  ( -0.000000000000000000, -1.000000000000000000, -0.000000000000000000 ) ) ;
#9969=CARTESIAN_POINT ( 'NONE',  ( 232.5999999999999375, -31.68749999999999289, 103.4641016151377499 ) ) ;
#9970=ORIENTED_EDGE ( 'NONE', *, *, #14175, .T. ) ;
#9973=CARTESIAN_POINT ( 'NONE',  ( 231.0999999999999375, -32.11874999877096570, 102.5980762113533018 ) ) ;
#9974=CARTESIAN_POINT ( 'NONE',  ( 234.0999999999999375, -31.14374999877096428, -47.40192378864679768 ) ) ;
#9977=ORIENTED_EDGE ( 'NONE', *, *, #7612, .T. ) ;
#9987=CARTESIAN_POINT ( 'NONE',  ( 246.9999999999999716, -29.80000000000000426, 150.0000000000000000 ) ) ;
#9994=DIRECTION ( 'NONE',  ( 1.000000000000000000, 0.000000000000000000, 0.000000000000000000 ) ) ;
#9995=CARTESIAN_POINT ( 'NONE',  ( 235.3995413886006247, -35.00000000000000000, 99.68825842091030154 ) ) ;
#9999=CARTESIAN_POINT ( 'NONE',  ( 235.3564303562499447, -34.56562499938547717, -48.40857419181671162 ) ) ;
#10006=CARTESIAN_POINT ( 'NONE',  ( 233.9782151781249411, -31.64062499938547646, 97.61286128772489690 ) ) ;
#10012=CARTESIAN_POINT ( 'NONE',  ( 229.8435696437499871, -33.25312499938547717, -48.40857419181671162 ) ) ;
#10018=CARTESIAN_POINT ( 'NONE',  ( 232.5999999999999091, -34.10624999877096286, -53.00000000000010658 ) ) ;
#10036=CARTESIAN_POINT ( 'NONE',  ( 244.7999999999999545, -35.00000000000000000, 147.7999999999999829 ) ) ;
#10038=ORIENTED_EDGE ( 'NONE', *, *, #9949, .T. ) ;
#10041=CARTESIAN_POINT ( 'NONE',  ( 105.1999999999999744, -31.99999999999999289, -100.0000000000000000 ) ) ;
#10042=CARTESIAN_POINT ( 'NONE',  ( 229.8435696437499871, -32.01562499938548001, -48.40857419181671162 ) ) ;
#10044=CARTESIAN_POINT ( 'NONE',  ( 231.7961524227065695, -32.79240381056765585, -53.00000000000011369 ) ) ;
#10045=EDGE_LOOP ( 'NONE', ( #19051, #10902, #15908, #17831 ) ) ;
#10052=CARTESIAN_POINT ( 'NONE',  ( 235.3564303562499447, -30.51562499938548001, 101.5914258081833879 ) ) ;
#10056=VECTOR ( 'NONE', #17476, 1000.000000000000000 ) ;
#10059=CYLINDRICAL_SURFACE ( 'NONE', #4277, 3.000000000000002665 ) ;
#10061=CARTESIAN_POINT ( 'NONE',  ( 235.5999999999999943, -30.26249999999999218, 101.7320508075688537 ) ) ;
#10063=CARTESIAN_POINT ( 'NONE',  ( 229.8435696437499303, -32.05312499938548143, -50.00000000000011369 ) ) ;
#10064=CARTESIAN_POINT ( 'NONE',  ( 235.5999999999999375, -33.31874999877096144, 99.99999999999998579 ) ) ;
#10065=CARTESIAN_POINT ( 'NONE',  ( 232.5999999999999375, -31.40624999877096712, -53.46410161513786363 ) ) ;
#10066=CARTESIAN_POINT ( 'NONE',  ( 232.5999999999999375, -33.48749999999999716, -47.00000000000011369 ) ) ;
#10068=VERTEX_POINT ( 'NONE', #471 ) ;
#10071=VECTOR ( 'NONE', #4503, 1000.000000000000000 ) ;
#10073=CARTESIAN_POINT ( 'NONE',  ( 233.4038475772933054, -34.36740381056765870, -47.00000000000011369 ) ) ;
#10094=CARTESIAN_POINT ( 'NONE',  ( 233.9782151781249411, -32.69062499938547717, -47.61286128772501769 ) ) ;
#10097=EDGE_LOOP ( 'NONE', ( #6535, #401, #18385, #6527, #5288 ) ) ;
#10099=EDGE_CURVE ( 'NONE', #13209, #5719, #15019, .T. ) ;
#10103=CARTESIAN_POINT ( 'NONE',  ( 232.5999999999999375, -32.50312499938547717, 96.81714838363319586 ) ) ;
#10104=CARTESIAN_POINT ( 'NONE',  ( 233.9782151781249411, -32.09062499938547575, -52.38713871227520968 ) ) ;
#10110=CARTESIAN_POINT ( 'NONE',  ( 229.5999999999999375, -31.31249999999998934, -48.26794919243123161 ) ) ;
#10113=ORIENTED_EDGE ( 'NONE', *, *, #17821, .F. ) ;
#10121=CARTESIAN_POINT ( 'NONE',  ( 229.8435696437499587, -33.25312499938547717, 101.5914258081833879 ) ) ;
#10126=CARTESIAN_POINT ( 'NONE',  ( 99.99999999999997158, -29.80000000000000071, 150.0000000000000000 ) ) ;
#10131=CARTESIAN_POINT ( 'NONE',  ( 232.5999999999999375, -34.78124999877096002, -47.00000000000011369 ) ) ;
#10136=CARTESIAN_POINT ( 'NONE',  ( 235.3564303562499447, -35.01562499938548001, 101.5914258081833879 ) ) ;
#10137=CARTESIAN_POINT ( 'NONE',  ( 229.8435696437499871, -34.79062499938547859, -51.59142580818350865 ) ) ;
#10143=ORIENTED_EDGE ( 'NONE', *, *, #15198, .F. ) ;
#10145=( BOUNDED_SURFACE ( )  B_SPLINE_SURFACE ( 1, 2, ( 
 ( #14990, #3159, #16361, #4348, #17927, #1613, #10495, #6106, #15084, #13228, #2877, #10308, #5723, #8834, #16460, #19101, #10399, #7469, #7562, #9120, #2971, #14791, #4536, #155, #12054, #4644, #7181, #19202, #1417, #19303, #11673, #10211, #10594, #11862, #16174, #1519, #17829, #13130, #17637, #2783, #8926, #4441, #8736, #14690, #56, #5817, #11766, #6006, #12535, #13713, #18507, #18124, #10877, #11068, #15475, #1991, #16848, #1794, #7758, #9612, #17038, #18410, #5030, #14001, #9409, #3648, #2087, #7653, #13899, #1701, #18314, #13609, #12348, #4739, #1892, #16940, #5125, #354, #3552, #7947, #6493, #447, #10684, #7850, #15374, #8043, #3452, #16743, #537, #639, #12442, #10970, #251, #12156, #6208, #16652, #9509, #3255, #10780, #6394, #9211, #13805, #6588, #15177, #12251, #6301, #18219, #4837, #3356, #9313, #15277, #4933, #8242, #12737, #15955, #9999, #2372, #5614, #3936, #9708, #17521, #18993, #3741, #8143, #2187, #15669, #1104, #2278, #4041, #11362, #17136, #18606, #6972, #14473, #18895 ),
 ( #14192, #18705, #829, #2559, #17327, #6788, #5221, #12924, #7062, #5515, #11461, #5325, #5422, #926, #11263, #17231, #3835, #17429, #14095, #18797, #15865, #8523, #11559, #9902, #9803, #1021, #13021, #4134, #15574, #734, #15765, #8333, #14289, #6688, #11170, #12632, #6882, #12831, #2472, #8429, #14381, #8618, #7447, #11842, #11746, #6087, #13404, #8814, #1591, #1206, #3046, #7540, #2761, #13498, #7163, #19278, #137, #4514, #10379, #5894, #10185, #16148, #18006, #12034, #36, #5986, #9008, #17810, #10094, #10472, #16052, #2951, #2655, #7349, #14568, #1397, #13112, #10288, #11938, #19083, #8716, #17909, #16341, #14866, #14770, #5701, #16248, #4420, #16437, #8904, #5793, #1493, #14969, #11653, #17614, #4229, #14670, #1305, #7253, #13207, #19179, #17713, #13304, #4328, #2857, #18292, #1683, #15156, #12135, #16828, #6566, #7635, #618, #7925, #3330, #16630, #1773, #5011, #18391, #10758, #13978, #12326, #18105, #12514, #8019, #4716, #16538, #10574, #10661, #9485, #4618, #13589, #3138, #13876, #9290 ) ),
 .UNSPECIFIED., .F., .F., .F. ) 
 B_SPLINE_SURFACE_WITH_KNOTS ( ( 2, 2 ),
 ( 3, 2, 2, 2, 2, 2, 2, 2, 2, 2, 2, 2, 2, 2, 2, 2, 2, 2, 2, 2, 2, 2, 2, 2, 2, 2, 2, 2, 2, 2, 2, 2, 2, 2, 2, 2, 2, 2, 2, 2, 2, 2, 2, 2, 2, 2, 2, 2, 2, 2, 2, 2, 2, 2, 2, 2, 2, 2, 2, 2, 2, 2, 2, 2, 2, 2, 2, 3 ),
 ( 0.000000000000000000, 1.000000000000000000 ),
 ( 0.000000000000000000, 0.01388888888888888812, 0.02777777777777777624, 0.04166666666666666435, 0.05555555555555555247, 0.06944444444444444753, 0.08333333333333332871, 0.09722222222222222376, 0.1111111111111111049, 0.1250000000000000000, 0.1388888888888888951, 0.1527777777777777901, 0.1666666666666666574, 0.1805555555555555525, 0.1944444444444444475, 0.2083333333333333426, 0.2222222222222222099, 0.2361111111111111049, 0.2500000000000000000, 0.2638888888888888951, 0.2777777777777777901, 0.2916666666666666852, 0.3055555555555555802, 0.3194444444444444198, 0.3333333333333333148, 0.3472222222222222099, 0.3611111111111111049, 0.3750000000000000000, 0.3888888888888888951, 0.4027777777777777901, 0.4166666666666666852, 0.4305555555555555802, 0.4444444444444444198, 0.4583333333333333148, 0.4722222222222222099, 0.4861111111111111049, 0.5000000000000000000, 0.5138888888888888395, 0.5277777777777777901, 0.5416666666666666297, 0.5555555555555555802, 0.5694444444444444198, 0.5833333333333333703, 0.5972222222222222099, 0.6111111111111111605, 0.6250000000000000000, 0.6388888888888888395, 0.6527777777777777901, 0.6666666666666666297, 0.6805555555555555802, 0.6944444444444444198, 0.7083333333333333703, 0.7222222222222222099, 0.7361111111111111605, 0.7500000000000000000, 0.7638888888888888395, 0.7777777777777777901, 0.7916666666666666297, 0.8055555555555555802, 0.8194444444444444198, 0.8333333333333333703, 0.8472222222222222099, 0.8611111111111111605, 0.8750000000000000000, 0.8888888888888888395, 0.9027777777777777901, 0.9166666666666666297, 0.9258785565094813652 ),
 .UNSPECIFIED. ) 
 GEOMETRIC_REPRESENTATION_ITEM ( )  RATIONAL_B_SPLINE_SURFACE ( (
 ( 1.000000000000000000, 0.8660254037844387076, 1.000000000000000000, 0.8660254037844387076, 1.000000000000000000, 0.8660254037844387076, 1.000000000000000000, 0.8660254037844387076, 1.000000000000000000, 0.8660254037844387076, 1.000000000000000000, 0.8660254037844387076, 1.000000000000000000, 0.8660254037844387076, 1.000000000000000000, 0.8660254037844387076, 1.000000000000000000, 0.8660254037844387076, 1.000000000000000000, 0.8660254037844387076, 1.000000000000000000, 0.8660254037844387076, 1.000000000000000000, 0.8660254037844387076, 1.000000000000000000, 0.8660254037844387076, 1.000000000000000000, 0.8660254037844387076, 1.000000000000000000, 0.8660254037844387076, 1.000000000000000000, 0.8660254037844387076, 1.000000000000000000, 0.8660254037844387076, 1.000000000000000000, 0.8660254037844387076, 1.000000000000000000, 0.8660254037844387076, 1.000000000000000000, 0.8660254037844387076, 1.000000000000000000, 0.8660254037844387076, 1.000000000000000000, 0.8660254037844387076, 1.000000000000000000, 0.8660254037844387076, 1.000000000000000000, 0.8660254037844387076, 1.000000000000000000, 0.8660254037844387076, 1.000000000000000000, 0.8660254037844387076, 1.000000000000000000, 0.8660254037844387076, 1.000000000000000000, 0.8660254037844387076, 1.000000000000000000, 0.8660254037844387076, 1.000000000000000000, 0.8660254037844387076, 1.000000000000000000, 0.8660254037844387076, 1.000000000000000000, 0.8660254037844387076, 1.000000000000000000, 0.8660254037844387076, 1.000000000000000000, 0.8660254037844387076, 1.000000000000000000, 0.8660254037844387076, 1.000000000000000000, 0.8660254037844387076, 1.000000000000000000, 0.8660254037844387076, 1.000000000000000000, 0.8660254037844387076, 1.000000000000000000, 0.8660254037844387076, 1.000000000000000000, 0.8660254037844387076, 1.000000000000000000, 0.8660254037844387076, 1.000000000000000000, 0.8660254037844387076, 1.000000000000000000, 0.8660254037844387076, 1.000000000000000000, 0.8660254037844387076, 1.000000000000000000, 0.8660254037844387076, 1.000000000000000000, 0.8660254037844387076, 1.000000000000000000, 0.8660254037844387076, 1.000000000000000000, 0.8660254037844387076, 1.000000000000000000, 0.8660254037844387076, 1.000000000000000000, 0.8660254037844387076, 1.000000000000000000, 0.8660254037844387076, 1.000000000000000000, 0.8660254037844387076, 1.000000000000000000, 0.8660254037844387076, 1.000000000000000000, 0.8660254037844387076, 1.000000000000000000, 0.8660254037844387076, 1.000000000000000000, 0.8660254037844387076, 1.000000000000000000, 0.8660254037844387076, 1.000000000000000000, 0.8660254037844387076, 1.000000000000000000, 0.8660254037844387076, 1.000000000000000000, 0.8660254037844387076, 1.000000000000000000, 0.8660254037844387076, 1.000000000000000000, 0.8660254037844387076, 1.000000000000000000, 0.8660254037844387076, 1.000000000000000000, 0.8660254037844387076, 1.000000000000000000, 0.8660254037844387076, 1.000000000000000000, 0.8660254037844387076, 1.000000000000000000, 0.9111405360107203144, 0.9401542295229963209),
 ( 1.000000000000000000, 0.8660254037844387076, 1.000000000000000000, 0.8660254037844387076, 1.000000000000000000, 0.8660254037844387076, 1.000000000000000000, 0.8660254037844387076, 1.000000000000000000, 0.8660254037844387076, 1.000000000000000000, 0.8660254037844387076, 1.000000000000000000, 0.8660254037844387076, 1.000000000000000000, 0.8660254037844387076, 1.000000000000000000, 0.8660254037844387076, 1.000000000000000000, 0.8660254037844387076, 1.000000000000000000, 0.8660254037844387076, 1.000000000000000000, 0.8660254037844387076, 1.000000000000000000, 0.8660254037844387076, 1.000000000000000000, 0.8660254037844387076, 1.000000000000000000, 0.8660254037844387076, 1.000000000000000000, 0.8660254037844387076, 1.000000000000000000, 0.8660254037844387076, 1.000000000000000000, 0.8660254037844387076, 1.000000000000000000, 0.8660254037844387076, 1.000000000000000000, 0.8660254037844387076, 1.000000000000000000, 0.8660254037844387076, 1.000000000000000000, 0.8660254037844387076, 1.000000000000000000, 0.8660254037844387076, 1.000000000000000000, 0.8660254037844387076, 1.000000000000000000, 0.8660254037844387076, 1.000000000000000000, 0.8660254037844387076, 1.000000000000000000, 0.8660254037844387076, 1.000000000000000000, 0.8660254037844387076, 1.000000000000000000, 0.8660254037844387076, 1.000000000000000000, 0.8660254037844387076, 1.000000000000000000, 0.8660254037844387076, 1.000000000000000000, 0.8660254037844387076, 1.000000000000000000, 0.8660254037844387076, 1.000000000000000000, 0.8660254037844387076, 1.000000000000000000, 0.8660254037844387076, 1.000000000000000000, 0.8660254037844387076, 1.000000000000000000, 0.8660254037844387076, 1.000000000000000000, 0.8660254037844387076, 1.000000000000000000, 0.8660254037844387076, 1.000000000000000000, 0.8660254037844387076, 1.000000000000000000, 0.8660254037844387076, 1.000000000000000000, 0.8660254037844387076, 1.000000000000000000, 0.8660254037844387076, 1.000000000000000000, 0.8660254037844387076, 1.000000000000000000, 0.8660254037844387076, 1.000000000000000000, 0.8660254037844387076, 1.000000000000000000, 0.8660254037844387076, 1.000000000000000000, 0.8660254037844387076, 1.000000000000000000, 0.8660254037844387076, 1.000000000000000000, 0.8660254037844387076, 1.000000000000000000, 0.8660254037844387076, 1.000000000000000000, 0.8660254037844387076, 1.000000000000000000, 0.8660254037844387076, 1.000000000000000000, 0.8660254037844387076, 1.000000000000000000, 0.8660254037844387076, 1.000000000000000000, 0.8660254037844387076, 1.000000000000000000, 0.8660254037844387076, 1.000000000000000000, 0.8660254037844387076, 1.000000000000000000, 0.8660254037844387076, 1.000000000000000000, 0.8660254037844387076, 1.000000000000000000, 0.8660254037844387076, 1.000000000000000000, 0.8660254037844387076, 1.000000000000000000, 0.8660254037844387076, 1.000000000000000000, 0.8660254037844387076, 1.000000000000000000, 0.8660254037844387076, 1.000000000000000000, 0.8660254037844387076, 1.000000000000000000, 0.9111405360107203144, 0.9401542295229963209) ) ) 
 REPRESENTATION_ITEM ( '' )  SURFACE ( )  );
#10147=CARTESIAN_POINT ( 'NONE',  ( 233.9782151781249411, -30.55312499938548143, 102.3871387122750889 ) ) ;
#10151=DIRECTION ( 'NONE',  ( 1.000000000000000000, 0.000000000000000000, -0.000000000000000000 ) ) ;
#10152=CIRCLE ( 'NONE', #15772, 5.199999999999996625 ) ;
#10155=CARTESIAN_POINT ( 'NONE',  ( 234.0999999999999375, -32.09999999999999432, 102.5980762113533018 ) ) ;
#10158=CARTESIAN_POINT ( 'NONE',  ( 235.5999999999999943, -32.38124999877096144, 98.26794919243110371 ) ) ;
#10159=CARTESIAN_POINT ( 'NONE',  ( 234.0999999999999375, -33.39374999877096428, -47.40192378864679768 ) ) ;
#10166=ORIENTED_EDGE ( 'NONE', *, *, #13150, .F. ) ;
#10172=CARTESIAN_POINT ( 'NONE',  ( 235.5999999999999375, -32.41874999877096286, -50.00000000000011369 ) ) ;
#10176=CARTESIAN_POINT ( 'NONE',  ( 231.2217848218749339, -30.51562499938548001, 102.3871387122750889 ) ) ;
#10182=CARTESIAN_POINT ( 'NONE',  ( 231.2217848218749339, -34.82812499938548001, 97.61286128772489690 ) ) ;
#10185=CARTESIAN_POINT ( 'NONE',  ( 229.8435696437499303, -32.39062499938548001, -50.00000000000011369 ) ) ;
#10187=EDGE_CURVE ( 'NONE', #11798, #9344, #13923, .T. ) ;
#10195=CARTESIAN_POINT ( 'NONE',  ( 229.8435696437499871, -31.52812499938547575, 98.40857419181659793 ) ) ;
#10196=CARTESIAN_POINT ( 'NONE',  ( 232.5999999999999943, -34.30312499938547433, -53.18285161636690361 ) ) ;
#10198=CARTESIAN_POINT ( 'NONE',  ( 105.1999999999999602, -32.00000000000000711, -97.80000000000002558 ) ) ;
#10199=FACE_OUTER_BOUND ( 'NONE', #16877, .T. ) ;
#10202=CARTESIAN_POINT ( 'NONE',  ( 232.5999999999999375, -34.97812499938547859, -46.81714838363331666 ) ) ;
#10206=VECTOR ( 'NONE', #7720, 1000.000000000000000 ) ;
#10211=CARTESIAN_POINT ( 'NONE',  ( 235.3564303562499447, -31.41562499938548214, -48.40857419181671162 ) ) ;
#10215=CARTESIAN_POINT ( 'NONE',  ( 235.3564303562499447, -33.02812499938547575, 98.40857419181659793 ) ) ;
#10216=FACE_OUTER_BOUND ( 'NONE', #16028, .T. ) ;
#10218=AXIS2_PLACEMENT_3D ( 'NONE', #7891, #1927, #5159 ) ;
#10225=VECTOR ( 'NONE', #9898, 1000.000000000000000 ) ;
#10233=CARTESIAN_POINT ( 'NONE',  ( 229.8435696437499871, -33.81562499938547717, 101.5914258081833879 ) ) ;
#10235=DIRECTION ( 'NONE',  ( -0.000000000000000000, -1.000000000000000000, -0.000000000000000000 ) ) ;
#10239=VERTEX_POINT ( 'NONE', #6909 ) ;
#10243=CARTESIAN_POINT ( 'NONE',  ( 231.7961524227065695, -33.69240381056765443, -53.00000000000010658 ) ) ;
#10249=CARTESIAN_POINT ( 'NONE',  ( 229.8435696437499871, -31.11562499938547788, 101.5914258081833879 ) ) ;
#10257=CARTESIAN_POINT ( 'NONE',  ( 229.5999999999999375, -34.01249999999999574, 101.7320508075688679 ) ) ;
#10258=VERTEX_POINT ( 'NONE', #9931 ) ;
#10260=CARTESIAN_POINT ( 'NONE',  ( 231.0999999999999375, -32.56874999877096144, 102.5980762113533018 ) ) ;
#10261=CARTESIAN_POINT ( 'NONE',  ( 231.0999999999999375, -34.36874999877096570, -47.40192378864679768 ) ) ;
#10264=ORIENTED_EDGE ( 'NONE', *, *, #11037, .F. ) ;
#10267=( BOUNDED_CURVE ( )  B_SPLINE_CURVE ( 2, ( #17024, #9792, #11055, #15360, #627, #2263, #3822, #524, #8232 ),
 .UNSPECIFIED., .F., .F. ) 
 B_SPLINE_CURVE_WITH_KNOTS ( ( 3, 2, 2, 2, 3 ),
 ( 0.5625000000000002220, 0.5694444444444444198, 0.5833333333333333703, 0.5972222222222222099, 0.6041666666666667407 ),
 .UNSPECIFIED. ) 
 CURVE ( )  GEOMETRIC_REPRESENTATION_ITEM ( )  RATIONAL_B_SPLINE_CURVE ( ( 0.9330127018922194093, 0.9330127018922215187, 1.000000000000000000, 0.8660254037844387076, 1.000000000000000000, 0.8660254037844387076, 1.000000000000000000, 0.9330127018922187432, 0.9330127018922192983 ) ) 
 REPRESENTATION_ITEM ( '' )  );
#10268=CARTESIAN_POINT ( 'NONE',  ( 229.5999999999999375, -34.94999999999999574, 99.99999999999998579 ) ) ;
#10269=PLANE ( 'NONE',  #7859 ) ;
#10270=ORIENTED_EDGE ( 'NONE', *, *, #412, .F. ) ;
#10271=CARTESIAN_POINT ( 'NONE',  ( 232.5999999999999375, -34.61249999999999716, -53.00000000000011369 ) ) ;
#10276=CARTESIAN_POINT ( 'NONE',  ( 231.0723800503075154, -31.99999999999999289, -52.33115044585625242 ) ) ;
#10279=CARTESIAN_POINT ( 'NONE',  ( 244.7999999999999545, -29.80000000000000426, 150.0000000000000000 ) ) ;
#10280=ORIENTED_EDGE ( 'NONE', *, *, #9358, .T. ) ;
#10285=CARTESIAN_POINT ( 'NONE',  ( 229.5999999999999375, -34.40624999877096002, 101.7320508075688821 ) ) ;
#10288=CARTESIAN_POINT ( 'NONE',  ( 235.3564303562499447, -33.02812499938547575, -51.59142580818350865 ) ) ;
#10290=EDGE_LOOP ( 'NONE', ( #2711, #9441, #12970, #2611 ) ) ;
#10296=CARTESIAN_POINT ( 'NONE',  ( 232.5999999999999375, -32.27812499938547575, 103.1828516163667899 ) ) ;
#10297=CARTESIAN_POINT ( 'NONE',  ( 231.2217848218749339, -33.21562499938547575, -47.61286128772501769 ) ) ;
#10298=CARTESIAN_POINT ( 'NONE',  ( 232.5999999999999375, -29.99999999999999645, 99.99999999999998579 ) ) ;
#10300=EDGE_CURVE ( 'NONE', #484, #6637, #15451, .T. ) ;
#10303=CARTESIAN_POINT ( 'NONE',  ( 233.9782151781249411, -34.94062499938547717, -47.61286128772501769 ) ) ;
#10308=CARTESIAN_POINT ( 'NONE',  ( 229.8435696437499871, -30.66562499938547859, -48.40857419181671162 ) ) ;
#10310=ORIENTED_EDGE ( 'NONE', *, *, #17948, .F. ) ;
#10313=EDGE_CURVE ( 'NONE', #13743, #15900, #5249, .T. ) ;
#10314=CARTESIAN_POINT ( 'NONE',  ( 230.9489134087918671, -32.00820041275123629, 97.77040367152254419 ) ) ;
#10317=DIRECTION ( 'NONE',  ( -1.000000000000000000, -0.000000000000000000, -0.000000000000000000 ) ) ;
#10328=DIRECTION ( 'NONE',  ( 0.000000000000000000, -3.491481338843133355E-15, -1.000000000000000000 ) ) ;
#10330=CARTESIAN_POINT ( 'NONE',  ( 232.5999999999999659, -32.81249999999999289, 97.00000000000000000 ) ) ;
#10338=CARTESIAN_POINT ( 'NONE',  ( 233.9782151781249411, -32.80312499938548143, 102.3871387122750889 ) ) ;
#10345=CARTESIAN_POINT ( 'NONE',  ( 235.5999999999999943, -33.78749999999999432, 98.26794919243110371 ) ) ;
#10349=CARTESIAN_POINT ( 'NONE',  ( 231.0999999999999375, -35.26874999877096428, 102.5980762113533018 ) ) ;
#10350=CARTESIAN_POINT ( 'NONE',  ( 231.0999999999999375, -33.91874999877096286, -47.40192378864679768 ) ) ;
#10353=ORIENTED_EDGE ( 'NONE', *, *, #12952, .F. ) ;
#10355=CARTESIAN_POINT ( 'NONE',  ( 105.1999999999999744, -34.99999999999999289, 150.0000000000000000 ) ) ;
#10356=CARTESIAN_POINT ( 'NONE',  ( 232.5999999999999375, -29.99999999999999645, 99.99999999999998579 ) ) ;
#10360=VECTOR ( 'NONE', #6711, 1000.000000000000000 ) ;
#10368=CARTESIAN_POINT ( 'NONE',  ( 233.9782151781249411, -30.74062499938547788, 97.61286128772489690 ) ) ;
#10376=CARTESIAN_POINT ( 'NONE',  ( 232.5999999999999375, -34.78124999877096002, -47.00000000000011369 ) ) ;
#10378=DIRECTION ( 'NONE',  ( 0.000000000000000000, 0.000000000000000000, 1.000000000000000000 ) ) ;
#10379=CARTESIAN_POINT ( 'NONE',  ( 231.2217848218749339, -32.31562499938547717, -47.61286128772501769 ) ) ;
#10381=EDGE_LOOP ( 'NONE', ( #3281, #12253, #8885, #3407 ) ) ;
#10388=CARTESIAN_POINT ( 'NONE',  ( 231.2217848218749339, -34.11562499938548143, 102.3871387122750889 ) ) ;
#10389=CARTESIAN_POINT ( 'NONE',  ( 235.3564303562499447, -34.82812499938548001, -51.59142580818350154 ) ) ;
#10393=CARTESIAN_POINT ( 'NONE',  ( 229.8435696437499303, -34.64062499938548001, -50.00000000000011369 ) ) ;
#10396=ORIENTED_EDGE ( 'NONE', *, *, #3306, .T. ) ;
#10399=CARTESIAN_POINT ( 'NONE',  ( 233.9782151781249411, -30.85312499938547859, -52.38713871227520968 ) ) ;
#10403=CARTESIAN_POINT ( 'NONE',  ( 231.2217848218749339, -34.56562499938547717, 102.3871387122750889 ) ) ;
#10411=LINE ( 'NONE', #7667, #9276 ) ;
#10417=DIRECTION ( 'NONE',  ( 1.000000000000000000, 0.000000000000000000, 0.000000000000000000 ) ) ;
#10421=DIRECTION ( 'NONE',  ( 0.000000000000000000, 0.000000000000000000, 1.000000000000000000 ) ) ;
#10425=EDGE_CURVE ( 'NONE', #13758, #12372, #4067, .T. ) ;
#10427=DIRECTION ( 'NONE',  ( 0.000000000000000000, 0.000000000000000000, -1.000000000000000000 ) ) ;
#10429=CARTESIAN_POINT ( 'NONE',  ( 235.3564303562499447, -30.96562499938547930, 101.5914258081833879 ) ) ;
#10437=CARTESIAN_POINT ( 'NONE',  ( 229.5999999999999375, -34.08749999999999147, 98.26794919243111792 ) ) ;
#10440=CARTESIAN_POINT ( 'NONE',  ( 232.5999999999999943, -33.74062499938548143, -46.81714838363331666 ) ) ;
#10442=CARTESIAN_POINT ( 'NONE',  ( 232.5999999999999375, -34.33124999877096428, 103.4641016151377499 ) ) ;
#10443=CARTESIAN_POINT ( 'NONE',  ( 232.5999999999999375, -34.10624999877096286, -53.46410161513786363 ) ) ;
#10444=ADVANCED_FACE ( 'NONE', ( #10216 ), #11678, .F. ) ;
#10448=DIRECTION ( 'NONE',  ( 1.000000000000000000, 0.000000000000000000, -0.000000000000000000 ) ) ;
#10462=DIRECTION ( 'NONE',  ( -1.000000000000000000, 0.000000000000000000, 0.000000000000000000 ) ) ;
#10472=CARTESIAN_POINT ( 'NONE',  ( 232.5999999999999375, -32.72812499938547859, -46.81714838363331666 ) ) ;
#10482=CARTESIAN_POINT ( 'NONE',  ( 235.3564303562499447, -34.37812499938547717, 98.40857419181659793 ) ) ;
#10483=AXIS2_PLACEMENT_3D ( 'NONE', #4672, #13456, #10427 ) ;
#10484=CARTESIAN_POINT ( 'NONE',  ( 232.5999999999999943, -33.17812499938548143, -46.81714838363331666 ) ) ;
#10488=ORIENTED_EDGE ( 'NONE', *, *, #1235, .T. ) ;
#10489=CARTESIAN_POINT ( 'NONE',  ( 229.5999999999999375, -29.99999999999999645, -50.00000000000011369 ) ) ;
#10495=CARTESIAN_POINT ( 'NONE',  ( 235.3564303562499447, -30.47812499938547859, -50.00000000000011369 ) ) ;
#10496=VECTOR ( 'NONE', #11892, 1000.000000000000000 ) ;
#10504=CARTESIAN_POINT ( 'NONE',  ( 249.9999999999999716, -29.80000000000000426, -100.0000000000000000 ) ) ;
#10506=CARTESIAN_POINT ( 'NONE',  ( 230.9316747517339081, -35.00000000000000000, 102.2567273996571515 ) ) ;
#10512=ORIENTED_EDGE ( 'NONE', *, *, #10425, .T. ) ;
#10516=CARTESIAN_POINT ( 'NONE',  ( 232.5999999999999375, -34.64062499938548001, -46.81714838363331666 ) ) ;
#10526=CARTESIAN_POINT ( 'NONE',  ( 229.5999999999999375, -34.49999999999999289, -50.00000000000011369 ) ) ;
#10527=CARTESIAN_POINT ( 'NONE',  ( 235.3564303562499447, -31.34062499938548285, 98.40857419181659793 ) ) ;
#10537=AXIS2_PLACEMENT_3D ( 'NONE', #2821, #6050, #8777 ) ;
#10538=CARTESIAN_POINT ( 'NONE',  ( 235.5999999999999375, -34.72499999999999432, 99.99999999999998579 ) ) ;
#10540=AXIS2_PLACEMENT_3D ( 'NONE', #7341, #19270, #11738 ) ;
#10543=CARTESIAN_POINT ( 'NONE',  ( 232.5999999999999943, -33.51562499938548001, -53.18285161636690361 ) ) ;
#10545=CARTESIAN_POINT ( 'NONE',  ( 229.8435696437499871, -31.11562499938547788, 101.5914258081833879 ) ) ;
#10546=CARTESIAN_POINT ( 'NONE',  ( 235.5999999999999943, -32.45624999877096428, -48.26794919243124582 ) ) ;
#10548=ORIENTED_EDGE ( 'NONE', *, *, #4234, .F. ) ;
#10555=CARTESIAN_POINT ( 'NONE',  ( 232.5999999999999659, -32.58749999999999858, 102.9999999999999858 ) ) ;
#10557=EDGE_CURVE ( 'NONE', #4900, #1498, #12950, .T. ) ;
#10561=LINE ( 'NONE', #1763, #3799 ) ;
#10565=CARTESIAN_POINT ( 'NONE',  ( 232.5999999999999375, -31.37812499938547717, 103.1828516163667899 ) ) ;
#10570=CARTESIAN_POINT ( 'NONE',  ( 235.5999999999999943, -33.78750000000000142, 98.26794919243110371 ) ) ;
#10574=CARTESIAN_POINT ( 'NONE',  ( 235.3564303562499447, -34.90312499938547575, -48.40857419181671162 ) ) ;
#10583=CARTESIAN_POINT ( 'NONE',  ( 232.5999999999999375, -33.17812499938548143, 103.1828516163667899 ) ) ;
#10584=CARTESIAN_POINT ( 'NONE',  ( 235.3564303562499447, -33.55312499938548143, -48.40857419181671162 ) ) ;
#10585=DIRECTION ( 'NONE',  ( 0.000000000000000000, 0.000000000000000000, 1.000000000000000000 ) ) ;
#10588=CARTESIAN_POINT ( 'NONE',  ( 229.5999999999999375, -31.76249999999999218, -48.26794919243123161 ) ) ;
#10594=CARTESIAN_POINT ( 'NONE',  ( 233.9782151781249411, -31.45312499938548356, -47.61286128772501769 ) ) ;
#10598=CARTESIAN_POINT ( 'NONE',  ( 235.3564303562499447, -34.45312499938548001, 101.5914258081833879 ) ) ;
#10622=CARTESIAN_POINT ( 'NONE',  ( 229.8435696437499871, -32.09062499938548285, 98.40857419181659793 ) ) ;
#10628=DIRECTION ( 'NONE',  ( -1.000000000000000000, 0.000000000000000000, -0.000000000000000000 ) ) ;
#10631=CARTESIAN_POINT ( 'NONE',  ( 232.5999999999999375, -34.16249999999999432, 96.53589838486223584 ) ) ;
#10632=ORIENTED_EDGE ( 'NONE', *, *, #11295, .F. ) ;
#10633=CARTESIAN_POINT ( 'NONE',  ( 231.2217848218749339, -33.32812499938548001, -47.61286128772501769 ) ) ;
#10635=CARTESIAN_POINT ( 'NONE',  ( 235.5999999999999943, -35.15624999877096002, 101.7320508075688537 ) ) ;
#10636=CARTESIAN_POINT ( 'NONE',  ( 234.0999999999999375, -34.74374999877096570, -47.40192378864679768 ) ) ;
#10638=ORIENTED_EDGE ( 'NONE', *, *, #17371, .T. ) ;
#10644=LINE ( 'NONE', #7619, #14856 ) ;
#10647=( BOUNDED_CURVE ( )  B_SPLINE_CURVE ( 2, ( #14542, #17203, #1079, #2249, #8220, #7037, #18964, #801, #12703 ),
 .UNSPECIFIED., .F., .F. ) 
 B_SPLINE_CURVE_WITH_KNOTS ( ( 3, 2, 2, 2, 3 ),
 ( 0.8125000000000000000, 0.8194444444444444198, 0.8333333333333333703, 0.8472222222222222099, 0.8541666666666668517 ),
 .UNSPECIFIED. ) 
 CURVE ( )  GEOMETRIC_REPRESENTATION_ITEM ( )  RATIONAL_B_SPLINE_CURVE ( ( 0.9330127018922194093, 0.9330127018922194093, 1.000000000000000000, 0.8660254037844387076, 1.000000000000000000, 0.8660254037844387076, 1.000000000000000000, 0.9330127018922177440, 0.9330127018922194093 ) ) 
 REPRESENTATION_ITEM ( '' )  );
#10651=CARTESIAN_POINT ( 'NONE',  ( 235.5999999999999943, -33.41249999999999432, 101.7320508075688537 ) ) ;
#10654=CARTESIAN_POINT ( 'NONE',  ( 233.9782151781249411, -32.24062499938548143, 102.3871387122750889 ) ) ;
#10660=CARTESIAN_POINT ( 'NONE',  ( 229.8966310988219846, -35.00000000000002132, -49.00607337841733369 ) ) ;
#10661=CARTESIAN_POINT ( 'NONE',  ( 233.9782151781249411, -34.94062499938547717, -47.61286128772501769 ) ) ;
#10663=VERTEX_POINT ( 'NONE', #13615 ) ;
#10670=CARTESIAN_POINT ( 'NONE',  ( 233.9782151781249411, -33.44062499938547717, 97.61286128772489690 ) ) ;
#10676=ORIENTED_EDGE ( 'NONE', *, *, #19299, .F. ) ;
#10677=CARTESIAN_POINT ( 'NONE',  ( 234.0999999999999375, -33.44999999999999574, -47.40192378864679768 ) ) ;
#10684=CARTESIAN_POINT ( 'NONE',  ( 231.2217848218749339, -33.32812499938548001, -47.61286128772501769 ) ) ;
#10687=VERTEX_POINT ( 'NONE', #2235 ) ;
#10690=CARTESIAN_POINT ( 'NONE',  ( 229.8435696437499587, -33.70312499938548001, 101.5914258081833879 ) ) ;
#10699=CARTESIAN_POINT ( 'NONE',  ( 233.9782151781249411, -31.79062499938548214, -47.61286128772501769 ) ) ;
#10716=DIRECTION ( 'NONE',  ( -1.000000000000000000, -0.000000000000000000, -0.000000000000000000 ) ) ;
#10717=CARTESIAN_POINT ( 'NONE',  ( 229.8435696437499871, -34.34062499938547575, 98.40857419181659793 ) ) ;
#10723=CARTESIAN_POINT ( 'NONE',  ( 105.1999999999999744, -4.999999999999976907, 153.0000000000000000 ) ) ;
#10728=CARTESIAN_POINT ( 'NONE',  ( 229.8435696437499587, -34.26562499938548001, -48.40857419181671162 ) ) ;
#10730=CARTESIAN_POINT ( 'NONE',  ( 232.5999999999999375, -35.23124999877096286, 103.4641016151377499 ) ) ;
#10731=CARTESIAN_POINT ( 'NONE',  ( 235.3564303562499447, -30.89062499938548001, -51.59142580818350865 ) ) ;
#10732=CARTESIAN_POINT ( 'NONE',  ( 232.5999999999999375, -34.61249999999999716, -53.00000000000011369 ) ) ;
#10739=CARTESIAN_POINT ( 'NONE',  ( 99.99999999999997158, -5.200000000000008171, 150.0000000000000000 ) ) ;
#10740=CARTESIAN_POINT ( 'NONE',  ( 231.7961524227065411, -34.08615380933862582, 97.00000000000000000 ) ) ;
#10750=CARTESIAN_POINT ( 'NONE',  ( 235.3564303562499447, -32.57812499938547290, 98.40857419181659793 ) ) ;
#10754=VERTEX_POINT ( 'NONE', #7974 ) ;
#10756=CARTESIAN_POINT ( 'NONE',  ( 246.9999999999999716, -5.000000000000004441, -100.0000000000000000 ) ) ;
#10757=LINE ( 'NONE', #16436, #390 ) ;
#10758=CARTESIAN_POINT ( 'NONE',  ( 229.8435696437499871, -34.60312499938547859, -48.40857419181671162 ) ) ;
#10766=CARTESIAN_POINT ( 'NONE',  ( 229.8435696437499303, -34.19062499938547717, 99.99999999999998579 ) ) ;
#10767=( BOUNDED_CURVE ( )  B_SPLINE_CURVE ( 2, ( #8567, #17567, #15717, #5369, #12781, #8193, #12678, #10044, #14333 ),
 .UNSPECIFIED., .F., .F. ) 
 B_SPLINE_CURVE_WITH_KNOTS ( ( 3, 2, 2, 2, 3 ),
 ( 0.4791666666666665186, 0.4861111111111111049, 0.5000000000000000000, 0.5138888888888888395, 0.5208333333333332593 ),
 .UNSPECIFIED. ) 
 CURVE ( )  GEOMETRIC_REPRESENTATION_ITEM ( )  RATIONAL_B_SPLINE_CURVE ( ( 0.9330127018922194093, 0.9330127018922180770, 1.000000000000000000, 0.8660254037844387076, 1.000000000000000000, 0.8660254037844387076, 1.000000000000000000, 0.9330127018922198534, 0.9330127018922192983 ) ) 
 REPRESENTATION_ITEM ( '' )  );
#10774=CARTESIAN_POINT ( 'NONE',  ( 234.0999999999999375, -32.84999999999999432, -52.59807621135342970 ) ) ;
#10778=DIRECTION ( 'NONE',  ( -0.000000000000000000, -1.000000000000000000, -0.000000000000000000 ) ) ;
#10780=CARTESIAN_POINT ( 'NONE',  ( 231.2217848218749339, -33.92812499938548143, -52.38713871227520968 ) ) ;
#10785=CARTESIAN_POINT ( 'NONE',  ( 229.8435696437499587, -34.67812499938547433, 98.40857419181659793 ) ) ;
#10787=ADVANCED_FACE ( 'NONE', ( #18343 ), #14121, .F. ) ;
#10794=CARTESIAN_POINT ( 'NONE',  ( 244.7999999999999545, -35.00000000000000000, 150.0000000000000000 ) ) ;
#10802=FACE_OUTER_BOUND ( 'NONE', #6946, .T. ) ;
#10803=ORIENTED_EDGE ( 'NONE', *, *, #6180, .F. ) ;
#10810=CARTESIAN_POINT ( 'NONE',  ( 231.2217848218749339, -35.12812499938548427, 102.3871387122750889 ) ) ;
#10813=LINE ( 'NONE', #1921, #12733 ) ;
#10819=EDGE_LOOP ( 'NONE', ( #2858, #15009, #7009, #951 ) ) ;
#10820=CARTESIAN_POINT ( 'NONE',  ( 235.3564303562499447, -33.66562499938548569, -48.40857419181671162 ) ) ;
#10822=CARTESIAN_POINT ( 'NONE',  ( 233.9782151781249411, -31.90312499938548285, 102.3871387122750889 ) ) ;
#10823=CARTESIAN_POINT ( 'NONE',  ( 231.2217848218749339, -31.52812499938548285, -47.61286128772501769 ) ) ;
#10825=( BOUNDED_CURVE ( )  B_SPLINE_CURVE ( 2, ( #1917, #473, #6797, #6422, #12743, #18711, #13027, #17334, #4335 ),
 .UNSPECIFIED., .F., .F. ) 
 B_SPLINE_CURVE_WITH_KNOTS ( ( 3, 2, 2, 2, 3 ),
 ( 0.4791666666666666852, 0.4861111111111111049, 0.5000000000000000000, 0.5138888888888888395, 0.5208333333333331483 ),
 .UNSPECIFIED. ) 
 CURVE ( )  GEOMETRIC_REPRESENTATION_ITEM ( )  RATIONAL_B_SPLINE_CURVE ( ( 0.9330127018922194093, 0.9330127018922196314, 1.000000000000000000, 0.8660254037844387076, 1.000000000000000000, 0.8660254037844387076, 1.000000000000000000, 0.9330127018922209636, 0.9330127018922194093 ) ) 
 REPRESENTATION_ITEM ( '' )  );
#10827=ORIENTED_EDGE ( 'NONE', *, *, #9949, .F. ) ;
#10829=ORIENTED_EDGE ( 'NONE', *, *, #9337, .F. ) ;
#10841=CARTESIAN_POINT ( 'NONE',  ( 244.7999999999999545, -35.00000000000000000, 150.0000000000000000 ) ) ;
#10843=CARTESIAN_POINT ( 'NONE',  ( 231.2217848218749339, -33.36562499938548143, 97.61286128772489690 ) ) ;
#10844=CARTESIAN_POINT ( 'NONE',  ( 231.2217848218749339, -32.76562499938548001, 102.3871387122750889 ) ) ;
#10845=ORIENTED_EDGE ( 'NONE', *, *, #19313, .F. ) ;
#10847=CIRCLE ( 'NONE', #12090, 2.199999999999993516 ) ;
#10848=CARTESIAN_POINT ( 'NONE',  ( 229.5999999999999375, -31.29374999877096286, 99.99999999999998579 ) ) ;
#10849=FACE_BOUND ( 'NONE', #5918, .T. ) ;
#10856=VECTOR ( 'NONE', #2581, 1000.000000000000000 ) ;
#10862=DIRECTION ( 'NONE',  ( 1.000000000000000000, -4.625929269271214620E-17, 4.415659757031858318E-14 ) ) ;
#10864=LINE ( 'NONE', #18591, #3689 ) ;
#10872=CARTESIAN_POINT ( 'NONE',  ( 232.5999999999999375, -32.81249999999999289, -53.46410161513786363 ) ) ;
#10875=CARTESIAN_POINT ( 'NONE',  ( 232.5999999999999375, -29.99999999999999645, -50.00000000000011369 ) ) ;
#10877=CARTESIAN_POINT ( 'NONE',  ( 233.9782151781249411, -32.20312499938548001, -52.38713871227520968 ) ) ;
#10891=CARTESIAN_POINT ( 'NONE',  ( 229.8435696437499871, -30.62812499938547717, -51.59142580818350865 ) ) ;
#10894=EDGE_LOOP ( 'NONE', ( #4741, #7138, #12325, #117 ) ) ;
#10896=CARTESIAN_POINT ( 'NONE',  ( 231.0999999999999375, -32.17499999999999716, 102.5980762113533018 ) ) ;
#10902=ORIENTED_EDGE ( 'NONE', *, *, #1230, .F. ) ;
#10907=DIRECTION ( 'NONE',  ( -0.000000000000000000, 0.000000000000000000, 1.000000000000000000 ) ) ;
#10909=CARTESIAN_POINT ( 'NONE',  ( 233.9782151781249411, -33.70312499938548001, 102.3871387122750889 ) ) ;
#10912=DIRECTION ( 'NONE',  ( 1.000000000000000000, 0.000000000000000000, 0.000000000000000000 ) ) ;
#10922=CARTESIAN_POINT ( 'NONE',  ( 229.8435696437499871, -32.99062499938548143, 98.40857419181659793 ) ) ;
#10923=CARTESIAN_POINT ( 'NONE',  ( 232.5999999999999375, -31.26562499938548356, -53.18285161636690361 ) ) ;
#10930=EDGE_CURVE ( 'NONE', #9169, #12702, #8293, .T. ) ;
#10931=CARTESIAN_POINT ( 'NONE',  ( 232.5999999999999375, -29.99999999999999645, -53.00000000000012079 ) ) ;
#10939=CARTESIAN_POINT ( 'NONE',  ( 244.7999999999999545, -29.80000000000002203, 147.7999999999999829 ) ) ;
#10941=CARTESIAN_POINT ( 'NONE',  ( 235.3564303562499447, -33.51562499938548001, 99.99999999999998579 ) ) ;
#10943=CARTESIAN_POINT ( 'NONE',  ( 231.0999999999999375, -31.21874999877096357, 102.5980762113533018 ) ) ;
#10944=DIRECTION ( 'NONE',  ( 1.000000000000000000, -4.625929269271485174E-17, 0.000000000000000000 ) ) ;
#10945=ORIENTED_EDGE ( 'NONE', *, *, #4451, .F. ) ;
#10950=ORIENTED_EDGE ( 'NONE', *, *, #101, .T. ) ;
#10966=CARTESIAN_POINT ( 'NONE',  ( 231.0999999999999375, -31.72499999999999787, -47.40192378864679768 ) ) ;
#10970=CARTESIAN_POINT ( 'NONE',  ( 235.3564303562499447, -33.66562499938548569, -48.40857419181671162 ) ) ;
#10977=VECTOR ( 'NONE', #309, 1000.000000000000000 ) ;
#10978=CARTESIAN_POINT ( 'NONE',  ( 233.4038475772933339, -34.63259618943233420, 97.00000000000000000 ) ) ;
#10983=CARTESIAN_POINT ( 'NONE',  ( 233.9782151781249411, -30.89062499938548001, -47.61286128772501769 ) ) ;
#10991=( BOUNDED_CURVE ( )  B_SPLINE_CURVE ( 2, ( #4657, #16192, #17844, #2984, #1242, #2800, #7194, #4363, #16282 ),
 .UNSPECIFIED., .F., .F. ) 
 B_SPLINE_CURVE_WITH_KNOTS ( ( 3, 2, 2, 2, 3 ),
 ( 0.8125000000000000000, 0.8194444444444444198, 0.8333333333333333703, 0.8472222222222222099, 0.8530683953269213582 ),
 .UNSPECIFIED. ) 
 CURVE ( )  GEOMETRIC_REPRESENTATION_ITEM ( )  RATIONAL_B_SPLINE_CURVE ( ( 0.9330127018922194093, 0.9330127018922194093, 1.000000000000000000, 0.8660254037844387076, 1.000000000000000000, 0.8660254037844387076, 1.000000000000000000, 0.9436068149601996025, 0.9346881722405915305 ) ) 
 REPRESENTATION_ITEM ( '' )  );
#10996=VERTEX_POINT ( 'NONE', #17647 ) ;
#10998=DIRECTION ( 'NONE',  ( 0.000000000000000000, 0.000000000000000000, 1.000000000000000000 ) ) ;
#11000=CARTESIAN_POINT ( 'NONE',  ( 232.5999999999999375, -34.19062499938547717, 103.1828516163667899 ) ) ;
#11006=VECTOR ( 'NONE', #2019, 1000.000000000000000 ) ;
#11012=CARTESIAN_POINT ( 'NONE',  ( 235.3564303562499447, -34.56562499938547717, -48.40857419181671162 ) ) ;
#11014=CARTESIAN_POINT ( 'NONE',  ( 235.3564303562499447, -31.34062499938548285, 98.40857419181659793 ) ) ;
#11015=CARTESIAN_POINT ( 'NONE',  ( 233.9782151781249411, -31.75312499938547717, -52.38713871227520968 ) ) ;
#11018=CARTESIAN_POINT ( 'NONE',  ( 234.0999999999999375, -34.64999999999999147, -52.59807621135342970 ) ) ;
#11019=ORIENTED_EDGE ( 'NONE', *, *, #9014, .F. ) ;
#11024=DIRECTION ( 'NONE',  ( -1.000000000000000000, 0.000000000000000000, -0.000000000000000000 ) ) ;
#11035=DIRECTION ( 'NONE',  ( -0.000000000000000000, 0.000000000000000000, -1.000000000000000000 ) ) ;
#11036=CARTESIAN_POINT ( 'NONE',  ( 235.3564303562499447, -34.86562499938547433, 99.99999999999998579 ) ) ;
#11037=EDGE_CURVE ( 'NONE', #3413, #4556, #16092, .T. ) ;
#11040=CARTESIAN_POINT ( 'NONE',  ( 229.5999999999999375, -30.80624999877096215, 101.7320508075688679 ) ) ;
#11047=CARTESIAN_POINT ( 'NONE',  ( 99.99999999999997158, -5.200000000000008171, -100.0000000000000000 ) ) ;
#11048=CARTESIAN_POINT ( 'NONE',  ( 232.5999999999999375, -33.88124999877096855, -47.00000000000011369 ) ) ;
#11050=CARTESIAN_POINT ( 'NONE',  ( 232.5999999999999375, -33.48749999999999716, -47.00000000000011369 ) ) ;
#11055=CARTESIAN_POINT ( 'NONE',  ( 231.0999999999999375, -33.07499999999999574, 102.5980762113533018 ) ) ;
#11061=CARTESIAN_POINT ( 'NONE',  ( 229.5999999999999375, -34.91249999999999432, -48.26794919243123161 ) ) ;
#11062=ADVANCED_FACE ( 'NONE', ( #13338 ), #5924, .T. ) ;
#11066=CARTESIAN_POINT ( 'NONE',  ( 229.8435696437499303, -32.50312499938547717, 99.99999999999998579 ) ) ;
#11068=CARTESIAN_POINT ( 'NONE',  ( 235.3564303562499447, -32.24062499938548143, -51.59142580818350865 ) ) ;
#11070=ORIENTED_EDGE ( 'NONE', *, *, #412, .T. ) ;
#11081=CARTESIAN_POINT ( 'NONE',  ( 229.8435696437499871, -32.87812499938547717, -51.59142580818350865 ) ) ;
#11094=CARTESIAN_POINT ( 'NONE',  ( 232.3466685930879123, -34.99995246259152282, -52.98928446312130802 ) ) ;
#11096=CARTESIAN_POINT ( 'NONE',  ( 233.9782151781249411, -30.89062499938548001, 102.3871387122750889 ) ) ;
#11106=CARTESIAN_POINT ( 'NONE',  ( 229.5999999999999375, -34.91249999999999432, 101.7320508075688679 ) ) ;
#11110=CARTESIAN_POINT ( 'NONE',  ( 235.3564303562499447, -33.59062499938548285, 98.40857419181659793 ) ) ;
#11111=CARTESIAN_POINT ( 'NONE',  ( 232.5999999999999375, -31.94062499938548072, -46.81714838363331666 ) ) ;
#11119=VERTEX_POINT ( 'NONE', #3075 ) ;
#11129=DIRECTION ( 'NONE',  ( 0.000000000000000000, 0.000000000000000000, -1.000000000000000000 ) ) ;
#11130=CARTESIAN_POINT ( 'NONE',  ( 230.8769377533405986, -32.00000000000000711, 102.1915028381723971 ) ) ;
#11131=CARTESIAN_POINT ( 'NONE',  ( 233.9782151781249411, -34.79062499938547859, 97.61286128772489690 ) ) ;
#11134=CARTESIAN_POINT ( 'NONE',  ( 235.5999999999999943, -31.10624999877096286, 101.7320508075688537 ) ) ;
#11139=AXIS2_PLACEMENT_3D ( 'NONE', #17806, #1680, #7345 ) ;
#11140=DIRECTION ( 'NONE',  ( 5.139921410301648824E-16, 1.000000000000000000, -3.597944987211154374E-15 ) ) ;
#11147=DIRECTION ( 'NONE',  ( 1.000000000000000000, -0.000000000000000000, -0.000000000000000000 ) ) ;
#11160=CARTESIAN_POINT ( 'NONE',  ( 246.9999999999999716, -5.000000000000004441, -100.0000000000000000 ) ) ;
#11163=CARTESIAN_POINT ( 'NONE',  ( 229.5999999999999375, -34.08749999999999147, -51.73205080756898866 ) ) ;
#11168=CARTESIAN_POINT ( 'NONE',  ( 232.5999999999999943, -32.61562499938548143, 96.81714838363319586 ) ) ;
#11170=CARTESIAN_POINT ( 'NONE',  ( 231.2217848218749339, -31.41562499938547859, -47.61286128772501769 ) ) ;
#11181=CARTESIAN_POINT ( 'NONE',  ( 230.2961164517930968, -35.00002705695778360, 98.07851859032987818 ) ) ;
#11185=CARTESIAN_POINT ( 'NONE',  ( 233.9782151781249411, -33.59062499938547575, -47.61286128772501769 ) ) ;
#11188=ORIENTED_EDGE ( 'NONE', *, *, #11525, .F. ) ;
#11190=CARTESIAN_POINT ( 'NONE',  ( 232.5999999999999375, -32.75624999877096144, 96.99999999999998579 ) ) ;
#11198=CARTESIAN_POINT ( 'NONE',  ( 230.4285530052381716, -35.00000000000000000, -52.07926958674877937 ) ) ;
#11200=CARTESIAN_POINT ( 'NONE',  ( 232.5999999999999375, -31.60312499938548214, 96.81714838363319586 ) ) ;
#11205=CARTESIAN_POINT ( 'NONE',  ( 233.4038475772933339, -32.83259618943232994, 96.99999999999998579 ) ) ;
#11215=CARTESIAN_POINT ( 'NONE',  ( 229.8435696437499871, -31.56562499938547717, 101.5914258081833879 ) ) ;
#11216=CARTESIAN_POINT ( 'NONE',  ( 235.3564303562499447, -32.27812499938548285, -50.00000000000011369 ) ) ;
#11221=CARTESIAN_POINT ( 'NONE',  ( 99.99999999999997158, -5.200000000000008171, 150.0000000000000000 ) ) ;
#11222=EDGE_LOOP ( 'NONE', ( #707, #14149, #5386, #8398 ) ) ;
#11232=CARTESIAN_POINT ( 'NONE',  ( 231.7961524227065411, -34.08615380933862582, -53.00000000000009237 ) ) ;
#11234=CARTESIAN_POINT ( 'NONE',  ( 235.3564303562499447, -33.92812499938548143, 98.40857419181659793 ) ) ;
#11237=CARTESIAN_POINT ( 'NONE',  ( 229.5999999999999375, -30.43124999877096215, 98.26794919243111792 ) ) ;
#11238=CARTESIAN_POINT ( 'NONE',  ( 232.5999999999999375, -31.85624999877096641, -53.46410161513786363 ) ) ;
#11240=CARTESIAN_POINT ( 'NONE',  ( 232.5999999999999375, -32.75624999877096144, 96.99999999999998579 ) ) ;
#11243=ORIENTED_EDGE ( 'NONE', *, *, #16274, .T. ) ;
#11245=CARTESIAN_POINT ( 'NONE',  ( 233.4038475772933339, -33.67634618820329706, -53.00000000000011369 ) ) ;
#11253=CARTESIAN_POINT ( 'NONE',  ( 232.5999999999999375, -29.99999999999999645, -50.00000000000011369 ) ) ;
#11261=CARTESIAN_POINT ( 'NONE',  ( 229.5999999999999375, -34.94999999999999574, -50.00000000000011369 ) ) ;
#11263=CARTESIAN_POINT ( 'NONE',  ( 231.2217848218749339, -30.66562499938547859, -52.38713871227520968 ) ) ;
#11278=CARTESIAN_POINT ( 'NONE',  ( 229.8435696437499871, -33.77812499938548285, -51.59142580818350865 ) ) ;
#11292=AXIS2_PLACEMENT_3D ( 'NONE', #11841, #14669, #1304 ) ;
#11294=CARTESIAN_POINT ( 'NONE',  ( 229.5999999999999375, -34.08749999999999147, -51.73205080756898866 ) ) ;
#11295=EDGE_CURVE ( 'NONE', #19282, #16293, #16834, .T. ) ;
#11299=CARTESIAN_POINT ( 'NONE',  ( 232.5999999999999375, -29.99999999999999645, 96.99999999999998579 ) ) ;
#11300=CARTESIAN_POINT ( 'NONE',  ( 229.8306817459157401, -31.99999999999999289, 100.2387112178437150 ) ) ;
#11302=DIRECTION ( 'NONE',  ( -0.000000000000000000, -1.000000000000000000, -0.000000000000000000 ) ) ;
#11312=CARTESIAN_POINT ( 'NONE',  ( 229.8435696437499871, -35.22676544108146857, 98.99674642581742035 ) ) ;
#11313=EDGE_CURVE ( 'NONE', #16053, #13878, #7151, .T. ) ;
#11314=CARTESIAN_POINT ( 'NONE',  ( 231.2217848218749339, -34.22812499938548569, -47.61286128772501769 ) ) ;
#11316=PLANE ( 'NONE',  #5256 ) ;
#11328=DIRECTION ( 'NONE',  ( -1.000000000000000000, 0.000000000000000000, 0.000000000000000000 ) ) ;
#11329=DIRECTION ( 'NONE',  ( 0.000000000000000000, 0.000000000000000000, -1.000000000000000000 ) ) ;
#11330=CARTESIAN_POINT ( 'NONE',  ( 105.1999999999999886, -29.80000000000001492, -97.80000000000002558 ) ) ;
#11331=CARTESIAN_POINT ( 'NONE',  ( 231.0999999999999375, -31.72499999999999787, 102.5980762113533018 ) ) ;
#11334=CARTESIAN_POINT ( 'NONE',  ( 229.5999999999999375, -33.95624999877095718, 101.7320508075688679 ) ) ;
#11335=CARTESIAN_POINT ( 'NONE',  ( 229.5999999999999375, -32.23124999877096286, -51.73205080756898866 ) ) ;
#11336=ORIENTED_EDGE ( 'NONE', *, *, #8993, .T. ) ;
#11342=CARTESIAN_POINT ( 'NONE',  ( 231.7961524227065979, -33.18615380933862724, 97.00000000000000000 ) ) ;
#11346=CARTESIAN_POINT ( 'NONE',  ( 235.3140393761304665, -32.00000000000000000, -48.72172371342785624 ) ) ;
#11347=( BOUNDED_CURVE ( )  B_SPLINE_CURVE ( 2, ( #9473, #4998, #1953, #8007, #13966, #698, #9674, #11232, #2048 ),
 .UNSPECIFIED., .F., .F. ) 
 B_SPLINE_CURVE_WITH_KNOTS ( ( 3, 2, 2, 2, 3 ),
 ( 0.6458333333333331483, 0.6527777777777777901, 0.6666666666666666297, 0.6805555555555555802, 0.6874999999999997780 ),
 .UNSPECIFIED. ) 
 CURVE ( )  GEOMETRIC_REPRESENTATION_ITEM ( )  RATIONAL_B_SPLINE_CURVE ( ( 0.9330127018922194093, 0.9330127018922177440, 1.000000000000000000, 0.8660254037844387076, 1.000000000000000000, 0.8660254037844387076, 1.000000000000000000, 0.9330127018922215187, 0.9330127018922194093 ) ) 
 REPRESENTATION_ITEM ( '' )  );
#11351=CARTESIAN_POINT ( 'NONE',  ( 234.1999394931801532, -31.99999999999997868, -52.45377063617920754 ) ) ;
#11356=ORIENTED_EDGE ( 'NONE', *, *, #9427, .T. ) ;
#11357=DIRECTION ( 'NONE',  ( -0.000000000000000000, -1.000000000000000000, -0.000000000000000000 ) ) ;
#11358=CARTESIAN_POINT ( 'NONE',  ( 233.9419434205216533, -34.99999999999999289, 97.38506107425222069 ) ) ;
#11360=CARTESIAN_POINT ( 'NONE',  ( 231.2217848218749339, -34.67812499938548143, 102.3871387122750889 ) ) ;
#11362=CARTESIAN_POINT ( 'NONE',  ( 232.5999999999999375, -35.09062499938547575, -46.81714838363331666 ) ) ;
#11376=CARTESIAN_POINT ( 'NONE',  ( 229.8435696437499871, -33.32812499938548001, -51.59142580818350865 ) ) ;
#11392=( BOUNDED_CURVE ( )  B_SPLINE_CURVE ( 2, ( #17587, #8492, #3808, #6760, #898, #11622, #1178, #14447, #11240 ),
 .UNSPECIFIED., .F., .F. ) 
 B_SPLINE_CURVE_WITH_KNOTS ( ( 3, 2, 2, 2, 3 ),
 ( 0.3958333333333333703, 0.4027777777777777901, 0.4166666666666666852, 0.4305555555555555802, 0.4375000000000001110 ),
 .UNSPECIFIED. ) 
 CURVE ( )  GEOMETRIC_REPRESENTATION_ITEM ( )  RATIONAL_B_SPLINE_CURVE ( ( 0.9330127018922194093, 0.9330127018922196314, 1.000000000000000000, 0.8660254037844387076, 1.000000000000000000, 0.8660254037844387076, 1.000000000000000000, 0.9330127018922182991, 0.9330127018922194093 ) ) 
 REPRESENTATION_ITEM ( '' )  );
#11402=CARTESIAN_POINT ( 'NONE',  ( 229.5999999999999375, -34.89374999877096428, -50.00000000000011369 ) ) ;
#11404=CARTESIAN_POINT ( 'NONE',  ( 231.0999999999999375, -33.97500000000000142, 102.5980762113533018 ) ) ;
#11409=CARTESIAN_POINT ( 'NONE',  ( 235.3564303562499447, -34.97812499938547859, 99.99999999999998579 ) ) ;
#11410=CARTESIAN_POINT ( 'NONE',  ( 229.8435696437499871, -32.99062499938548143, -51.59142580818350865 ) ) ;
#11411=LINE ( 'NONE', #16098, #16162 ) ;
#11413=DIRECTION ( 'NONE',  ( 1.000000000000000000, 0.000000000000000000, -0.000000000000000000 ) ) ;
#11427=CARTESIAN_POINT ( 'NONE',  ( 230.8788704469753839, -35.00000000000000000, 97.53419980903893816 ) ) ;
#11429=CARTESIAN_POINT ( 'NONE',  ( 229.5999999999999375, -30.89999999999999858, 99.99999999999998579 ) ) ;
#11434=CARTESIAN_POINT ( 'NONE',  ( 229.5999999999999375, -32.15624999877096002, 101.7320508075688679 ) ) ;
#11435=CARTESIAN_POINT ( 'NONE',  ( 232.5999999999999375, -30.50624999877096144, -53.46410161513786363 ) ) ;
#11441=CARTESIAN_POINT ( 'NONE',  ( 235.5999999999999375, -33.76874999877096428, -50.00000000000011369 ) ) ;
#11452=LINE ( 'NONE', #11733, #3379 ) ;
#11455=ORIENTED_EDGE ( 'NONE', *, *, #19036, .F. ) ;
#11457=CARTESIAN_POINT ( 'NONE',  ( 234.0999999999999375, -34.35000000000000142, -47.40192378864679768 ) ) ;
#11459=DIRECTION ( 'NONE',  ( 0.000000000000000000, 0.000000000000000000, -1.000000000000000000 ) ) ;
#11461=CARTESIAN_POINT ( 'NONE',  ( 231.2217848218749339, -30.51562499938548001, -47.61286128772501769 ) ) ;
#11464=ORIENTED_EDGE ( 'NONE', *, *, #17948, .T. ) ;
#11475=CARTESIAN_POINT ( 'NONE',  ( 231.2217848218749339, -34.11562499938548143, -47.61286128772501769 ) ) ;
#11486=DIRECTION ( 'NONE',  ( 5.139921410301648824E-16, 1.000000000000000000, 0.000000000000000000 ) ) ;
#11498=DIRECTION ( 'NONE',  ( -0.000000000000000000, -1.000000000000000000, -0.000000000000000000 ) ) ;
#11503=EDGE_CURVE ( 'NONE', #3766, #9169, #15773, .T. ) ;
#11504=EDGE_LOOP ( 'NONE', ( #878, #18818, #14788, #14111, #18084, #16675, #3048, #10827, #2952, #7707, #16560, #14735, #3038, #2035, #5846, #9195, #14427 ) ) ;
#11507=CARTESIAN_POINT ( 'NONE',  ( 229.8435696437499303, -34.30312499938548143, 99.99999999999998579 ) ) ;
#11508=CARTESIAN_POINT ( 'NONE',  ( 235.3564303562499447, -32.24062499938548143, -51.59142580818350865 ) ) ;
#11513=LINE ( 'NONE', #15816, #10056 ) ;
#11525=EDGE_CURVE ( 'NONE', #13878, #10068, #5484, .T. ) ;
#11527=CARTESIAN_POINT ( 'NONE',  ( 235.5999999999999943, -31.08749999999999503, 98.26794919243110371 ) ) ;
#11529=VERTEX_POINT ( 'NONE', #4240 ) ;
#11530=CARTESIAN_POINT ( 'NONE',  ( 235.5999999999999943, -33.28124999877096002, 98.26794919243110371 ) ) ;
#11531=CARTESIAN_POINT ( 'NONE',  ( 229.5999999999999375, -30.39374999877096428, -50.00000000000011369 ) ) ;
#11545=EDGE_CURVE ( 'NONE', #1971, #14449, #6580, .T. ) ;
#11553=CARTESIAN_POINT ( 'NONE',  ( 235.3594282536526237, -35.00000000000000000, 100.3964642588227605 ) ) ;
#11559=CARTESIAN_POINT ( 'NONE',  ( 231.2217848218749339, -30.96562499938547930, -47.61286128772501769 ) ) ;
#11565=CARTESIAN_POINT ( 'NONE',  ( 233.9782151781249411, -30.74062499938547788, 97.61286128772489690 ) ) ;
#11571=CARTESIAN_POINT ( 'NONE',  ( 231.1166048115126443, -35.16733441503057378, -52.52040863755893696 ) ) ;
#11582=CARTESIAN_POINT ( 'NONE',  ( 233.9782151781249411, -32.24062499938548143, 102.3871387122750889 ) ) ;
#11596=CARTESIAN_POINT ( 'NONE',  ( 229.8435696437499871, -34.71562499938548285, 101.5914258081833879 ) ) ;
#11598=DIRECTION ( 'NONE',  ( 0.000000000000000000, 0.000000000000000000, 1.000000000000000000 ) ) ;
#11602=DIRECTION ( 'NONE',  ( 0.000000000000000000, -0.000000000000000000, -1.000000000000000000 ) ) ;
#11611=EDGE_CURVE ( 'NONE', #12372, #12231, #9529, .T. ) ;
#11613=CARTESIAN_POINT ( 'NONE',  ( 232.1454721953969056, -34.99999999999999289, 102.7245357809972290 ) ) ;
#11615=CARTESIAN_POINT ( 'NONE',  ( 234.0999999999999375, -31.64999999999999858, 102.5980762113533018 ) ) ;
#11619=CARTESIAN_POINT ( 'NONE',  ( 232.5999999999999375, -34.55624999877095860, 97.00000000000000000 ) ) ;
#11620=CARTESIAN_POINT ( 'NONE',  ( 234.0999999999999375, -32.49374999877096570, 102.5980762113533018 ) ) ;
#11621=CARTESIAN_POINT ( 'NONE',  ( 231.0999999999999375, -34.06874999877096144, -52.59807621135342970 ) ) ;
#11622=CARTESIAN_POINT ( 'NONE',  ( 229.5999999999999375, -32.68124999877096570, 98.26794919243111792 ) ) ;
#11624=ORIENTED_EDGE ( 'NONE', *, *, #2917, .F. ) ;
#11625=VERTEX_POINT ( 'NONE', #15854 ) ;
#11630=FACE_OUTER_BOUND ( 'NONE', #10819, .T. ) ;
#11631=ORIENTED_EDGE ( 'NONE', *, *, #4099, .T. ) ;
#11639=CARTESIAN_POINT ( 'NONE',  ( 232.5999999999999375, -32.30624999877096570, -53.00000000000011369 ) ) ;
#11643=VECTOR ( 'NONE', #16085, 1000.000000000000000 ) ;
#11644=CARTESIAN_POINT ( 'NONE',  ( 229.8435696437499871, -30.17812499938547433, 98.40857419181659793 ) ) ;
#11650=CARTESIAN_POINT ( 'NONE',  ( 232.5999999999999943, -33.74062499938548143, 103.1828516163667899 ) ) ;
#11652=CARTESIAN_POINT ( 'NONE',  ( 99.99999999999997158, -5.200000000000008171, -100.0000000000000000 ) ) ;
#11653=CARTESIAN_POINT ( 'NONE',  ( 232.5999999999999375, -33.62812499938547717, -46.81714838363331666 ) ) ;
#11659=CARTESIAN_POINT ( 'NONE',  ( 235.3564303562499447, -31.26562499938547646, 99.99999999999998579 ) ) ;
#11661=ADVANCED_FACE ( 'NONE', ( #4973 ), #9650, .T. ) ;
#11666=CARTESIAN_POINT ( 'NONE',  ( 235.3564303562499447, -34.37812499938547717, -51.59142580818350865 ) ) ;
#11673=CARTESIAN_POINT ( 'NONE',  ( 235.3564303562499447, -31.37812499938547717, -50.00000000000011369 ) ) ;
#11677=CARTESIAN_POINT ( 'NONE',  ( 229.8435696437499587, -32.42812499938548143, 98.40857419181659793 ) ) ;
#11678=PLANE ( 'NONE',  #3293 ) ;
#11681=CARTESIAN_POINT ( 'NONE',  ( 231.4702054326072016, -32.00000000000000711, -47.41965524898115092 ) ) ;
#11683=CARTESIAN_POINT ( 'NONE',  ( 230.7186334667983658, -32.00000000000000711, 97.98546077809203325 ) ) ;
#11688=ORIENTED_EDGE ( 'NONE', *, *, #17389, .T. ) ;
#11690=CARTESIAN_POINT ( 'NONE',  ( 232.5999999999999375, -34.86562499938548143, 96.81714838363319586 ) ) ;
#11691=CARTESIAN_POINT ( 'NONE',  ( 235.3564303562499447, -34.49062499938548143, -51.59142580818350865 ) ) ;
#11693=DIRECTION ( 'NONE',  ( 1.000000000000000000, 0.000000000000000000, 0.000000000000000000 ) ) ;
#11694=VERTEX_POINT ( 'NONE', #5260 ) ;
#11698=CARTESIAN_POINT ( 'NONE',  ( 229.5999999999999375, -33.56249999999999289, -48.26794919243123161 ) ) ;
#11702=CARTESIAN_POINT ( 'NONE',  ( 229.8435696437499871, -32.54062499938547859, 98.40857419181659793 ) ) ;
#11707=PLANE ( 'NONE',  #274 ) ;
#11711=CARTESIAN_POINT ( 'NONE',  ( 229.5999999999999375, -32.28750000000000142, 98.26794919243111792 ) ) ;
#11713=DIRECTION ( 'NONE',  ( -1.000000000000000000, 0.000000000000000000, 0.000000000000000000 ) ) ;
#11715=CARTESIAN_POINT ( 'NONE',  ( 232.5999999999999375, -31.85624999877096641, 96.53589838486223584 ) ) ;
#11716=CARTESIAN_POINT ( 'NONE',  ( 235.5999999999999943, -34.25624999877096855, -48.26794919243124582 ) ) ;
#11719=EDGE_LOOP ( 'NONE', ( #8473, #6238, #18911, #6416 ) ) ;
#11726=CARTESIAN_POINT ( 'NONE',  ( 244.7999999999999545, -35.00000000000000000, -97.80000000000002558 ) ) ;
#11727=EDGE_CURVE ( 'NONE', #10663, #138, #8078, .T. ) ;
#11730=CARTESIAN_POINT ( 'NONE',  ( 235.5999999999999943, -32.45624999877096428, -48.26794919243124582 ) ) ;
#11733=CARTESIAN_POINT ( 'NONE',  ( 105.1999999999999744, -34.99999999999999289, -100.0000000000000000 ) ) ;
#11738=DIRECTION ( 'NONE',  ( 1.000000000000000000, 0.000000000000000000, 0.000000000000000000 ) ) ;
#11740=CARTESIAN_POINT ( 'NONE',  ( 235.5999999999999943, -33.35624999877096286, -48.26794919243124582 ) ) ;
#11741=ADVANCED_FACE ( 'NONE', ( #4169, #19212, #9937 ), #14701, .T. ) ;
#11742=DIRECTION ( 'NONE',  ( 1.000000000000000000, -4.970554372426382520E-17, -0.000000000000000000 ) ) ;
#11746=CARTESIAN_POINT ( 'NONE',  ( 233.9782151781249411, -31.79062499938548214, -47.61286128772501769 ) ) ;
#11754=LINE ( 'NONE', #2864, #5877 ) ;
#11755=CARTESIAN_POINT ( 'NONE',  ( 229.8435696437499303, -31.94062499938547717, 99.99999999999998579 ) ) ;
#11756=CARTESIAN_POINT ( 'NONE',  ( 229.8435696437499587, -33.77812499938547575, -51.59142580818350154 ) ) ;
#11760=CARTESIAN_POINT ( 'NONE',  ( 235.5999999999999943, -31.08749999999999503, -51.73205080756900287 ) ) ;
#11762=AXIS2_PLACEMENT_3D ( 'NONE', #10298, #6172, #16711 ) ;
#11763=ORIENTED_EDGE ( 'NONE', *, *, #18919, .T. ) ;
#11766=CARTESIAN_POINT ( 'NONE',  ( 231.2217848218749339, -31.97812499938548214, -47.61286128772501769 ) ) ;
#11768=ORIENTED_EDGE ( 'NONE', *, *, #13046, .F. ) ;
#11772=CARTESIAN_POINT ( 'NONE',  ( 230.2961164517930968, -35.00002705695767702, -51.92148140967023551 ) ) ;
#11775=VECTOR ( 'NONE', #11357, 1000.000000000000000 ) ;
#11778=LINE ( 'NONE', #6115, #5250 ) ;
#11783=VECTOR ( 'NONE', #1769, 1000.000000000000000 ) ;
#11784=CARTESIAN_POINT ( 'NONE',  ( 244.7999999999999545, -4.999999999999976907, 153.0000000000000000 ) ) ;
#11789=DIRECTION ( 'NONE',  ( 0.000000000000000000, 0.000000000000000000, -1.000000000000000000 ) ) ;
#11791=AXIS2_PLACEMENT_3D ( 'NONE', #13426, #7561, #17926 ) ;
#11792=AXIS2_PLACEMENT_3D ( 'NONE', #6888, #16587, #12838 ) ;
#11797=DIRECTION ( 'NONE',  ( 0.000000000000000000, -1.261617073437673828E-14, -1.000000000000000000 ) ) ;
#11798=VERTEX_POINT ( 'NONE', #2796 ) ;
#11800=CARTESIAN_POINT ( 'NONE',  ( 231.0999999999999375, -33.52499999999999147, -47.40192378864679768 ) ) ;
#11801=AXIS2_PLACEMENT_3D ( 'NONE', #16915, #9482, #6563 ) ;
#11805=CARTESIAN_POINT ( 'NONE',  ( 235.3564303562499447, -32.72812499938547859, 99.99999999999998579 ) ) ;
#11810=DIRECTION ( 'NONE',  ( 0.000000000000000000, 0.000000000000000000, 1.000000000000000000 ) ) ;
#11813=CARTESIAN_POINT ( 'NONE',  ( 234.0999999999999375, -34.64999999999999147, 97.40192378864668399 ) ) ;
#11815=CARTESIAN_POINT ( 'NONE',  ( 235.5999999999999943, -34.63124999877096144, 98.26794919243110371 ) ) ;
#11816=CARTESIAN_POINT ( 'NONE',  ( 231.0999999999999375, -34.96874999877096002, 97.40192378864668399 ) ) ;
#11817=CARTESIAN_POINT ( 'NONE',  ( 232.5999999999999375, -34.55624999877095860, -53.46410161513786363 ) ) ;
#11822=CARTESIAN_POINT ( 'NONE',  ( 99.99999999999997158, -5.200000000000008171, 150.0000000000000000 ) ) ;
#11824=ORIENTED_EDGE ( 'NONE', *, *, #15198, .T. ) ;
#11841=CARTESIAN_POINT ( 'NONE',  ( 232.5999999999999375, -29.99999999999999645, 99.99999999999998579 ) ) ;
#11842=CARTESIAN_POINT ( 'NONE',  ( 235.3564303562499447, -31.75312499938547717, -48.40857419181671162 ) ) ;
#11850=CARTESIAN_POINT ( 'NONE',  ( 231.2217848218749339, -33.21562499938547575, 102.3871387122750889 ) ) ;
#11851=CARTESIAN_POINT ( 'NONE',  ( 235.3564303562499447, -33.51562499938548001, -50.00000000000011369 ) ) ;
#11855=CARTESIAN_POINT ( 'NONE',  ( 233.9782151781249411, -34.49062499938548143, -47.61286128772501769 ) ) ;
#11858=EDGE_CURVE ( 'NONE', #12080, #11529, #7285, .T. ) ;
#11862=CARTESIAN_POINT ( 'NONE',  ( 232.5999999999999375, -31.49062499938547788, -46.81714838363331666 ) ) ;
#11871=CARTESIAN_POINT ( 'NONE',  ( 231.9083760470965103, -32.00000000000000711, -47.24830349208670555 ) ) ;
#11876=CARTESIAN_POINT ( 'NONE',  ( 244.7999999999999545, -5.000000000000000888, -103.0000000000000995 ) ) ;
#11890=DIRECTION ( 'NONE',  ( 1.000000000000000000, 0.000000000000000000, -0.000000000000000000 ) ) ;
#11892=DIRECTION ( 'NONE',  ( -0.000000000000000000, -1.000000000000000000, -0.000000000000000000 ) ) ;
#11894=CARTESIAN_POINT ( 'NONE',  ( 231.2217848218749339, -31.67812499938547788, 97.61286128772489690 ) ) ;
#11901=CARTESIAN_POINT ( 'NONE',  ( 235.5999999999999943, -33.28124999877096002, 98.26794919243110371 ) ) ;
#11904=CARTESIAN_POINT ( 'NONE',  ( 235.5999999999999375, -33.82499999999999574, 99.99999999999998579 ) ) ;
#11905=ORIENTED_EDGE ( 'NONE', *, *, #2920, .F. ) ;
#11907=CARTESIAN_POINT ( 'NONE',  ( 234.0999999999999375, -35.04374999877096286, 97.40192378864668399 ) ) ;
#11908=CARTESIAN_POINT ( 'NONE',  ( 231.0999999999999375, -32.71874999877096002, -52.59807621135342970 ) ) ;
#11910=ORIENTED_EDGE ( 'NONE', *, *, #9832, .T. ) ;
#11917=CARTESIAN_POINT ( 'NONE',  ( 105.1999999999999886, -29.79999999999999361, -100.0000000000000000 ) ) ;
#11920=VECTOR ( 'NONE', #11140, 1000.000000000000000 ) ;
#11924=CYLINDRICAL_SURFACE ( 'NONE', #14129, 3.000000000000002665 ) ;
#11928=DIRECTION ( 'NONE',  ( 0.000000000000000000, 0.000000000000000000, 1.000000000000000000 ) ) ;
#11929=VERTEX_POINT ( 'NONE', #17938 ) ;
#11934=CARTESIAN_POINT ( 'NONE',  ( 235.5999999999999943, -34.70624999877096428, -48.26794919243124582 ) ) ;
#11935=CARTESIAN_POINT ( 'NONE',  ( 232.5999999999999375, -29.99999999999999645, -47.00000000000010658 ) ) ;
#11938=CARTESIAN_POINT ( 'NONE',  ( 235.3564303562499447, -33.06562499938547717, -50.00000000000011369 ) ) ;
#11947=CARTESIAN_POINT ( 'NONE',  ( 229.8435696437499871, -34.15312499938547575, 101.5914258081833879 ) ) ;
#11948=CARTESIAN_POINT ( 'NONE',  ( 233.9782151781249411, -34.49062499938548143, -47.61286128772501769 ) ) ;
#11952=CARTESIAN_POINT ( 'NONE',  ( 234.0999999999999375, -30.29999999999999716, -47.40192378864679768 ) ) ;
#11978=DIRECTION ( 'NONE',  ( 0.000000000000000000, 0.000000000000000000, -1.000000000000000000 ) ) ;
#11979=CARTESIAN_POINT ( 'NONE',  ( 235.3564303562499447, -34.97812499938547859, -50.00000000000011369 ) ) ;
#11982=EDGE_CURVE ( 'NONE', #12892, #10996, #4698, .T. ) ;
#11984=FACE_OUTER_BOUND ( 'NONE', #9579, .T. ) ;
#11985=VERTEX_POINT ( 'NONE', #7574 ) ;
#11986=EDGE_CURVE ( 'NONE', #15818, #11985, #6784, .T. ) ;
#11992=CARTESIAN_POINT ( 'NONE',  ( 229.8435696437499871, -31.56562499938547717, 101.5914258081833879 ) ) ;
#12000=CARTESIAN_POINT ( 'NONE',  ( 235.5999999999999943, -32.96249999999999858, 101.7320508075688537 ) ) ;
#12002=CARTESIAN_POINT ( 'NONE',  ( 233.9782151781249411, -34.45312499938548001, -52.38713871227520968 ) ) ;
#12004=CARTESIAN_POINT ( 'NONE',  ( 234.0999999999999375, -35.19374999877096855, 102.5980762113533018 ) ) ;
#12005=CARTESIAN_POINT ( 'NONE',  ( 231.0999999999999375, -33.46874999877096002, -47.40192378864679768 ) ) ;
#12009=CARTESIAN_POINT ( 'NONE',  ( 105.1999999999999744, -34.99999999999999289, -100.0000000000000000 ) ) ;
#12014=AXIS2_PLACEMENT_3D ( 'NONE', #9882, #11147, #18777 ) ;
#12017=( BOUNDED_CURVE ( )  B_SPLINE_CURVE ( 2, ( #12133, #1771, #18002, #10285, #16338, #2947, #8901, #13690, #14966 ),
 .UNSPECIFIED., .F., .F. ) 
 B_SPLINE_CURVE_WITH_KNOTS ( ( 3, 2, 2, 2, 3 ),
 ( 0.7291666666666665186, 0.7361111111111111605, 0.7500000000000000000, 0.7638888888888888395, 0.7708333333333332593 ),
 .UNSPECIFIED. ) 
 CURVE ( )  GEOMETRIC_REPRESENTATION_ITEM ( )  RATIONAL_B_SPLINE_CURVE ( ( 0.9330127018922194093, 0.9330127018922177440, 1.000000000000000000, 0.8660254037844387076, 1.000000000000000000, 0.8660254037844387076, 1.000000000000000000, 0.9330127018922198534, 0.9330127018922192983 ) ) 
 REPRESENTATION_ITEM ( '' )  );
#12024=CARTESIAN_POINT ( 'NONE',  ( 232.5999999999999375, -30.47812499938547859, 103.1828516163667899 ) ) ;
#12025=ORIENTED_EDGE ( 'NONE', *, *, #17619, .T. ) ;
#12026=( NAMED_UNIT ( * ) PLANE_ANGLE_UNIT ( ) SI_UNIT ( $, .RADIAN. ) );
#12029=AXIS2_PLACEMENT_3D ( 'NONE', #13009, #18978, #5602 ) ;
#12034=CARTESIAN_POINT ( 'NONE',  ( 232.5999999999999375, -32.50312499938547717, -53.18285161636690361 ) ) ;
#12036=ORIENTED_EDGE ( 'NONE', *, *, #1235, .F. ) ;
#12042=CARTESIAN_POINT ( 'NONE',  ( 229.8435696437499871, -33.25312499938547717, 101.5914258081833879 ) ) ;
#12049=CARTESIAN_POINT ( 'NONE',  ( 232.5999999999999375, -32.58749999999999858, -46.53589838486234953 ) ) ;
#12054=CARTESIAN_POINT ( 'NONE',  ( 229.8435696437499303, -31.15312499938548285, -50.00000000000011369 ) ) ;
#12059=EDGE_CURVE ( 'NONE', #15031, #12702, #6697, .T. ) ;
#12061=CYLINDRICAL_SURFACE ( 'NONE', #1014, 3.000000000000009770 ) ;
#12076=CARTESIAN_POINT ( 'NONE',  ( 244.7999999999999545, -4.999999999999976907, 153.0000000000000000 ) ) ;
#12080=VERTEX_POINT ( 'NONE', #16949 ) ;
#12083=( BOUNDED_CURVE ( )  B_SPLINE_CURVE ( 2, ( #5462, #16091, #11404, #17366, #2697, #1054, #14511, #7105, #13061 ),
 .UNSPECIFIED., .F., .F. ) 
 B_SPLINE_CURVE_WITH_KNOTS ( ( 3, 2, 2, 2, 3 ),
 ( 0.7291666666666667407, 0.7361111111111111605, 0.7500000000000000000, 0.7638888888888888395, 0.7708333333333332593 ),
 .UNSPECIFIED. ) 
 CURVE ( )  GEOMETRIC_REPRESENTATION_ITEM ( )  RATIONAL_B_SPLINE_CURVE ( ( 0.9330127018922192983, 0.9330127018922198534, 1.000000000000000000, 0.8660254037844387076, 1.000000000000000000, 0.8660254037844387076, 1.000000000000000000, 0.9330127018922198534, 0.9330127018922192983 ) ) 
 REPRESENTATION_ITEM ( '' )  );
#12087=CARTESIAN_POINT ( 'NONE',  ( 232.5999999999999375, -33.65624999877096002, -53.00000000000011369 ) ) ;
#12088=CARTESIAN_POINT ( 'NONE',  ( 235.3564303562499447, -30.92812499938547788, 99.99999999999998579 ) ) ;
#12090=AXIS2_PLACEMENT_3D ( 'NONE', #13685, #6276, #3616 ) ;
#12094=FACE_OUTER_BOUND ( 'NONE', #15746, .T. ) ;
#12098=CARTESIAN_POINT ( 'NONE',  ( 232.5999999999999375, -33.03749999999999432, 103.4641016151377499 ) ) ;
#12099=ORIENTED_EDGE ( 'NONE', *, *, #10930, .T. ) ;
#12100=CARTESIAN_POINT ( 'NONE',  ( 235.3564303562499447, -34.52812499938547575, -50.00000000000011369 ) ) ;
#12102=CARTESIAN_POINT ( 'NONE',  ( 235.5999999999999375, -34.21874999877096002, 99.99999999999998579 ) ) ;
#12103=CARTESIAN_POINT ( 'NONE',  ( 233.9782151781249411, -30.55312499938548143, -47.61286128772501769 ) ) ;
#12108=ORIENTED_EDGE ( 'NONE', *, *, #15340, .F. ) ;
#12109=CARTESIAN_POINT ( 'NONE',  ( 231.0999999999999375, -32.71874999877096002, -52.59807621135342970 ) ) ;
#12114=CARTESIAN_POINT ( 'NONE',  ( 235.5999999999999375, -32.47499999999999432, 99.99999999999998579 ) ) ;
#12121=CARTESIAN_POINT ( 'NONE',  ( 244.7999999999999545, -4.999999999999976907, 150.0000000000000000 ) ) ;
#12127=CARTESIAN_POINT ( 'NONE',  ( 229.8435696437499303, -31.49062499938547788, 99.99999999999998579 ) ) ;
#12129=SURFACE_STYLE_FILL_AREA ( #9000 ) ;
#12133=CARTESIAN_POINT ( 'NONE',  ( 232.5999999999999375, -34.33124999877097139, 102.9999999999999858 ) ) ;
#12134=CARTESIAN_POINT ( 'NONE',  ( 229.9986727058519307, -35.00000000000000711, -48.78874432549886819 ) ) ;
#12135=CARTESIAN_POINT ( 'NONE',  ( 229.8435696437499303, -34.19062499938547717, -50.00000000000011369 ) ) ;
#12138=DIRECTION ( 'NONE',  ( 0.000000000000000000, 0.000000000000000000, -1.000000000000000000 ) ) ;
#12144=CARTESIAN_POINT ( 'NONE',  ( 235.3564303562499447, -34.90312499938547575, 101.5914258081833879 ) ) ;
#12150=CARTESIAN_POINT ( 'NONE',  ( 231.0999999999999375, -31.87499999999999289, -52.59807621135342970 ) ) ;
#12156=CARTESIAN_POINT ( 'NONE',  ( 232.5999999999999375, -33.74062499938548143, -46.81714838363331666 ) ) ;
#12158=ORIENTED_EDGE ( 'NONE', *, *, #16274, .F. ) ;
#12160=CARTESIAN_POINT ( 'NONE',  ( 229.8435696437499303, -33.74062499938548143, 99.99999999999998579 ) ) ;
#12168=CARTESIAN_POINT ( 'NONE',  ( 233.9782151781249411, -31.64062499938547646, -52.38713871227520968 ) ) ;
#12171=PRODUCT_DEFINITION_CONTEXT ( 'detailed design', #19198, 'design' ) ;
#12181=CARTESIAN_POINT ( 'NONE',  ( 105.2000000000110020, -34.99999999999999289, -100.0000000000000000 ) ) ;
#12184=CARTESIAN_POINT ( 'NONE',  ( 232.5999999999999375, -33.51562499938548001, 96.81714838363319586 ) ) ;
#12187=DIRECTION ( 'NONE',  ( 1.000000000000000000, -4.625929269271524001E-17, -6.308085367188448025E-15 ) ) ;
#12189=LINE ( 'NONE', #10723, #2755 ) ;
#12192=CARTESIAN_POINT ( 'NONE',  ( 234.0999999999999375, -33.74999999999999289, 97.40192378864668399 ) ) ;
#12193=ORIENTED_EDGE ( 'NONE', *, *, #12336, .F. ) ;
#12194=CARTESIAN_POINT ( 'NONE',  ( 235.3564303562499447, -33.59062499938547575, -51.59142580818350154 ) ) ;
#12196=CARTESIAN_POINT ( 'NONE',  ( 229.5999999999999375, -35.30624999877095860, 101.7320508075688679 ) ) ;
#12197=CARTESIAN_POINT ( 'NONE',  ( 231.0999999999999375, -34.81874999877096144, -47.40192378864679768 ) ) ;
#12199=DIRECTION ( 'NONE',  ( 0.000000000000000000, 0.000000000000000000, 1.000000000000000000 ) ) ;
#12201=ORIENTED_EDGE ( 'NONE', *, *, #12713, .F. ) ;
#12205=ORIENTED_EDGE ( 'NONE', *, *, #8320, .F. ) ;
#12214=ADVANCED_FACE ( 'NONE', ( #623 ), #5305, .T. ) ;
#12217=CYLINDRICAL_SURFACE ( 'NONE', #5279, 3.000000000000009770 ) ;
#12218=CARTESIAN_POINT ( 'NONE',  ( 233.9782151781249411, -31.79062499938548214, 102.3871387122750889 ) ) ;
#12219=VERTEX_POINT ( 'NONE', #9691 ) ;
#12222=VERTEX_POINT ( 'NONE', #17213 ) ;
#12225=CARTESIAN_POINT ( 'NONE',  ( 230.0248882325211923, -35.00000000000002132, -51.51699773205431399 ) ) ;
#12231=VERTEX_POINT ( 'NONE', #8317 ) ;
#12235=ADVANCED_FACE ( 'NONE', ( #5202 ), #8228, .F. ) ;
#12239=CARTESIAN_POINT ( 'NONE',  ( 233.9782151781249411, -34.94062499938547717, 102.3871387122750889 ) ) ;
#12246=CARTESIAN_POINT ( 'NONE',  ( 235.5999999999999375, -33.82499999999999574, -50.00000000000011369 ) ) ;
#12251=CARTESIAN_POINT ( 'NONE',  ( 233.9782151781249411, -34.15312499938547575, -47.61286128772501769 ) ) ;
#12253=ORIENTED_EDGE ( 'NONE', *, *, #11986, .F. ) ;
#12255=VECTOR ( 'NONE', #2735, 1000.000000000000000 ) ;
#12256=( BOUNDED_CURVE ( )  B_SPLINE_CURVE ( 2, ( #3125, #24, #15048, #13391, #214, #6171, #7623, #13576, #18091 ),
 .UNSPECIFIED., .F., .F. ) 
 B_SPLINE_CURVE_WITH_KNOTS ( ( 3, 2, 2, 2, 3 ),
 ( 0.6458333333333332593, 0.6527777777777777901, 0.6666666666666666297, 0.6805555555555555802, 0.6875000000000000000 ),
 .UNSPECIFIED. ) 
 CURVE ( )  GEOMETRIC_REPRESENTATION_ITEM ( )  RATIONAL_B_SPLINE_CURVE ( ( 0.9330127018922192983, 0.9330127018922187432, 1.000000000000000000, 0.8660254037844387076, 1.000000000000000000, 0.8660254037844387076, 1.000000000000000000, 0.9330127018922194093, 0.9330127018922194093 ) ) 
 REPRESENTATION_ITEM ( '' )  );
#12262=CARTESIAN_POINT ( 'NONE',  ( 230.3249173797030096, -32.00000000000000000, -48.43364869553379037 ) ) ;
#12268=CARTESIAN_POINT ( 'NONE',  ( 229.8435696437499871, -30.55312499938547788, -48.40857419181671162 ) ) ;
#12274=CARTESIAN_POINT ( 'NONE',  ( 234.0999999999999375, -34.35000000000000142, 102.5980762113533018 ) ) ;
#12284=CARTESIAN_POINT ( 'NONE',  ( 235.3564303562499447, -33.14062499938548001, 98.40857419181659793 ) ) ;
#12287=CARTESIAN_POINT ( 'NONE',  ( 229.5999999999999375, -32.73749999999999716, 98.26794919243111792 ) ) ;
#12290=PLANE ( 'NONE',  #13045 ) ;
#12295=CARTESIAN_POINT ( 'NONE',  ( 235.3564303562499447, -33.17812499938548143, -50.00000000000011369 ) ) ;
#12297=CARTESIAN_POINT ( 'NONE',  ( 229.8435696437499303, -32.50312499938547717, 99.99999999999998579 ) ) ;
#12298=CARTESIAN_POINT ( 'NONE',  ( 229.5999999999999943, -35.36739044046695568, -51.09190523015522700 ) ) ;
#12314=CARTESIAN_POINT ( 'NONE',  ( 105.1999999999999744, -31.99999999999999289, 153.0000000000000000 ) ) ;
#12315=CARTESIAN_POINT ( 'NONE',  ( 233.9782151781249411, -33.44062499938547717, 97.61286128772489690 ) ) ;
#12316=CARTESIAN_POINT ( 'NONE',  ( 233.9782151781249411, -32.69062499938547717, 102.3871387122750889 ) ) ;
#12317=VERTEX_POINT ( 'NONE', #11346 ) ;
#12318=( NAMED_UNIT ( * ) PLANE_ANGLE_UNIT ( ) SI_UNIT ( $, .RADIAN. ) );
#12320=CARTESIAN_POINT ( 'NONE',  ( 229.5999999999999375, -32.15624999877096002, 101.7320508075688821 ) ) ;
#12325=ORIENTED_EDGE ( 'NONE', *, *, #14019, .T. ) ;
#12326=CARTESIAN_POINT ( 'NONE',  ( 229.8435696437499871, -34.67812499938547433, -51.59142580818350865 ) ) ;
#12336=EDGE_CURVE ( 'NONE', #13758, #13209, #15846, .T. ) ;
#12343=CARTESIAN_POINT ( 'NONE',  ( 235.5999999999999375, -31.57499999999999218, -50.00000000000011369 ) ) ;
#12346=DIRECTION ( 'NONE',  ( -0.000000000000000000, -1.000000000000000000, -0.000000000000000000 ) ) ;
#12348=CARTESIAN_POINT ( 'NONE',  ( 229.8435696437499303, -32.95312499938548001, -50.00000000000011369 ) ) ;
#12355=CARTESIAN_POINT ( 'NONE',  ( 229.8787539177867814, -32.00000000000002132, -50.47355695758027139 ) ) ;
#12362=CARTESIAN_POINT ( 'NONE',  ( 232.5999999999999375, -30.92812499938547433, -46.81714838363331666 ) ) ;
#12369=( BOUNDED_CURVE ( )  B_SPLINE_CURVE ( 2, ( #12530, #9604, #15569, #2467, #6877 ),
 .UNSPECIFIED., .F., .F. ) 
 B_SPLINE_CURVE_WITH_KNOTS ( ( 3, 2, 3 ),
 ( 0.2975293541897500171, 0.3055555555555555802, 0.3125000000000000555 ),
 .UNSPECIFIED. ) 
 CURVE ( )  GEOMETRIC_REPRESENTATION_ITEM ( )  RATIONAL_B_SPLINE_CURVE ( ( 0.9346381638529870362, 0.9225778897267418177, 1.000000000000000000, 0.9330127018922187432, 0.9330127018922192983 ) ) 
 REPRESENTATION_ITEM ( '' )  );
#12371=CARTESIAN_POINT ( 'NONE',  ( 235.5999999999999375, -32.02499999999999858, -50.00000000000011369 ) ) ;
#12372=VERTEX_POINT ( 'NONE', #11726 ) ;
#12379=CARTESIAN_POINT ( 'NONE',  ( 229.8435696437499871, -34.71562499938548285, 101.5914258081833879 ) ) ;
#12382=DIRECTION ( 'NONE',  ( 0.000000000000000000, 1.000000000000000000, 0.000000000000000000 ) ) ;
#12390=CARTESIAN_POINT ( 'NONE',  ( 232.5999999999999375, -32.84062499938548285, 103.1828516163667899 ) ) ;
#12391=CARTESIAN_POINT ( 'NONE',  ( 229.8435696437499303, -31.60312499938548214, -50.00000000000011369 ) ) ;
#12395=EDGE_LOOP ( 'NONE', ( #10548, #9574, #2272, #18463, #10264, #13759 ) ) ;
#12397=CARTESIAN_POINT ( 'NONE',  ( 231.7961524227065695, -32.73615380933862440, -53.00000000000012079 ) ) ;
#12398=CARTESIAN_POINT ( 'NONE',  ( 232.5999999999999375, -29.99999999999999645, -50.00000000000011369 ) ) ;
#12400=ORIENTED_EDGE ( 'NONE', *, *, #17619, .F. ) ;
#12407=AXIS2_PLACEMENT_3D ( 'NONE', #13104, #14857, #17899 ) ;
#12411=CARTESIAN_POINT ( 'NONE',  ( 232.5999999999999375, -33.17812499938548143, 103.1828516163667899 ) ) ;
#12414=CARTESIAN_POINT ( 'NONE',  ( 232.5999999999999375, -30.95624999877096428, 96.53589838486223584 ) ) ;
#12415=CARTESIAN_POINT ( 'NONE',  ( 102.9999999999999858, -29.80000000000000071, 150.0000000000000000 ) ) ;
#12421=CARTESIAN_POINT ( 'NONE',  ( 229.5999999999999375, -33.58124999877096428, 98.26794919243111792 ) ) ;
#12426=CARTESIAN_POINT ( 'NONE',  ( 235.5999999999999375, -33.37499999999999289, -50.00000000000011369 ) ) ;
#12437=CARTESIAN_POINT ( 'NONE',  ( 229.5999999999999375, -31.79999999999999361, -50.00000000000011369 ) ) ;
#12440=CARTESIAN_POINT ( 'NONE',  ( 235.3564303562499447, -32.72812499938547859, 99.99999999999998579 ) ) ;
#12442=CARTESIAN_POINT ( 'NONE',  ( 235.3564303562499447, -33.62812499938547717, -50.00000000000011369 ) ) ;
#12455=FACE_OUTER_BOUND ( 'NONE', #11504, .T. ) ;
#12471=CARTESIAN_POINT ( 'NONE',  ( 233.9782151781249411, -34.90312499938547575, 97.61286128772489690 ) ) ;
#12476=CARTESIAN_POINT ( 'NONE',  ( 230.3249173797030096, -31.99999999999999289, 101.5663513044663091 ) ) ;
#12478=CARTESIAN_POINT ( 'NONE',  ( 244.7999999999999545, -29.80000000000002203, 153.0000000000000000 ) ) ;
#12483=CARTESIAN_POINT ( 'NONE',  ( 233.9782151781249411, -31.75312499938547717, 97.61286128772489690 ) ) ;
#12484=CARTESIAN_POINT ( 'NONE',  ( 231.2217848218749339, -31.07812499938548001, -47.61286128772501769 ) ) ;
#12491=LINE ( 'NONE', #11652, #6307 ) ;
#12502=CARTESIAN_POINT ( 'NONE',  ( 229.8435696437499871, -34.60312499938547859, 101.5914258081833879 ) ) ;
#12514=CARTESIAN_POINT ( 'NONE',  ( 232.5999999999999375, -34.75312499938547717, -53.18285161636690361 ) ) ;
#12515=CARTESIAN_POINT ( 'NONE',  ( 234.0999999999999375, -33.84374999877096002, -47.40192378864679768 ) ) ;
#12523=LINE ( 'NONE', #19167, #15995 ) ;
#12528=EDGE_LOOP ( 'NONE', ( #15498, #5589, #10038, #4959 ) ) ;
#12530=CARTESIAN_POINT ( 'NONE',  ( 235.3140393761304949, -32.00000000000000000, -48.72172371342785624 ) ) ;
#12533=CARTESIAN_POINT ( 'NONE',  ( 229.8435696437499587, -32.46562499938548285, 101.5914258081833879 ) ) ;
#12535=CARTESIAN_POINT ( 'NONE',  ( 229.8435696437499303, -32.05312499938548143, -50.00000000000011369 ) ) ;
#12537=EDGE_LOOP ( 'NONE', ( #8768, #13715, #4421, #3856 ) ) ;
#12548=CARTESIAN_POINT ( 'NONE',  ( 233.9782151781249411, -30.74062499938547788, -52.38713871227520968 ) ) ;
#12551=ORIENTED_EDGE ( 'NONE', *, *, #6395, .F. ) ;
#12556=AXIS2_PLACEMENT_3D ( 'NONE', #11330, #8395, #11035 ) ;
#12564=CARTESIAN_POINT ( 'NONE',  ( 229.5999999999999375, -34.01249999999999574, -48.26794919243123161 ) ) ;
#12566=CARTESIAN_POINT ( 'NONE',  ( 232.5999999999999375, -33.96562499938547575, 96.81714838363319586 ) ) ;
#12569=CARTESIAN_POINT ( 'NONE',  ( 231.0999999999999375, -32.77499999999999147, 97.40192378864668399 ) ) ;
#12576=CARTESIAN_POINT ( 'NONE',  ( 230.2961164517930968, -35.00002705695767702, -51.92148140967023551 ) ) ;
#12578=ORIENTED_EDGE ( 'NONE', *, *, #6183, .F. ) ;
#12581=CARTESIAN_POINT ( 'NONE',  ( 233.9782151781249411, -32.35312499938547859, 102.3871387122750889 ) ) ;
#12582=CARTESIAN_POINT ( 'NONE',  ( 232.5999999999999375, -33.74062499938548143, -46.81714838363331666 ) ) ;
#12599=DIRECTION ( 'NONE',  ( -0.000000000000000000, -1.000000000000000000, 3.597944987211154374E-15 ) ) ;
#12600=CARTESIAN_POINT ( 'NONE',  ( 232.5999999999999375, -34.07812499938548001, 103.1828516163667899 ) ) ;
#12603=CARTESIAN_POINT ( 'NONE',  ( 229.5999999999999375, -31.33124999877096073, 98.26794919243111792 ) ) ;
#12604=FACE_OUTER_BOUND ( 'NONE', #7680, .T. ) ;
#12605=EDGE_LOOP ( 'NONE', ( #9895, #16823, #15997, #7164 ) ) ;
#12621=CARTESIAN_POINT ( 'NONE',  ( 229.5999999999999375, -32.15624999877096002, -48.26794919243123161 ) ) ;
#12625=ORIENTED_EDGE ( 'NONE', *, *, #18550, .T. ) ;
#12626=CARTESIAN_POINT ( 'NONE',  ( 234.0999999999999375, -34.64999999999999147, -52.59807621135342970 ) ) ;
#12632=CARTESIAN_POINT ( 'NONE',  ( 229.8435696437499871, -31.45312499938547290, -48.40857419181671162 ) ) ;
#12633=ORIENTED_EDGE ( 'NONE', *, *, #13046, .T. ) ;
#12639=( BOUNDED_CURVE ( )  B_SPLINE_CURVE ( 2, ( #7343, #8711, #16532, #6082, #14861, #13296, #18101, #16624, #1299 ),
 .UNSPECIFIED., .F., .F. ) 
 B_SPLINE_CURVE_WITH_KNOTS ( ( 3, 2, 2, 2, 3 ),
 ( 0.4374999999999999445, 0.4444444444444444198, 0.4583333333333333148, 0.4722222222222222099, 0.4791666666666665186 ),
 .UNSPECIFIED. ) 
 CURVE ( )  GEOMETRIC_REPRESENTATION_ITEM ( )  RATIONAL_B_SPLINE_CURVE ( ( 0.9330127018922192983, 0.9330127018922187432, 1.000000000000000000, 0.8660254037844387076, 1.000000000000000000, 0.8660254037844387076, 1.000000000000000000, 0.9330127018922207416, 0.9330127018922194093 ) ) 
 REPRESENTATION_ITEM ( '' )  );
#12644=CARTESIAN_POINT ( 'NONE',  ( 229.8435696437499871, -32.35312499938547859, -48.40857419181671162 ) ) ;
#12647=ORIENTED_EDGE ( 'NONE', *, *, #18735, .T. ) ;
#12652=VECTOR ( 'NONE', #17548, 1000.000000000000000 ) ;
#12655=DIRECTION ( 'NONE',  ( 0.000000000000000000, 0.000000000000000000, 1.000000000000000000 ) ) ;
#12656=EDGE_LOOP ( 'NONE', ( #16488, #17083, #4135, #17222 ) ) ;
#12658=CARTESIAN_POINT ( 'NONE',  ( 230.5724978686189672, -35.00000000000000711, -52.22004150442379711 ) ) ;
#12660=CARTESIAN_POINT ( 'NONE',  ( 229.8435696437499871, -32.42812499938548143, 98.40857419181659793 ) ) ;
#12669=DIRECTION ( 'NONE',  ( 0.000000000000000000, 1.000000000000000000, 0.000000000000000000 ) ) ;
#12674=CARTESIAN_POINT ( 'NONE',  ( 229.8435696437499871, -32.46562499938548285, 101.5914258081833879 ) ) ;
#12675=CARTESIAN_POINT ( 'NONE',  ( 235.3564303562499447, -33.62812499938547717, -50.00000000000011369 ) ) ;
#12678=CARTESIAN_POINT ( 'NONE',  ( 231.0999999999999375, -32.77499999999999147, -52.59807621135342970 ) ) ;
#12679=ORIENTED_EDGE ( 'NONE', *, *, #7571, .F. ) ;
#12684=EDGE_CURVE ( 'NONE', #7898, #1498, #8560, .T. ) ;
#12687=EDGE_CURVE ( 'NONE', #1971, #5593, #10644, .T. ) ;
#12693=CARTESIAN_POINT ( 'NONE',  ( 231.5800379434388674, -35.00000000000000000, 97.17173842519744653 ) ) ;
#12696=CARTESIAN_POINT ( 'NONE',  ( 235.3564303562499447, -34.90312499938547575, 101.5914258081833879 ) ) ;
#12700=FACE_OUTER_BOUND ( 'NONE', #5772, .T. ) ;
#12701=CARTESIAN_POINT ( 'NONE',  ( 231.0999999999999375, -31.66874999877096641, -47.40192378864679768 ) ) ;
#12702=VERTEX_POINT ( 'NONE', #9270 ) ;
#12703=CARTESIAN_POINT ( 'NONE',  ( 232.5999999999999375, -34.61249999999999716, 97.00000000000000000 ) ) ;
#12710=CARTESIAN_POINT ( 'NONE',  ( 229.5999999999999375, -33.09374999877096002, 99.99999999999998579 ) ) ;
#12712=LINE ( 'NONE', #17406, #5160 ) ;
#12713=EDGE_CURVE ( 'NONE', #17759, #3211, #19308, .T. ) ;
#12716=VECTOR ( 'NONE', #9351, 1000.000000000000000 ) ;
#12718=ADVANCED_FACE ( 'NONE', ( #14846 ), #1472, .F. ) ;
#12721=LINE ( 'NONE', #9791, #13047 ) ;
#12730=CARTESIAN_POINT ( 'NONE',  ( 231.0999999999999375, -34.12499999999999289, -52.59807621135342970 ) ) ;
#12731=CARTESIAN_POINT ( 'NONE',  ( 235.5999999999999943, -33.28124999877096002, -51.73205080756900287 ) ) ;
#12733=VECTOR ( 'NONE', #12382, 1000.000000000000000 ) ;
#12734=CARTESIAN_POINT ( 'NONE',  ( 233.9782151781249411, -33.10312499938547859, 97.61286128772489690 ) ) ;
#12736=EDGE_CURVE ( 'NONE', #9023, #9588, #5952, .T. ) ;
#12737=CARTESIAN_POINT ( 'NONE',  ( 235.3564303562499447, -34.49062499938548143, -51.59142580818350865 ) ) ;
#12738=ORIENTED_EDGE ( 'NONE', *, *, #16994, .T. ) ;
#12743=CARTESIAN_POINT ( 'NONE',  ( 229.5999999999999375, -33.09374999877096002, -50.00000000000011369 ) ) ;
#12744=CARTESIAN_POINT ( 'NONE',  ( 235.3564303562499447, -32.65312499938547575, -48.40857419181671162 ) ) ;
#12750=CARTESIAN_POINT ( 'NONE',  ( 235.3564303562499447, -33.47812499938547148, -51.59142580818350865 ) ) ;
#12754=CARTESIAN_POINT ( 'NONE',  ( 235.5999999999999943, -34.25624999877096144, -48.26794919243124582 ) ) ;
#12762=DIRECTION ( 'NONE',  ( -0.000000000000000000, 1.000000000000000000, 0.000000000000000000 ) ) ;
#12767=DIRECTION ( 'NONE',  ( 0.000000000000000000, 0.000000000000000000, 1.000000000000000000 ) ) ;
#12768=CARTESIAN_POINT ( 'NONE',  ( 230.4319669496466645, -32.00000000000000000, 101.7116913729795300 ) ) ;
#12771=CARTESIAN_POINT ( 'NONE',  ( 233.0909187468005825, -32.00000000000000000, 97.16185054498762952 ) ) ;
#12778=CARTESIAN_POINT ( 'NONE',  ( 235.1663847376154592, -35.00000000000000000, -48.97827398863936565 ) ) ;
#12779=CARTESIAN_POINT ( 'NONE',  ( 232.5999999999999375, -33.06562499938547717, -53.18285161636690361 ) ) ;
#12781=CARTESIAN_POINT ( 'NONE',  ( 229.5999999999999375, -32.69999999999999574, -50.00000000000011369 ) ) ;
#12789=FACE_OUTER_BOUND ( 'NONE', #14166, .T. ) ;
#12795=CARTESIAN_POINT ( 'NONE',  ( 230.7036604445367232, -32.00000000000000711, 102.0295751981966390 ) ) ;
#12796=CARTESIAN_POINT ( 'NONE',  ( 235.5999999999999943, -30.18749999999999289, 98.26794919243110371 ) ) ;
#12800=CARTESIAN_POINT ( 'NONE',  ( 235.5999999999999943, -30.65624999877095647, 101.7320508075688537 ) ) ;
#12801=CARTESIAN_POINT ( 'NONE',  ( 229.5999999999999375, -32.15624999877096002, -48.26794919243123161 ) ) ;
#12813=EDGE_CURVE ( 'NONE', #2968, #5414, #1358, .T. ) ;
#12826=EDGE_CURVE ( 'NONE', #6930, #18607, #13418, .T. ) ;
#12828=CARTESIAN_POINT ( 'NONE',  ( 232.5999999999999943, -34.41562499938547859, 96.81714838363319586 ) ) ;
#12831=CARTESIAN_POINT ( 'NONE',  ( 229.8435696437499871, -31.52812499938547575, -51.59142580818350865 ) ) ;
#12836=CARTESIAN_POINT ( 'NONE',  ( 232.5999999999999375, -29.99999999999999645, -53.00000000000012079 ) ) ;
#12838=DIRECTION ( 'NONE',  ( 0.000000000000000000, 0.000000000000000000, -1.000000000000000000 ) ) ;
#12844=CARTESIAN_POINT ( 'NONE',  ( 233.9782151781249411, -32.54062499938547859, -52.38713871227520968 ) ) ;
#12848=DIRECTION ( 'NONE',  ( -1.000000000000000000, 0.000000000000000000, 0.000000000000000000 ) ) ;
#12853=CARTESIAN_POINT ( 'NONE',  ( 105.1999999999999886, -29.80000000000001492, -97.80000000000002558 ) ) ;
#12855=AXIS2_PLACEMENT_3D ( 'NONE', #4256, #13233, #8741 ) ;
#12856=CIRCLE ( 'NONE', #19107, 3.000000000000002665 ) ;
#12860=CARTESIAN_POINT ( 'NONE',  ( 105.1999999999999744, -29.80000000000000071, -100.0000000000000000 ) ) ;
#12861=EDGE_CURVE ( 'NONE', #2004, #9023, #15021, .T. ) ;
#12866=CARTESIAN_POINT ( 'NONE',  ( 232.3828836072648869, -32.00000000000001421, 97.16008101253267171 ) ) ;
#12869=ORIENTED_EDGE ( 'NONE', *, *, #7677, .F. ) ;
#12871=CARTESIAN_POINT ( 'NONE',  ( 233.9782151781249411, -33.70312499938548001, 102.3871387122750889 ) ) ;
#12872=CARTESIAN_POINT ( 'NONE',  ( 233.9782151781249411, -33.55312499938548143, -52.38713871227520968 ) ) ;
#12875=ORIENTED_EDGE ( 'NONE', *, *, #8279, .T. ) ;
#12889=CARTESIAN_POINT ( 'NONE',  ( 235.2218879900010791, -34.99999999999999289, 100.8506536761482124 ) ) ;
#12891=CARTESIAN_POINT ( 'NONE',  ( 234.0999999999999375, -31.19999999999999574, 102.5980762113533018 ) ) ;
#12892=VERTEX_POINT ( 'NONE', #13162 ) ;
#12895=CARTESIAN_POINT ( 'NONE',  ( 229.5999999999999375, -32.64374999877096428, 99.99999999999998579 ) ) ;
#12913=CARTESIAN_POINT ( 'NONE',  ( 234.7581833435468184, -31.99999999999999289, -52.02304716543538632 ) ) ;
#12919=CARTESIAN_POINT ( 'NONE',  ( 232.5999999999999375, -34.83749999999999147, -46.53589838486234953 ) ) ;
#12922=CARTESIAN_POINT ( 'NONE',  ( 233.9782151781249411, -34.00312499938547717, 97.61286128772489690 ) ) ;
#12924=CARTESIAN_POINT ( 'NONE',  ( 235.3564303562499447, -30.40312499938547575, -48.40857419181671162 ) ) ;
#12936=CARTESIAN_POINT ( 'NONE',  ( 231.2217848218749339, -33.66562499938547859, -47.61286128772501769 ) ) ;
#12940=VERTEX_POINT ( 'NONE', #15208 ) ;
#12949=CARTESIAN_POINT ( 'NONE',  ( 232.5999999999999943, -32.95312499938548001, 96.81714838363319586 ) ) ;
#12950=LINE ( 'NONE', #18922, #17656 ) ;
#12952=EDGE_CURVE ( 'NONE', #11625, #6661, #932, .T. ) ;
#12959=CARTESIAN_POINT ( 'NONE',  ( 233.5509609210264728, -32.00000000000000000, 97.25957015487007595 ) ) ;
#12960=CARTESIAN_POINT ( 'NONE',  ( 231.0999999999999375, -34.96874999877096002, -52.59807621135342970 ) ) ;
#12966=DIRECTION ( 'NONE',  ( 0.000000000000000000, 0.000000000000000000, 1.000000000000000000 ) ) ;
#12967=CARTESIAN_POINT ( 'NONE',  ( 229.8435696437499871, -32.46562499938548285, -48.40857419181671162 ) ) ;
#12970=ORIENTED_EDGE ( 'NONE', *, *, #7452, .T. ) ;
#12971=EDGE_CURVE ( 'NONE', #15137, #17445, #3366, .T. ) ;
#12979=CARTESIAN_POINT ( 'NONE',  ( 232.5999999999999375, -30.36562499938548498, 96.81714838363319586 ) ) ;
#12983=CARTESIAN_POINT ( 'NONE',  ( 234.1913891058629815, -35.00000000000002132, 102.2789443502791045 ) ) ;
#12986=CARTESIAN_POINT ( 'NONE',  ( 235.5999999999999375, -30.22499999999999432, 99.99999999999998579 ) ) ;
#12990=CARTESIAN_POINT ( 'NONE',  ( 229.5999999999999375, -32.68124999877096570, 98.26794919243111792 ) ) ;
#12991=CARTESIAN_POINT ( 'NONE',  ( 231.0999999999999375, -30.91874999877096286, -52.59807621135342970 ) ) ;
#12993=DIRECTION ( 'NONE',  ( -0.000000000000000000, -0.000000000000000000, 1.000000000000000000 ) ) ;
#12997=CARTESIAN_POINT ( 'NONE',  ( 244.7999999999999545, -29.80000000000001492, -97.80000000000002558 ) ) ;
#12998=( BOUNDED_CURVE ( )  B_SPLINE_CURVE ( 2, ( #2101, #7771, #6221, #15288, #6407, #267, #18330, #9422, #5042 ),
 .UNSPECIFIED., .F., .F. ) 
 B_SPLINE_CURVE_WITH_KNOTS ( ( 3, 2, 2, 2, 3 ),
 ( 0.5208333333333332593, 0.5277777777777777901, 0.5416666666666666297, 0.5555555555555555802, 0.5625000000000002220 ),
 .UNSPECIFIED. ) 
 CURVE ( )  GEOMETRIC_REPRESENTATION_ITEM ( )  RATIONAL_B_SPLINE_CURVE ( ( 0.9330127018922192983, 0.9330127018922187432, 1.000000000000000000, 0.8660254037844387076, 1.000000000000000000, 0.8660254037844387076, 1.000000000000000000, 0.9330127018922171889, 0.9330127018922194093 ) ) 
 REPRESENTATION_ITEM ( '' )  );
#13008=CARTESIAN_POINT ( 'NONE',  ( 232.3828836072649722, -31.99999999999998579, -52.83991898746749172 ) ) ;
#13009=CARTESIAN_POINT ( 'NONE',  ( 244.7999999999999545, -29.80000000000001492, -97.80000000000002558 ) ) ;
#13014=VECTOR ( 'NONE', #8261, 1000.000000000000000 ) ;
#13016=CARTESIAN_POINT ( 'NONE',  ( 232.5999999999999375, -29.99999999999999645, -47.00000000000010658 ) ) ;
#13018=CARTESIAN_POINT ( 'NONE',  ( 231.2217848218749339, -33.92812499938548143, 97.61286128772489690 ) ) ;
#13021=CARTESIAN_POINT ( 'NONE',  ( 231.2217848218749339, -31.11562499938547788, -52.38713871227520968 ) ) ;
#13027=CARTESIAN_POINT ( 'NONE',  ( 231.0999999999999375, -33.16874999877095576, -52.59807621135342970 ) ) ;
#13028=CARTESIAN_POINT ( 'NONE',  ( 235.3564303562499447, -31.30312499938547788, 101.5914258081833879 ) ) ;
#13034=CARTESIAN_POINT ( 'NONE',  ( 229.8435696437499303, -31.94062499938547717, -50.00000000000011369 ) ) ;
#13045=AXIS2_PLACEMENT_3D ( 'NONE', #13651, #1924, #10628 ) ;
#13046=EDGE_CURVE ( 'NONE', #8256, #18958, #7939, .T. ) ;
#13047=VECTOR ( 'NONE', #15656, 1000.000000000000000 ) ;
#13048=CARTESIAN_POINT ( 'NONE',  ( 229.8435696437499303, -33.29062499938547148, 99.99999999999998579 ) ) ;
#13051=EDGE_CURVE ( 'NONE', #18958, #10687, #10825, .T. ) ;
#13057=CARTESIAN_POINT ( 'NONE',  ( 232.5999999999999375, -29.99999999999999645, 96.99999999999998579 ) ) ;
#13058=CARTESIAN_POINT ( 'NONE',  ( 244.7999999999999545, -32.00000000000000000, 150.0000000000000000 ) ) ;
#13061=CARTESIAN_POINT ( 'NONE',  ( 232.5999999999999375, -34.16249999999999432, 96.99999999999997158 ) ) ;
#13064=CARTESIAN_POINT ( 'NONE',  ( 232.5999999999999375, -33.96562499938547575, 96.81714838363319586 ) ) ;
#13079=CARTESIAN_POINT ( 'NONE',  ( 229.5999999999999375, -32.24999999999999289, -50.00000000000011369 ) ) ;
#13081=CARTESIAN_POINT ( 'NONE',  ( 235.5999999999999375, -32.02499999999999858, 99.99999999999998579 ) ) ;
#13082=ORIENTED_EDGE ( 'NONE', *, *, #2560, .T. ) ;
#13085=CARTESIAN_POINT ( 'NONE',  ( 229.5999999999999375, -31.70624999877096073, 101.7320508075688679 ) ) ;
#13086=CARTESIAN_POINT ( 'NONE',  ( 231.0999999999999375, -30.76874999877096428, -47.40192378864679768 ) ) ;
#13092=CARTESIAN_POINT ( 'NONE',  ( 244.7999999999999545, -32.00000000000001421, -103.0000000000000142 ) ) ;
#13104=CARTESIAN_POINT ( 'NONE',  ( 244.7999999999999545, -29.80000000000000426, -100.0000000000000000 ) ) ;
#13109=CARTESIAN_POINT ( 'NONE',  ( 232.5999999999999943, -34.19062499938547717, 103.1828516163667899 ) ) ;
#13112=CARTESIAN_POINT ( 'NONE',  ( 233.9782151781249411, -32.99062499938548143, -52.38713871227520968 ) ) ;
#13116=DIRECTION ( 'NONE',  ( -0.000000000000000000, -1.000000000000000000, -0.000000000000000000 ) ) ;
#13119=CARTESIAN_POINT ( 'NONE',  ( 231.2217848218749339, -31.56562499938547717, 97.61286128772489690 ) ) ;
#13125=CARTESIAN_POINT ( 'NONE',  ( 229.5999999999999375, -31.34999999999999432, -50.00000000000011369 ) ) ;
#13129=CYLINDRICAL_SURFACE ( 'NONE', #727, 3.000000000000009770 ) ;
#13130=CARTESIAN_POINT ( 'NONE',  ( 229.8435696437499871, -31.64062499938547290, -51.59142580818350865 ) ) ;
#13132=ORIENTED_EDGE ( 'NONE', *, *, #8502, .F. ) ;
#13134=CARTESIAN_POINT ( 'NONE',  ( 231.2217848218749339, -33.36562499938548143, 97.61286128772489690 ) ) ;
#13138=CARTESIAN_POINT ( 'NONE',  ( 234.1936318287815197, -32.00000000000000711, -47.53037344451306012 ) ) ;
#13142=DIRECTION ( 'NONE',  ( -0.000000000000000000, -1.000000000000000000, -0.000000000000000000 ) ) ;
#13143=CARTESIAN_POINT ( 'NONE',  ( 105.2000000000000739, -29.80000000000002203, 150.0000000000000000 ) ) ;
#13146=ORIENTED_EDGE ( 'NONE', *, *, #5667, .T. ) ;
#13148=CARTESIAN_POINT ( 'NONE',  ( 233.9782151781249411, -34.15312499938547575, 102.3871387122750889 ) ) ;
#13150=EDGE_CURVE ( 'NONE', #11929, #7231, #9910, .T. ) ;
#13154=CARTESIAN_POINT ( 'NONE',  ( 234.0999999999999375, -34.14374999877096428, 97.40192378864668399 ) ) ;
#13155=LINE ( 'NONE', #4274, #1503 ) ;
#13162=CARTESIAN_POINT ( 'NONE',  ( 235.4117376914898045, -31.99999999999999289, 98.95399275611721635 ) ) ;
#13164=CARTESIAN_POINT ( 'NONE',  ( 229.8435696437499871, -32.46562499938548285, 101.5914258081833879 ) ) ;
#13172=CARTESIAN_POINT ( 'NONE',  ( 231.0429922824658320, -35.00000000000000711, 97.42750194505826755 ) ) ;
#13174=CARTESIAN_POINT ( 'NONE',  ( 234.0999999999999375, -31.04999999999999361, 97.40192378864668399 ) ) ;
#13177=CARTESIAN_POINT ( 'NONE',  ( 235.5999999999999943, -32.90624999877096002, 101.7320508075688537 ) ) ;
#13178=CARTESIAN_POINT ( 'NONE',  ( 235.5999999999999943, -34.18124999877096570, -51.73205080756900287 ) ) ;
#13187=FACE_OUTER_BOUND ( 'NONE', #10045, .T. ) ;
#13203=CARTESIAN_POINT ( 'NONE',  ( 105.1999999999999886, -4.999999999999984013, -100.0000000000000995 ) ) ;
#13204=CARTESIAN_POINT ( 'NONE',  ( 231.2217848218749339, -33.77812499938547575, 102.3871387122750889 ) ) ;
#13207=CARTESIAN_POINT ( 'NONE',  ( 232.5999999999999375, -33.85312499938547859, -53.18285161636690361 ) ) ;
#13208=ORIENTED_EDGE ( 'NONE', *, *, #7571, .T. ) ;
#13209=VERTEX_POINT ( 'NONE', #16255 ) ;
#13210=FACE_OUTER_BOUND ( 'NONE', #12605, .T. ) ;
#13211=EDGE_CURVE ( 'NONE', #9169, #7775, #11754, .T. ) ;
#13216=CARTESIAN_POINT ( 'NONE',  ( 235.3564303562499447, -30.77812499938547575, 98.40857419181659793 ) ) ;
#13217=CARTESIAN_POINT ( 'NONE',  ( 229.8435696437499587, -33.25312499938547717, -48.40857419181671162 ) ) ;
#13220=( BOUNDED_CURVE ( )  B_SPLINE_CURVE ( 2, ( #15214, #4777, #1830, #6620, #16970, #12287, #12569, #3683, #13835 ),
 .UNSPECIFIED., .F., .F. ) 
 B_SPLINE_CURVE_WITH_KNOTS ( ( 3, 2, 2, 2, 3 ),
 ( 0.4791666666666665186, 0.4861111111111111049, 0.5000000000000000000, 0.5138888888888888395, 0.5208333333333333703 ),
 .UNSPECIFIED. ) 
 CURVE ( )  GEOMETRIC_REPRESENTATION_ITEM ( )  RATIONAL_B_SPLINE_CURVE ( ( 0.9330127018922194093, 0.9330127018922180770, 1.000000000000000000, 0.8660254037844387076, 1.000000000000000000, 0.8660254037844387076, 1.000000000000000000, 0.9330127018922187432, 0.9330127018922192983 ) ) 
 REPRESENTATION_ITEM ( '' )  );
#13222=CARTESIAN_POINT ( 'NONE',  ( 229.5999999999999375, -30.93749999999999289, -51.73205080756898866 ) ) ;
#13225=EDGE_CURVE ( 'NONE', #19255, #16126, #3944, .T. ) ;
#13228=CARTESIAN_POINT ( 'NONE',  ( 232.5999999999999375, -30.59062499938547930, -46.81714838363331666 ) ) ;
#13233=DIRECTION ( 'NONE',  ( -0.000000000000000000, -1.000000000000000000, -0.000000000000000000 ) ) ;
#13237=CARTESIAN_POINT ( 'NONE',  ( 232.1383900424028752, -31.99999999999999289, -47.18959324165065539 ) ) ;
#13242=ADVANCED_FACE ( 'NONE', ( #16547 ), #9200, .T. ) ;
#13243=CARTESIAN_POINT ( 'NONE',  ( 229.5999999999999375, -33.14999999999999147, -50.00000000000011369 ) ) ;
#13246=ORIENTED_EDGE ( 'NONE', *, *, #5667, .F. ) ;
#13250=CARTESIAN_POINT ( 'NONE',  ( 232.5999999999999375, -34.83749999999999147, -47.00000000000011369 ) ) ;
#13261=CARTESIAN_POINT ( 'NONE',  ( 229.8435696437499303, -32.05312499938548143, 99.99999999999998579 ) ) ;
#13269=CARTESIAN_POINT ( 'NONE',  ( 232.5999999999999375, -32.81249999999999289, 96.53589838486223584 ) ) ;
#13272=CARTESIAN_POINT ( 'NONE',  ( 235.5999999999999943, -34.70624999877096428, 101.7320508075688537 ) ) ;
#13273=CARTESIAN_POINT ( 'NONE',  ( 235.5999999999999943, -33.80624999877096570, -48.26794919243124582 ) ) ;
#13281=ORIENTED_EDGE ( 'NONE', *, *, #8045, .F. ) ;
#13288=DIRECTION ( 'NONE',  ( -0.000000000000000000, -1.000000000000000000, -0.000000000000000000 ) ) ;
#13296=CARTESIAN_POINT ( 'NONE',  ( 235.5999999999999943, -32.51249999999999574, -48.26794919243124582 ) ) ;
#13298=LINE ( 'NONE', #5788, #240 ) ;
#13300=CARTESIAN_POINT ( 'NONE',  ( 244.7999999999999545, -32.00000000000000000, 150.0000000000000000 ) ) ;
#13304=CARTESIAN_POINT ( 'NONE',  ( 235.3564303562499447, -33.96562499938547575, -50.00000000000011369 ) ) ;
#13315=CARTESIAN_POINT ( 'NONE',  ( 229.8435696437499871, -31.90312499938547575, 101.5914258081833879 ) ) ;
#13319=EDGE_CURVE ( 'NONE', #18970, #12892, #15223, .T. ) ;
#13320=CARTESIAN_POINT ( 'NONE',  ( 233.9782151781249411, -34.79062499938547859, -52.38713871227520968 ) ) ;
#13338=FACE_OUTER_BOUND ( 'NONE', #9754, .T. ) ;
#13341=CARTESIAN_POINT ( 'NONE',  ( 233.4038475772933623, -32.11740381056766580, 103.0000000000000000 ) ) ;
#13351=DIRECTION ( 'NONE',  ( -0.000000000000000000, 1.000000000000000000, -0.000000000000000000 ) ) ;
#13352=CARTESIAN_POINT ( 'NONE',  ( 229.8435696437499871, -34.34062499938547575, -51.59142580818350865 ) ) ;
#13356=DIRECTION ( 'NONE',  ( -0.000000000000000000, -1.000000000000000000, -0.000000000000000000 ) ) ;
#13359=DIRECTION ( 'NONE',  ( 0.000000000000000000, 0.000000000000000000, -1.000000000000000000 ) ) ;
#13365=CARTESIAN_POINT ( 'NONE',  ( 231.2217848218749339, -32.57812499938548001, 97.61286128772489690 ) ) ;
#13371=CARTESIAN_POINT ( 'NONE',  ( 235.5999999999999375, -33.31874999877096144, 99.99999999999998579 ) ) ;
#13373=CARTESIAN_POINT ( 'NONE',  ( 235.5999999999999943, -32.51249999999998863, 101.7320508075688537 ) ) ;
#13376=CARTESIAN_POINT ( 'NONE',  ( 235.3564303562499447, -30.44062499938548072, 98.40857419181659793 ) ) ;
#13377=CARTESIAN_POINT ( 'NONE',  ( 235.5999999999999375, -33.76874999877096428, -50.00000000000011369 ) ) ;
#13380=ORIENTED_EDGE ( 'NONE', *, *, #11986, .T. ) ;
#13381=DIRECTION ( 'NONE',  ( -0.000000000000000000, 0.000000000000000000, -1.000000000000000000 ) ) ;
#13384=ORIENTED_EDGE ( 'NONE', *, *, #3904, .T. ) ;
#13391=CARTESIAN_POINT ( 'NONE',  ( 229.5999999999999375, -33.56249999999999289, 101.7320508075688821 ) ) ;
#13395=CARTESIAN_POINT ( 'NONE',  ( 232.5999999999999375, -31.15312499938547930, 96.81714838363319586 ) ) ;
#13399=CARTESIAN_POINT ( 'NONE',  ( 233.4038475772932770, -33.41115380933862156, -47.00000000000009948 ) ) ;
#13404=CARTESIAN_POINT ( 'NONE',  ( 231.2217848218749339, -31.86562499938547788, -47.61286128772501769 ) ) ;
#13414=CARTESIAN_POINT ( 'NONE',  ( 232.5999999999999375, -33.40312499938547575, 96.81714838363319586 ) ) ;
#13415=CARTESIAN_POINT ( 'NONE',  ( 233.9782151781249411, -33.89062499938548001, -52.38713871227520968 ) ) ;
#13418=( BOUNDED_CURVE ( )  B_SPLINE_CURVE ( 2, ( #7400, #14925, #17959, #17863, #6044, #5945, #7209, #3096, #12087 ),
 .UNSPECIFIED., .F., .F. ) 
 B_SPLINE_CURVE_WITH_KNOTS ( ( 3, 2, 2, 2, 3 ),
 ( 0.5625000000000001110, 0.5694444444444444198, 0.5833333333333333703, 0.5972222222222222099, 0.6041666666666667407 ),
 .UNSPECIFIED. ) 
 CURVE ( )  GEOMETRIC_REPRESENTATION_ITEM ( )  RATIONAL_B_SPLINE_CURVE ( ( 0.9330127018922194093, 0.9330127018922204085, 1.000000000000000000, 0.8660254037844387076, 1.000000000000000000, 0.8660254037844387076, 1.000000000000000000, 0.9330127018922187432, 0.9330127018922192983 ) ) 
 REPRESENTATION_ITEM ( '' )  );
#13421=CARTESIAN_POINT ( 'NONE',  ( 232.5999999999999375, -34.75312499938547717, -53.18285161636690361 ) ) ;
#13423=CARTESIAN_POINT ( 'NONE',  ( 105.1999999999999886, -4.999999999999984013, -100.0000000000000995 ) ) ;
#13426=CARTESIAN_POINT ( 'NONE',  ( 232.5999999999999375, -29.99999999999999645, 99.99999999999998579 ) ) ;
#13431=CARTESIAN_POINT ( 'NONE',  ( 231.2217848218749339, -34.71562499938547575, 97.61286128772489690 ) ) ;
#13442=ORIENTED_EDGE ( 'NONE', *, *, #17045, .F. ) ;
#13444=DIRECTION ( 'NONE',  ( -0.000000000000000000, -1.000000000000000000, -0.000000000000000000 ) ) ;
#13445=CARTESIAN_POINT ( 'NONE',  ( 232.5999999999999375, -34.41562499938547859, -53.18285161636690361 ) ) ;
#13456=DIRECTION ( 'NONE',  ( -0.000000000000000000, -1.000000000000000000, -0.000000000000000000 ) ) ;
#13457=CARTESIAN_POINT ( 'NONE',  ( 232.5999999999999375, -31.49062499938547788, 103.1828516163667899 ) ) ;
#13460=CARTESIAN_POINT ( 'NONE',  ( 232.5999999999999375, -33.65624999877096002, 97.00000000000000000 ) ) ;
#13465=CARTESIAN_POINT ( 'NONE',  ( 235.5999999999999943, -32.88749999999998863, 98.26794919243110371 ) ) ;
#13467=CARTESIAN_POINT ( 'NONE',  ( 233.9782151781249411, -34.15312499938547575, -47.61286128772501769 ) ) ;
#13468=CARTESIAN_POINT ( 'NONE',  ( 235.3564303562499447, -30.47812499938547859, 99.99999999999998579 ) ) ;
#13469=CARTESIAN_POINT ( 'NONE',  ( 234.0999999999999375, -32.94374999877096144, -47.40192378864679768 ) ) ;
#13471=EDGE_CURVE ( 'NONE', #17889, #927, #12721, .T. ) ;
#13479=AXIS2_PLACEMENT_3D ( 'NONE', #18656, #4182, #11602 ) ;
#13498=CARTESIAN_POINT ( 'NONE',  ( 235.3564303562499447, -32.12812499938547717, -51.59142580818350865 ) ) ;
#13500=ORIENTED_EDGE ( 'NONE', *, *, #8076, .T. ) ;
#13507=CARTESIAN_POINT ( 'NONE',  ( 229.8435696437499871, -34.67812499938547433, 98.40857419181659793 ) ) ;
#13512=ORIENTED_EDGE ( 'NONE', *, *, #11727, .F. ) ;
#13513=CARTESIAN_POINT ( 'NONE',  ( 231.0999999999999375, -30.37499999999999645, -47.40192378864679768 ) ) ;
#13516=CARTESIAN_POINT ( 'NONE',  ( 249.9999999999999716, -5.000000000000004441, 150.0000000000000000 ) ) ;
#13522=CARTESIAN_POINT ( 'NONE',  ( 229.8435696437499587, -34.60312499938547859, 101.5914258081833879 ) ) ;
#13527=CARTESIAN_POINT ( 'NONE',  ( 231.7960411235079050, -35.00000000000002132, 102.6365808225362883 ) ) ;
#13530=CARTESIAN_POINT ( 'NONE',  ( 105.1999999999999744, -31.99999999999999289, 150.0000000000000000 ) ) ;
#13548=CARTESIAN_POINT ( 'NONE',  ( 233.9782151781249411, -31.75312499938547717, 97.61286128772489690 ) ) ;
#13555=CARTESIAN_POINT ( 'NONE',  ( 232.5999999999999375, -34.38749999999999574, 103.4641016151377499 ) ) ;
#13557=CARTESIAN_POINT ( 'NONE',  ( 235.3564303562499447, -34.49062499938548143, -51.59142580818350154 ) ) ;
#13559=EDGE_CURVE ( 'NONE', #12219, #3413, #10864, .T. ) ;
#13560=CARTESIAN_POINT ( 'NONE',  ( 229.8435696437499871, -30.29062499938548214, 98.40857419181659793 ) ) ;
#13561=CARTESIAN_POINT ( 'NONE',  ( 234.0999999999999375, -33.84374999877096002, -47.40192378864679768 ) ) ;
#13566=CARTESIAN_POINT ( 'NONE',  ( 229.5999999999999375, -34.91249999999999432, 101.7320508075688821 ) ) ;
#13567=CARTESIAN_POINT ( 'NONE',  ( 232.5999999999999375, -29.99999999999999645, -47.00000000000010658 ) ) ;
#13568=VERTEX_POINT ( 'NONE', #2174 ) ;
#13576=CARTESIAN_POINT ( 'NONE',  ( 231.7961524227065695, -33.69240381056765443, 96.99999999999998579 ) ) ;
#13581=CARTESIAN_POINT ( 'NONE',  ( 235.3564303562499447, -32.12812499938547717, 98.40857419181659793 ) ) ;
#13585=CARTESIAN_POINT ( 'NONE',  ( 232.5999999999999375, -33.71249999999999147, 96.99999999999998579 ) ) ;
#13586=DIRECTION ( 'NONE',  ( -0.000000000000000000, -1.000000000000000000, -0.000000000000000000 ) ) ;
#13587=DIRECTION ( 'NONE',  ( -0.000000000000000000, -1.000000000000000000, -0.000000000000000000 ) ) ;
#13589=CARTESIAN_POINT ( 'NONE',  ( 229.8435696437499871, -35.05312499938547433, -48.40857419181671162 ) ) ;
#13591=ORIENTED_EDGE ( 'NONE', *, *, #3143, .F. ) ;
#13597=CARTESIAN_POINT ( 'NONE',  ( 235.3564303562499447, -33.06562499938547717, 99.99999999999998579 ) ) ;
#13599=CARTESIAN_POINT ( 'NONE',  ( 232.5999999999999943, -34.75312499938547717, -53.18285161636690361 ) ) ;
#13603=CARTESIAN_POINT ( 'NONE',  ( 235.5999999999999943, -33.33749999999999147, -51.73205080756900287 ) ) ;
#13609=CARTESIAN_POINT ( 'NONE',  ( 229.8435696437499871, -32.91562499938547859, -48.40857419181671162 ) ) ;
#13611=ORIENTED_EDGE ( 'NONE', *, *, #3262, .T. ) ;
#13614=DIRECTION ( 'NONE',  ( -0.000000000000000000, -1.000000000000000000, -0.000000000000000000 ) ) ;
#13615=CARTESIAN_POINT ( 'NONE',  ( 230.5523683116323355, -32.00000000000000000, 101.8452947671440540 ) ) ;
#13617=CARTESIAN_POINT ( 'NONE',  ( 232.5999999999999375, -34.86562499938548143, -53.18285161636690361 ) ) ;
#13621=CARTESIAN_POINT ( 'NONE',  ( 229.9986727058461611, -34.99999999999999289, 101.2112556744905874 ) ) ;
#13624=CARTESIAN_POINT ( 'NONE',  ( 235.3564303562499447, -31.22812499938548214, -51.59142580818350865 ) ) ;
#13629=CARTESIAN_POINT ( 'NONE',  ( 105.1999999999999744, -31.99999999999999289, 153.0000000000000000 ) ) ;
#13630=EDGE_CURVE ( 'NONE', #13743, #18412, #71, .T. ) ;
#13638=( GEOMETRIC_REPRESENTATION_CONTEXT ( 3 ) GLOBAL_UNCERTAINTY_ASSIGNED_CONTEXT ( ( #5114 ) ) GLOBAL_UNIT_ASSIGNED_CONTEXT ( ( #17999, #12026, #14960 ) ) REPRESENTATION_CONTEXT ( 'NONE', 'WORKASPACE' ) );
#13644=CARTESIAN_POINT ( 'NONE',  ( 229.8435696437499871, -33.44062499938547717, 98.40857419181659793 ) ) ;
#13651=CARTESIAN_POINT ( 'NONE',  ( 0.000000000000000000, 0.000000000000000000, 153.0000000000000000 ) ) ;
#13655=CARTESIAN_POINT ( 'NONE',  ( 231.0999999999999375, -33.97500000000000142, 102.5980762113533018 ) ) ;
#13657=ORIENTED_EDGE ( 'NONE', *, *, #14228, .T. ) ;
#13658=CARTESIAN_POINT ( 'NONE',  ( 231.2217848218749339, -32.57812499938548001, -52.38713871227520968 ) ) ;
#13660=CARTESIAN_POINT ( 'NONE',  ( 229.8435696437499303, -30.70312499938548001, 99.99999999999998579 ) ) ;
#13662=CARTESIAN_POINT ( 'NONE',  ( 229.8435696437499871, -30.66562499938547859, -48.40857419181671162 ) ) ;
#13663=EDGE_CURVE ( 'NONE', #6967, #5568, #7149, .T. ) ;
#13669=CARTESIAN_POINT ( 'NONE',  ( 230.2961164517930968, -35.00002705695778360, 98.07851859032987818 ) ) ;
#13682=CARTESIAN_POINT ( 'NONE',  ( 229.8435696437499303, -32.39062499938548001, 99.99999999999998579 ) ) ;
#13685=CARTESIAN_POINT ( 'NONE',  ( 105.1999999999999744, -29.80000000000000071, 150.0000000000000000 ) ) ;
#13690=CARTESIAN_POINT ( 'NONE',  ( 231.7961524227065695, -34.53615380933862866, 96.99999999999998579 ) ) ;
#13691=CARTESIAN_POINT ( 'NONE',  ( 229.6880761451917579, -35.00000000000001421, -50.39325454734051846 ) ) ;
#13703=CARTESIAN_POINT ( 'NONE',  ( 231.2217848218749339, -34.26562499938548001, 97.61286128772489690 ) ) ;
#13707=ORIENTED_EDGE ( 'NONE', *, *, #18906, .T. ) ;
#13708=CARTESIAN_POINT ( 'NONE',  ( 235.5999999999999943, -32.96249999999999858, -48.26794919243124582 ) ) ;
#13713=CARTESIAN_POINT ( 'NONE',  ( 229.8435696437499871, -32.09062499938548285, -51.59142580818350865 ) ) ;
#13715=ORIENTED_EDGE ( 'NONE', *, *, #14490, .F. ) ;
#13717=CARTESIAN_POINT ( 'NONE',  ( 235.3564303562499447, -34.00312499938547717, 101.5914258081833879 ) ) ;
#13721=CARTESIAN_POINT ( 'NONE',  ( 230.4006479041920272, -35.00000000000000000, 101.7928000422452897 ) ) ;
#13724=CARTESIAN_POINT ( 'NONE',  ( 233.9782151781249411, -30.29062499938547859, -52.38713871227520968 ) ) ;
#13730=EDGE_CURVE ( 'NONE', #14449, #10754, #5987, .T. ) ;
#13731=CARTESIAN_POINT ( 'NONE',  ( 234.0999999999999375, -34.19999999999999574, 97.40192378864668399 ) ) ;
#13741=CARTESIAN_POINT ( 'NONE',  ( 235.3564303562499447, -34.11562499938548143, 101.5914258081833879 ) ) ;
#13743=VERTEX_POINT ( 'NONE', #14656 ) ;
#13747=LINE ( 'NONE', #385, #5265 ) ;
#13753=CARTESIAN_POINT ( 'NONE',  ( 231.2217848218749339, -32.87812499938547717, -47.61286128772501769 ) ) ;
#13755=CARTESIAN_POINT ( 'NONE',  ( 231.2217848218749339, -32.87812499938547717, 102.3871387122750889 ) ) ;
#13756=CARTESIAN_POINT ( 'NONE',  ( 231.2217848218749339, -30.32812499938548001, -52.38713871227520968 ) ) ;
#13758=VERTEX_POINT ( 'NONE', #9249 ) ;
#13759=ORIENTED_EDGE ( 'NONE', *, *, #18906, .F. ) ;
#13763=ORIENTED_EDGE ( 'NONE', *, *, #14490, .T. ) ;
#13764=ADVANCED_FACE ( 'NONE', ( #6239 ), #14035, .T. ) ;
#13775=CARTESIAN_POINT ( 'NONE',  ( 229.8435696437499871, -35.05312499938547433, 101.5914258081833879 ) ) ;
#13777=CARTESIAN_POINT ( 'NONE',  ( 232.5999999999999375, -32.72812499938547859, 103.1828516163667899 ) ) ;
#13780=CARTESIAN_POINT ( 'NONE',  ( 99.99999999999997158, -31.99999999999999289, -100.0000000000000000 ) ) ;
#13783=FACE_OUTER_BOUND ( 'NONE', #6449, .T. ) ;
#13784=CARTESIAN_POINT ( 'NONE',  ( 230.2491162085310066, -35.00000000000002132, -48.39201219457986980 ) ) ;
#13793=CARTESIAN_POINT ( 'NONE',  ( 235.3564303562499447, -33.96562499938547575, 99.99999999999998579 ) ) ;
#13798=ORIENTED_EDGE ( 'NONE', *, *, #2844, .F. ) ;
#13799=CARTESIAN_POINT ( 'NONE',  ( 235.5999999999999943, -32.43749999999999289, -51.73205080756900287 ) ) ;
#13802=CARTESIAN_POINT ( 'NONE',  ( 229.5999999999999091, -34.97364041986482164, -51.09190422181774949 ) ) ;
#13805=CARTESIAN_POINT ( 'NONE',  ( 235.3564303562499447, -34.04062499938547859, -51.59142580818350865 ) ) ;
#13810=CYLINDRICAL_SURFACE ( 'NONE', #4780, 3.000000000000009770 ) ;
#13816=CARTESIAN_POINT ( 'NONE',  ( 231.2217848218749339, -31.86562499938547788, -47.61286128772501769 ) ) ;
#13822=CARTESIAN_POINT ( 'NONE',  ( 232.5999999999999659, -32.13749999999999574, 102.9999999999999858 ) ) ;
#13826=ORIENTED_EDGE ( 'NONE', *, *, #17471, .F. ) ;
#13831=CARTESIAN_POINT ( 'NONE',  ( 235.5999999999999943, -32.83124999877096428, -51.73205080756900287 ) ) ;
#13832=CARTESIAN_POINT ( 'NONE',  ( 229.8435696437499871, -35.16562499938547148, 101.5914258081833879 ) ) ;
#13835=CARTESIAN_POINT ( 'NONE',  ( 232.5999999999999659, -32.81249999999999289, 97.00000000000000000 ) ) ;
#13837=CARTESIAN_POINT ( 'NONE',  ( 230.1700715539191435, -32.00000000000000000, 98.68659295968620881 ) ) ;
#13841=CARTESIAN_POINT ( 'NONE',  ( 232.5999999999999375, -29.99999999999999645, -53.00000000000012079 ) ) ;
#13843=CARTESIAN_POINT ( 'NONE',  ( 232.5999999999999943, -33.06562499938547717, -53.18285161636690361 ) ) ;
#13845=CARTESIAN_POINT ( 'NONE',  ( 233.9782151781249411, -32.80312499938548143, 102.3871387122750889 ) ) ;
#13846=CARTESIAN_POINT ( 'NONE',  ( 230.3018604581529871, -35.39427337414328889, -51.92835542527824089 ) ) ;
#13848=CARTESIAN_POINT ( 'NONE',  ( 233.4038475772933339, -34.81740381056766154, -47.00000000000011369 ) ) ;
#13854=VERTEX_POINT ( 'NONE', #15308 ) ;
#13861=CARTESIAN_POINT ( 'NONE',  ( 232.5999999999999375, -32.30624999877096570, 97.00000000000000000 ) ) ;
#13863=CARTESIAN_POINT ( 'NONE',  ( 229.5999999999999375, -34.85624999877096286, -48.26794919243123161 ) ) ;
#13864=CARTESIAN_POINT ( 'NONE',  ( 231.2217848218749339, -33.81562499938547717, 97.61286128772489690 ) ) ;
#13871=DIRECTION ( 'NONE',  ( -1.000000000000000000, -0.000000000000000000, -0.000000000000000000 ) ) ;
#13876=CARTESIAN_POINT ( 'NONE',  ( 229.8435696437499018, -35.11426555956767714, -51.00325860250310939 ) ) ;
#13878=VERTEX_POINT ( 'NONE', #17067 ) ;
#13883=EDGE_CURVE ( 'NONE', #1498, #4792, #13220, .T. ) ;
#13886=DIRECTION ( 'NONE',  ( 0.000000000000000000, 0.000000000000000000, -1.000000000000000000 ) ) ;
#13894=CARTESIAN_POINT ( 'NONE',  ( 235.5999999999999943, -31.98749999999999361, -51.73205080756900287 ) ) ;
#13897=CARTESIAN_POINT ( 'NONE',  ( 229.8435696437499587, -33.36562499938548143, 101.5914258081833879 ) ) ;
#13899=CARTESIAN_POINT ( 'NONE',  ( 233.9782151781249411, -32.80312499938548143, -47.61286128772501769 ) ) ;
#13907=CARTESIAN_POINT ( 'NONE',  ( 230.0666556977843697, -31.99999999999998579, -48.89901723339011852 ) ) ;
#13914=CARTESIAN_POINT ( 'NONE',  ( 235.3564303562499447, -30.77812499938547575, -51.59142580818350865 ) ) ;
#13923=( BOUNDED_CURVE ( )  B_SPLINE_CURVE ( 2, ( #17354, #5451, #15794, #12564, #5352, #11294, #9736, #15699, #17164 ),
 .UNSPECIFIED., .F., .F. ) 
 B_SPLINE_CURVE_WITH_KNOTS ( ( 3, 2, 2, 2, 3 ),
 ( 0.7291666666666667407, 0.7361111111111111605, 0.7500000000000000000, 0.7638888888888888395, 0.7708333333333332593 ),
 .UNSPECIFIED. ) 
 CURVE ( )  GEOMETRIC_REPRESENTATION_ITEM ( )  RATIONAL_B_SPLINE_CURVE ( ( 0.9330127018922192983, 0.9330127018922198534, 1.000000000000000000, 0.8660254037844387076, 1.000000000000000000, 0.8660254037844387076, 1.000000000000000000, 0.9330127018922198534, 0.9330127018922192983 ) ) 
 REPRESENTATION_ITEM ( '' )  );
#13926=EDGE_CURVE ( 'NONE', #19255, #17445, #10813, .T. ) ;
#13929=DIRECTION ( 'NONE',  ( -1.000000000000000000, 0.000000000000000000, 0.000000000000000000 ) ) ;
#13931=CARTESIAN_POINT ( 'NONE',  ( 235.3564303562499447, -34.94062499938547717, 98.40857419181659793 ) ) ;
#13934=EDGE_CURVE ( 'NONE', #14052, #3491, #18348, .T. ) ;
#13939=CYLINDRICAL_SURFACE ( 'NONE', #14885, 3.000000000000002665 ) ;
#13946=CARTESIAN_POINT ( 'NONE',  ( 235.3564303562499447, -33.21562499938548285, 101.5914258081833879 ) ) ;
#13947=CARTESIAN_POINT ( 'NONE',  ( 235.3564303562499447, -30.51562499938548001, -48.40857419181671162 ) ) ;
#13951=VERTEX_POINT ( 'NONE', #16878 ) ;
#13955=DIRECTION ( 'NONE',  ( -0.000000000000000000, 0.000000000000000000, 1.000000000000000000 ) ) ;
#13957=DIRECTION ( 'NONE',  ( 0.000000000000000000, 0.000000000000000000, 1.000000000000000000 ) ) ;
#13966=CARTESIAN_POINT ( 'NONE',  ( 229.5999999999999375, -33.99374999877096570, -50.00000000000011369 ) ) ;
#13968=CARTESIAN_POINT ( 'NONE',  ( 229.8435696437499871, -33.70312499938548001, 101.5914258081833879 ) ) ;
#13973=PLANE ( 'NONE',  #558 ) ;
#13974=ORIENTED_EDGE ( 'NONE', *, *, #162, .T. ) ;
#13978=CARTESIAN_POINT ( 'NONE',  ( 229.8435696437499303, -34.64062499938548001, -50.00000000000011369 ) ) ;
#13983=CARTESIAN_POINT ( 'NONE',  ( 234.0999999999999375, -33.29999999999999716, -52.59807621135342970 ) ) ;
#13988=DIRECTION ( 'NONE',  ( 0.000000000000000000, 6.982962677686266711E-15, -1.000000000000000000 ) ) ;
#13998=CYLINDRICAL_SURFACE ( 'NONE', #2408, 3.000000000000002665 ) ;
#13999=CARTESIAN_POINT ( 'NONE',  ( 233.9782151781249411, -33.55312499938548143, 97.61286128772489690 ) ) ;
#14001=CARTESIAN_POINT ( 'NONE',  ( 232.5999999999999375, -32.61562499938548143, -53.18285161636690361 ) ) ;
#14010=( BOUNDED_CURVE ( )  B_SPLINE_CURVE ( 2, ( #17492, #4101, #10063, #16021, #2623, #16791, #9354, #6149, #392, #7893, #7701, #15032, #1839, #6344, #9258, #3402, #13658, #9067, #7798, #15316, #3109, #485, #6437, #1742, #13753, #3015, #7510, #18074, #1932, #13843, #17877, #15225, #12295, #4786, #1654, #4583, #10633, #16599, #4486, #18261, #3204, #10543, #4683, #12194, #4878, #10820, #18164, #10440, #9163, #16506, #8972, #16405, #6249, #17973, #7606, #299, #14938, #1563, #13467, #15127, #105, #10728, #6055, #16691, #199, #3300, #12002, #13557, #12100, #11012, #7988, #15516, #2221, #6832, #6536, #15809, #16888, #6726, #8187, #3492, #3691, #18357, #8377 ),
 .UNSPECIFIED., .F., .F. ) 
 B_SPLINE_CURVE_WITH_KNOTS ( ( 3, 2, 2, 2, 2, 2, 2, 2, 2, 2, 2, 2, 2, 2, 2, 2, 2, 2, 2, 2, 2, 2, 2, 2, 2, 2, 2, 2, 2, 2, 2, 2, 2, 2, 2, 2, 2, 2, 2, 2, 2, 3 ),
 ( 0.3495698921800969861, 0.3600184345287978371, 0.3750192026341644391, 0.3900199707395310411, 0.4050207388448976431, 0.4200215069502642451, 0.4350222750556308471, 0.4500230431609974491, 0.4650238112663640511, 0.4800245793717305975, 0.4950253474770971440, 0.5100261155824636905, 0.5250268836878303480, 0.5400276517931970055, 0.5550284198985635520, 0.5700291880039300985, 0.5850299561092966449, 0.6000307242146634135, 0.6150314923200298489, 0.6300322604253965064, 0.6450330285307630529, 0.6600337966361297104, 0.6750345647414962569, 0.6900353328468626923, 0.7050361009522294609, 0.7200368690575960073, 0.7350376371629626648, 0.7500384052683291003, 0.7650391733736958688, 0.7800399414790624153, 0.7950407095844289618, 0.8100414776897955083, 0.8250422457951620547, 0.8400430139005288233, 0.8550437820058953697, 0.8700445501112619162, 0.8850453182166284627, 0.9000460863219950092, 0.9150468544273615557, 0.9300476225327283242, 0.9450483906380948707, 0.9496006163947610101 ),
 .UNSPECIFIED. ) 
 CURVE ( )  GEOMETRIC_REPRESENTATION_ITEM ( )  RATIONAL_B_SPLINE_CURVE ( ( 0.9433623850486680951, 0.9066821623815655151, 1.000000000000000000, 0.8660254037844387076, 1.000000000000000000, 0.8660254037844387076, 1.000000000000000000, 0.8660254037844387076, 1.000000000000000000, 0.8660254037844387076, 1.000000000000000000, 0.8660254037844387076, 1.000000000000000000, 0.8660254037844387076, 1.000000000000000000, 0.8660254037844387076, 1.000000000000000000, 0.8660254037844387076, 1.000000000000000000, 0.8660254037844387076, 1.000000000000000000, 0.8660254037844387076, 1.000000000000000000, 0.8660254037844387076, 1.000000000000000000, 0.8660254037844387076, 1.000000000000000000, 0.8660254037844387076, 1.000000000000000000, 0.8660254037844387076, 1.000000000000000000, 0.8660254037844387076, 1.000000000000000000, 0.8660254037844387076, 1.000000000000000000, 0.8660254037844387076, 1.000000000000000000, 0.8660254037844387076, 1.000000000000000000, 0.8660254037844387076, 1.000000000000000000, 0.8660254037844387076, 1.000000000000000000, 0.8660254037844387076, 1.000000000000000000, 0.8660254037844387076, 1.000000000000000000, 0.8660254037844387076, 1.000000000000000000, 0.8660254037844387076, 1.000000000000000000, 0.8660254037844387076, 1.000000000000000000, 0.8660254037844387076, 1.000000000000000000, 0.8660254037844387076, 1.000000000000000000, 0.8660254037844387076, 1.000000000000000000, 0.8660254037844387076, 1.000000000000000000, 0.8660254037844387076, 1.000000000000000000, 0.8660254037844387076, 1.000000000000000000, 0.8660254037844387076, 1.000000000000000000, 0.8660254037844387076, 1.000000000000000000, 0.8660254037844387076, 1.000000000000000000, 0.8660254037844387076, 1.000000000000000000, 0.8660254037844387076, 1.000000000000000000, 0.8660254037844387076, 1.000000000000000000, 0.8660254037844387076, 1.000000000000000000, 0.8660254037844387076, 1.000000000000000000, 0.9593432414028693067, 0.9433623850486648754 ) ) 
 REPRESENTATION_ITEM ( '' )  );
#14016=CARTESIAN_POINT ( 'NONE',  ( 233.9782151781249411, -31.19062499938547717, -52.38713871227520968 ) ) ;
#14019=EDGE_CURVE ( 'NONE', #1510, #18598, #6913, .T. ) ;
#14022=CARTESIAN_POINT ( 'NONE',  ( 233.4038475772933339, -34.18259618943231715, 97.00000000000000000 ) ) ;
#14029=CARTESIAN_POINT ( 'NONE',  ( 229.5999999999999375, -34.48124999877096286, -51.73205080756898866 ) ) ;
#14032=CARTESIAN_POINT ( 'NONE',  ( 232.5999999999999375, -30.25312499938548072, 96.81714838363319586 ) ) ;
#14035=PLANE ( 'NONE',  #8663 ) ;
#14036=LINE ( 'NONE', #7980, #11006 ) ;
#14041=CARTESIAN_POINT ( 'NONE',  ( 234.0999999999999375, -34.79999999999999716, 102.5980762113533018 ) ) ;
#14046=CARTESIAN_POINT ( 'NONE',  ( 235.3564303562499447, -32.72812499938547859, 99.99999999999998579 ) ) ;
#14047=CARTESIAN_POINT ( 'NONE',  ( 229.8435696437499871, -30.29062499938548214, -51.59142580818350865 ) ) ;
#14052=VERTEX_POINT ( 'NONE', #10126 ) ;
#14063=CARTESIAN_POINT ( 'NONE',  ( 233.4038475772933054, -32.51115380933862298, 102.9999999999999858 ) ) ;
#14065=CARTESIAN_POINT ( 'NONE',  ( 229.8435696437499871, -32.87812499938547717, 98.40857419181659793 ) ) ;
#14069=CARTESIAN_POINT ( 'NONE',  ( 235.5999999999999375, -31.06874999877096144, 99.99999999999998579 ) ) ;
#14080=( BOUNDED_SURFACE ( )  B_SPLINE_SURFACE ( 1, 2, ( 
 ( #9377, #11237, #2343, #8216, #797, #508, #16911, #12800, #5096, #15737, #18474, #11040, #17005, #8304, #6460, #12414, #6854, #18383, #14069, #11134, #17103, #5004, #10943, #705, #10848, #12603, #18575, #3714, #4901, #9679, #6756, #2246, #18674, #16820, #3427, #13085, #1077, #8691, #19054, #11715, #2829, #1176, #7222, #5676, #15927, #5488, #9973, #11434, #17395, #7319, #18865, #4010, #17585, #10158, #2625, #14445, #11620, #2445, #10260, #5388, #12895, #12990, #8587, #2529, #4197, #1275, #16121, #13177, #8490, #15833, #7035, #8400, #18962, #5584, #7134, #2729, #17683, #11530, #10064, #19150, #17493, #14641, #4103, #4296, #16023, #14352, #14540, #5763, #988, #16223, #8783, #14737, #1372, #18766, #6944, #11334, #17299, #3905, #9871, #17975, #7608, #7415, #12102, #6251, #4392, #10442, #14940, #5864, #16693, #15129, #1841, #10, #8974, #16406, #4788, #13272, #3302, #19247, #18076, #1565, #5959, #1745, #11816, #4488, #11907, #3016, #9260, #10635, #12004, #10730, #10349, #12196, #15227, #17880, #17785 ),
 ( #7511, #13560, #16314, #2923, #8875, #13376, #13468, #3110, #107, #4684, #7703, #201, #13660, #6058, #14835, #16601, #15033, #3206, #9165, #18166, #1461, #301, #4585, #10545, #16507, #9069, #1656, #6151, #393, #11014, #3404, #9658, #4879, #2136, #3494, #11215, #15617, #16794, #14139, #6537, #12483, #9453, #6439, #16890, #10822, #17180, #16980, #9357, #15419, #18547, #18359, #3783, #6727, #18263, #774, #9552, #12581, #18647, #486, #12674, #12297, #15318, #5270, #1934, #3592, #8092, #14046, #7895, #13845, #12390, #13755, #4981, #18452, #10922, #9750, #2030, #3692, #7990, #681, #13946, #15714, #6632, #586, #17078, #5164, #7800, #6345, #15518, #2223, #11110, #5073, #8189, #12871, #14330, #8379, #10233, #2415, #6923, #1150, #13064, #5557, #17369, #15999, #5365, #13148, #8282, #15810, #15904, #11507, #968, #7108, #4176, #2603, #16096, #18842, #18747, #19029, #4079, #5651, #11596, #7199, #2318, #17564, #11690, #2701, #5465, #11409, #10136, #8564, #14231, #17468, #17278, #8660, #11312, #14517 ) ),
 .UNSPECIFIED., .F., .F., .F. ) 
 B_SPLINE_SURFACE_WITH_KNOTS ( ( 2, 2 ),
 ( 3, 2, 2, 2, 2, 2, 2, 2, 2, 2, 2, 2, 2, 2, 2, 2, 2, 2, 2, 2, 2, 2, 2, 2, 2, 2, 2, 2, 2, 2, 2, 2, 2, 2, 2, 2, 2, 2, 2, 2, 2, 2, 2, 2, 2, 2, 2, 2, 2, 2, 2, 2, 2, 2, 2, 2, 2, 2, 2, 2, 2, 2, 2, 2, 2, 2, 2, 3 ),
 ( 0.000000000000000000, 1.000000000000000000 ),
 ( 0.000000000000000000, 0.01388888888888888812, 0.02777777777777777624, 0.04166666666666666435, 0.05555555555555555247, 0.06944444444444444753, 0.08333333333333332871, 0.09722222222222222376, 0.1111111111111111049, 0.1250000000000000000, 0.1388888888888888951, 0.1527777777777777901, 0.1666666666666666574, 0.1805555555555555525, 0.1944444444444444475, 0.2083333333333333426, 0.2222222222222222099, 0.2361111111111111049, 0.2500000000000000000, 0.2638888888888888951, 0.2777777777777777901, 0.2916666666666666852, 0.3055555555555555802, 0.3194444444444444198, 0.3333333333333333148, 0.3472222222222222099, 0.3611111111111111049, 0.3750000000000000000, 0.3888888888888888951, 0.4027777777777777901, 0.4166666666666666852, 0.4305555555555555802, 0.4444444444444444198, 0.4583333333333333148, 0.4722222222222222099, 0.4861111111111111049, 0.5000000000000000000, 0.5138888888888888395, 0.5277777777777777901, 0.5416666666666666297, 0.5555555555555555802, 0.5694444444444444198, 0.5833333333333333703, 0.5972222222222222099, 0.6111111111111111605, 0.6250000000000000000, 0.6388888888888888395, 0.6527777777777777901, 0.6666666666666666297, 0.6805555555555555802, 0.6944444444444444198, 0.7083333333333333703, 0.7222222222222222099, 0.7361111111111111605, 0.7500000000000000000, 0.7638888888888888395, 0.7777777777777777901, 0.7916666666666666297, 0.8055555555555555802, 0.8194444444444444198, 0.8333333333333333703, 0.8472222222222222099, 0.8611111111111111605, 0.8750000000000000000, 0.8888888888888888395, 0.9027777777777777901, 0.9166666666666666297, 0.9258785144422092550 ),
 .UNSPECIFIED. ) 
 GEOMETRIC_REPRESENTATION_ITEM ( )  RATIONAL_B_SPLINE_SURFACE ( (
 ( 1.000000000000000000, 0.8660254037844387076, 1.000000000000000000, 0.8660254037844387076, 1.000000000000000000, 0.8660254037844387076, 1.000000000000000000, 0.8660254037844387076, 1.000000000000000000, 0.8660254037844387076, 1.000000000000000000, 0.8660254037844387076, 1.000000000000000000, 0.8660254037844387076, 1.000000000000000000, 0.8660254037844387076, 1.000000000000000000, 0.8660254037844387076, 1.000000000000000000, 0.8660254037844387076, 1.000000000000000000, 0.8660254037844387076, 1.000000000000000000, 0.8660254037844387076, 1.000000000000000000, 0.8660254037844387076, 1.000000000000000000, 0.8660254037844387076, 1.000000000000000000, 0.8660254037844387076, 1.000000000000000000, 0.8660254037844387076, 1.000000000000000000, 0.8660254037844387076, 1.000000000000000000, 0.8660254037844387076, 1.000000000000000000, 0.8660254037844387076, 1.000000000000000000, 0.8660254037844387076, 1.000000000000000000, 0.8660254037844387076, 1.000000000000000000, 0.8660254037844387076, 1.000000000000000000, 0.8660254037844387076, 1.000000000000000000, 0.8660254037844387076, 1.000000000000000000, 0.8660254037844387076, 1.000000000000000000, 0.8660254037844387076, 1.000000000000000000, 0.8660254037844387076, 1.000000000000000000, 0.8660254037844387076, 1.000000000000000000, 0.8660254037844387076, 1.000000000000000000, 0.8660254037844387076, 1.000000000000000000, 0.8660254037844387076, 1.000000000000000000, 0.8660254037844387076, 1.000000000000000000, 0.8660254037844387076, 1.000000000000000000, 0.8660254037844387076, 1.000000000000000000, 0.8660254037844387076, 1.000000000000000000, 0.8660254037844387076, 1.000000000000000000, 0.8660254037844387076, 1.000000000000000000, 0.8660254037844387076, 1.000000000000000000, 0.8660254037844387076, 1.000000000000000000, 0.8660254037844387076, 1.000000000000000000, 0.8660254037844387076, 1.000000000000000000, 0.8660254037844387076, 1.000000000000000000, 0.8660254037844387076, 1.000000000000000000, 0.8660254037844387076, 1.000000000000000000, 0.8660254037844387076, 1.000000000000000000, 0.8660254037844387076, 1.000000000000000000, 0.8660254037844387076, 1.000000000000000000, 0.8660254037844387076, 1.000000000000000000, 0.8660254037844387076, 1.000000000000000000, 0.8660254037844387076, 1.000000000000000000, 0.8660254037844387076, 1.000000000000000000, 0.8660254037844387076, 1.000000000000000000, 0.8660254037844387076, 1.000000000000000000, 0.8660254037844387076, 1.000000000000000000, 0.8660254037844387076, 1.000000000000000000, 0.8660254037844387076, 1.000000000000000000, 0.8660254037844387076, 1.000000000000000000, 0.8660254037844387076, 1.000000000000000000, 0.8660254037844387076, 1.000000000000000000, 0.8660254037844387076, 1.000000000000000000, 0.8660254037844387076, 1.000000000000000000, 0.8660254037844387076, 1.000000000000000000, 0.8660254037844387076, 1.000000000000000000, 0.8660254037844387076, 1.000000000000000000, 0.8660254037844387076, 1.000000000000000000, 0.8660254037844387076, 1.000000000000000000, 0.9111409417988175496, 0.9401539645359766606),
 ( 1.000000000000000000, 0.8660254037844387076, 1.000000000000000000, 0.8660254037844387076, 1.000000000000000000, 0.8660254037844387076, 1.000000000000000000, 0.8660254037844387076, 1.000000000000000000, 0.8660254037844387076, 1.000000000000000000, 0.8660254037844387076, 1.000000000000000000, 0.8660254037844387076, 1.000000000000000000, 0.8660254037844387076, 1.000000000000000000, 0.8660254037844387076, 1.000000000000000000, 0.8660254037844387076, 1.000000000000000000, 0.8660254037844387076, 1.000000000000000000, 0.8660254037844387076, 1.000000000000000000, 0.8660254037844387076, 1.000000000000000000, 0.8660254037844387076, 1.000000000000000000, 0.8660254037844387076, 1.000000000000000000, 0.8660254037844387076, 1.000000000000000000, 0.8660254037844387076, 1.000000000000000000, 0.8660254037844387076, 1.000000000000000000, 0.8660254037844387076, 1.000000000000000000, 0.8660254037844387076, 1.000000000000000000, 0.8660254037844387076, 1.000000000000000000, 0.8660254037844387076, 1.000000000000000000, 0.8660254037844387076, 1.000000000000000000, 0.8660254037844387076, 1.000000000000000000, 0.8660254037844387076, 1.000000000000000000, 0.8660254037844387076, 1.000000000000000000, 0.8660254037844387076, 1.000000000000000000, 0.8660254037844387076, 1.000000000000000000, 0.8660254037844387076, 1.000000000000000000, 0.8660254037844387076, 1.000000000000000000, 0.8660254037844387076, 1.000000000000000000, 0.8660254037844387076, 1.000000000000000000, 0.8660254037844387076, 1.000000000000000000, 0.8660254037844387076, 1.000000000000000000, 0.8660254037844387076, 1.000000000000000000, 0.8660254037844387076, 1.000000000000000000, 0.8660254037844387076, 1.000000000000000000, 0.8660254037844387076, 1.000000000000000000, 0.8660254037844387076, 1.000000000000000000, 0.8660254037844387076, 1.000000000000000000, 0.8660254037844387076, 1.000000000000000000, 0.8660254037844387076, 1.000000000000000000, 0.8660254037844387076, 1.000000000000000000, 0.8660254037844387076, 1.000000000000000000, 0.8660254037844387076, 1.000000000000000000, 0.8660254037844387076, 1.000000000000000000, 0.8660254037844387076, 1.000000000000000000, 0.8660254037844387076, 1.000000000000000000, 0.8660254037844387076, 1.000000000000000000, 0.8660254037844387076, 1.000000000000000000, 0.8660254037844387076, 1.000000000000000000, 0.8660254037844387076, 1.000000000000000000, 0.8660254037844387076, 1.000000000000000000, 0.8660254037844387076, 1.000000000000000000, 0.8660254037844387076, 1.000000000000000000, 0.8660254037844387076, 1.000000000000000000, 0.8660254037844387076, 1.000000000000000000, 0.8660254037844387076, 1.000000000000000000, 0.8660254037844387076, 1.000000000000000000, 0.8660254037844387076, 1.000000000000000000, 0.8660254037844387076, 1.000000000000000000, 0.8660254037844387076, 1.000000000000000000, 0.8660254037844387076, 1.000000000000000000, 0.8660254037844387076, 1.000000000000000000, 0.8660254037844387076, 1.000000000000000000, 0.8660254037844387076, 1.000000000000000000, 0.9111409417988175496, 0.9401539645359766606) ) ) 
 REPRESENTATION_ITEM ( '' )  SURFACE ( )  );
#14084=LINE ( 'NONE', #1978, #1648 ) ;
#14093=CARTESIAN_POINT ( 'NONE',  ( 231.2217848218749339, -32.57812499938548001, 97.61286128772489690 ) ) ;
#14095=CARTESIAN_POINT ( 'NONE',  ( 235.3564303562499447, -30.81562499938547717, -50.00000000000011369 ) ) ;
#14102=VECTOR ( 'NONE', #17984, 1000.000000000000000 ) ;
#14108=CARTESIAN_POINT ( 'NONE',  ( 232.5999999999999375, -32.50312499938547717, -53.18285161636690361 ) ) ;
#14111=ORIENTED_EDGE ( 'NONE', *, *, #12736, .F. ) ;
#14120=CARTESIAN_POINT ( 'NONE',  ( 231.0429922824658320, -35.00000000000000711, -52.57249805494185324 ) ) ;
#14121=PLANE ( 'NONE',  #7966 ) ;
#14123=CARTESIAN_POINT ( 'NONE',  ( 235.3564303562499447, -32.20312499938548001, 101.5914258081833879 ) ) ;
#14129=AXIS2_PLACEMENT_3D ( 'NONE', #7718, #13288, #17895 ) ;
#14130=( BOUNDED_CURVE ( )  B_SPLINE_CURVE ( 2, ( #7831, #4910, #3434, #9385, #6469, #12421, #15744, #9686, #2452 ),
 .UNSPECIFIED., .F., .F. ) 
 B_SPLINE_CURVE_WITH_KNOTS ( ( 3, 2, 2, 2, 3 ),
 ( 0.5625000000000001110, 0.5694444444444444198, 0.5833333333333333703, 0.5972222222222222099, 0.6041666666666667407 ),
 .UNSPECIFIED. ) 
 CURVE ( )  GEOMETRIC_REPRESENTATION_ITEM ( )  RATIONAL_B_SPLINE_CURVE ( ( 0.9330127018922194093, 0.9330127018922204085, 1.000000000000000000, 0.8660254037844387076, 1.000000000000000000, 0.8660254037844387076, 1.000000000000000000, 0.9330127018922187432, 0.9330127018922192983 ) ) 
 REPRESENTATION_ITEM ( '' )  );
#14134=CARTESIAN_POINT ( 'NONE',  ( 230.3018593135002448, -35.00052333152935802, 98.07164593887567605 ) ) ;
#14139=CARTESIAN_POINT ( 'NONE',  ( 231.2217848218749339, -31.67812499938547788, 97.61286128772489690 ) ) ;
#14140=CARTESIAN_POINT ( 'NONE',  ( 231.2217848218749339, -32.12812499938547717, -52.38713871227520968 ) ) ;
#14149=ORIENTED_EDGE ( 'NONE', *, *, #458, .T. ) ;
#14153=CARTESIAN_POINT ( 'NONE',  ( 105.1999999999999744, -4.999999999999976907, 150.0000000000000000 ) ) ;
#14157=DIRECTION ( 'NONE',  ( -1.000000000000000000, 0.000000000000000000, -0.000000000000000000 ) ) ;
#14159=CARTESIAN_POINT ( 'NONE',  ( 235.3140393761304665, -32.00000000000000000, 101.2782762865722361 ) ) ;
#14160=CARTESIAN_POINT ( 'NONE',  ( 229.8435696437499303, -34.19062499938547717, 99.99999999999998579 ) ) ;
#14164=DIRECTION ( 'NONE',  ( 0.000000000000000000, 0.000000000000000000, 1.000000000000000000 ) ) ;
#14165=CARTESIAN_POINT ( 'NONE',  ( 231.0999999999999375, -30.46874999877096002, -52.59807621135342970 ) ) ;
#14166=EDGE_LOOP ( 'NONE', ( #2809, #16170, #13512, #13384 ) ) ;
#14175=EDGE_CURVE ( 'NONE', #804, #15440, #11778, .T. ) ;
#14180=CARTESIAN_POINT ( 'NONE',  ( 229.8435696437499018, -35.11426555956767714, 98.99674139749697588 ) ) ;
#14181=CARTESIAN_POINT ( 'NONE',  ( 231.7961524227065695, -32.10134618820329422, -47.00000000000011369 ) ) ;
#14186=CARTESIAN_POINT ( 'NONE',  ( 231.0999999999999375, -34.57499999999999574, -52.59807621135342970 ) ) ;
#14190=CARTESIAN_POINT ( 'NONE',  ( 235.3564303562499447, -32.31562499938547717, 101.5914258081833879 ) ) ;
#14192=CARTESIAN_POINT ( 'NONE',  ( 229.8435696437499303, -30.14062499938548001, -50.00000000000011369 ) ) ;
#14199=CARTESIAN_POINT ( 'NONE',  ( 230.9489134087919524, -32.00820041275123629, -52.22959632847759082 ) ) ;
#14204=CARTESIAN_POINT ( 'NONE',  ( 235.3564303562499447, -33.10312499938547859, -48.40857419181671162 ) ) ;
#14208=CARTESIAN_POINT ( 'NONE',  ( 229.5999999999999375, -32.28749999999999432, 98.26794919243111792 ) ) ;
#14212=LINE ( 'NONE', #2396, #9922 ) ;
#14224=LINE ( 'NONE', #9838, #16179 ) ;
#14227=LINE ( 'NONE', #17465, #8026 ) ;
#14228=EDGE_CURVE ( 'NONE', #11694, #5568, #2979, .T. ) ;
#14231=CARTESIAN_POINT ( 'NONE',  ( 232.5999999999999375, -35.09062499938547575, 103.1828516163667899 ) ) ;
#14232=CARTESIAN_POINT ( 'NONE',  ( 235.3564303562499447, -32.76562499938548001, -48.40857419181671162 ) ) ;
#14239=LINE ( 'NONE', #11221, #713 ) ;
#14251=EDGE_CURVE ( 'NONE', #12317, #16053, #9615, .T. ) ;
#14253=VECTOR ( 'NONE', #5285, 1000.000000000000000 ) ;
#14254=CARTESIAN_POINT ( 'NONE',  ( 231.0999999999999375, -30.07499999999999574, 97.40192378864668399 ) ) ;
#14255=ORIENTED_EDGE ( 'NONE', *, *, #14754, .T. ) ;
#14258=CARTESIAN_POINT ( 'NONE',  ( 235.5999999999999375, -31.96874999877096002, -50.00000000000011369 ) ) ;
#14271=MECHANICAL_DESIGN_GEOMETRIC_PRESENTATION_REPRESENTATION('',(#17080),#3676);
#14276=CARTESIAN_POINT ( 'NONE',  ( 232.8516854624778887, -31.99999999999997868, -52.85844335754083545 ) ) ;
#14283=CARTESIAN_POINT ( 'NONE',  ( 229.5999999999999659, -34.97364041986482874, -51.09190422181774949 ) ) ;
#14284=CARTESIAN_POINT ( 'NONE',  ( 232.5999999999999091, -34.10624999877096286, 96.99999999999998579 ) ) ;
#14285=CIRCLE ( 'NONE', #15220, 5.199999999999996625 ) ;
#14287=DIRECTION ( 'NONE',  ( -1.000000000000000000, 0.000000000000000000, -0.000000000000000000 ) ) ;
#14289=CARTESIAN_POINT ( 'NONE',  ( 233.9782151781249411, -31.34062499938548285, -47.61286128772501769 ) ) ;
#14298=CARTESIAN_POINT ( 'NONE',  ( 231.2217848218749339, -32.76562499938548001, -47.61286128772501769 ) ) ;
#14303=CARTESIAN_POINT ( 'NONE',  ( 235.3564303562499447, -33.96562499938547575, -50.00000000000011369 ) ) ;
#14307=DIRECTION ( 'NONE',  ( -0.000000000000000000, -1.000000000000000000, -0.000000000000000000 ) ) ;
#14315=CARTESIAN_POINT ( 'NONE',  ( 231.7961524227065695, -34.35134618820329422, -47.00000000000009948 ) ) ;
#14323=CARTESIAN_POINT ( 'NONE',  ( 235.3140393761304665, -32.00000000000000000, 101.2782762865722361 ) ) ;
#14330=CARTESIAN_POINT ( 'NONE',  ( 232.5999999999999375, -33.74062499938548143, 103.1828516163667899 ) ) ;
#14331=CARTESIAN_POINT ( 'NONE',  ( 235.3564303562499447, -33.66562499938548569, -48.40857419181671162 ) ) ;
#14333=CARTESIAN_POINT ( 'NONE',  ( 232.5999999999999375, -32.81249999999999289, -53.00000000000011369 ) ) ;
#14349=CARTESIAN_POINT ( 'NONE',  ( 232.5999999999999375, -30.56250000000000000, 96.53589838486223584 ) ) ;
#14352=CARTESIAN_POINT ( 'NONE',  ( 229.5999999999999375, -33.58124999877096428, 98.26794919243111792 ) ) ;
#14353=CARTESIAN_POINT ( 'NONE',  ( 231.0999999999999375, -31.81874999877096144, -52.59807621135342970 ) ) ;
#14355=DIRECTION ( 'NONE',  ( -1.000000000000000000, 0.000000000000000000, 0.000000000000000000 ) ) ;
#14357=LINE ( 'NONE', #6664, #11920 ) ;
#14370=ADVANCED_FACE ( 'NONE', ( #5806 ), #14579, .F. ) ;
#14374=CARTESIAN_POINT ( 'NONE',  ( 232.5999999999999375, -34.78124999877096002, -47.00000000000011369 ) ) ;
#14375=ORIENTED_EDGE ( 'NONE', *, *, #11858, .F. ) ;
#14376=CARTESIAN_POINT ( 'NONE',  ( 235.5999999999999943, -34.31249999999999289, -48.26794919243124582 ) ) ;
#14379=CARTESIAN_POINT ( 'NONE',  ( 235.3564303562499447, -34.07812499938548001, 99.99999999999998579 ) ) ;
#14381=CARTESIAN_POINT ( 'NONE',  ( 233.9782151781249411, -31.64062499938547646, -52.38713871227520968 ) ) ;
#14383=ORIENTED_EDGE ( 'NONE', *, *, #5896, .F. ) ;
#14394=CARTESIAN_POINT ( 'NONE',  ( 235.3564303562499447, -34.00312499938547717, -48.40857419181671162 ) ) ;
#14404=AXIS2_PLACEMENT_3D ( 'NONE', #7952, #4937, #17140 ) ;
#14405=CARTESIAN_POINT ( 'NONE',  ( 235.3564303562499447, -32.61562499938548143, 99.99999999999998579 ) ) ;
#14411=LINE ( 'NONE', #8553, #1344 ) ;
#14412=CARTESIAN_POINT ( 'NONE',  ( 244.7999999999999545, -32.00000000000000000, -100.0000000000000000 ) ) ;
#14414=CARTESIAN_POINT ( 'NONE',  ( 233.4038475772933339, -32.06115380933863435, 103.0000000000000000 ) ) ;
#14423=CARTESIAN_POINT ( 'NONE',  ( 233.0319854768594041, -35.00000000000000000, -47.27181766474440394 ) ) ;
#14424=CARTESIAN_POINT ( 'NONE',  ( 235.3564303562499447, -33.21562499938548285, -48.40857419181671162 ) ) ;
#14427=ORIENTED_EDGE ( 'NONE', *, *, #11525, .T. ) ;
#14437=CYLINDRICAL_SURFACE ( 'NONE', #18207, 3.000000000000009770 ) ;
#14441=CARTESIAN_POINT ( 'NONE',  ( 229.5999999999999375, -31.38749999999999218, 98.26794919243111792 ) ) ;
#14445=CARTESIAN_POINT ( 'NONE',  ( 235.5999999999999943, -32.45624999877096428, 101.7320508075688537 ) ) ;
#14446=CARTESIAN_POINT ( 'NONE',  ( 235.5999999999999943, -30.65624999877095647, -48.26794919243124582 ) ) ;
#14447=CARTESIAN_POINT ( 'NONE',  ( 231.7961524227065695, -32.73615380933862440, 96.99999999999995737 ) ) ;
#14449=VERTEX_POINT ( 'NONE', #4703 ) ;
#14452=LINE ( 'NONE', #16128, #15044 ) ;
#14458=CARTESIAN_POINT ( 'NONE',  ( 234.1461053235293548, -35.00000000000002132, -52.48908440345743998 ) ) ;
#14460=CARTESIAN_POINT ( 'NONE',  ( 232.5999999999999091, -32.08124999877096428, -47.00000000000011369 ) ) ;
#14467=EDGE_CURVE ( 'NONE', #6637, #11529, #8626, .T. ) ;
#14470=CARTESIAN_POINT ( 'NONE',  ( 231.2217848218749339, -34.37812499938547717, 97.61286128772489690 ) ) ;
#14472=FACE_OUTER_BOUND ( 'NONE', #10894, .T. ) ;
#14473=CARTESIAN_POINT ( 'NONE',  ( 229.8435696437499018, -35.22676555956767430, -51.00325860250310939 ) ) ;
#14479=DIRECTION ( 'NONE',  ( -1.000000000000000000, -0.000000000000000000, -0.000000000000000000 ) ) ;
#14480=CARTESIAN_POINT ( 'NONE',  ( 229.8435696437499871, -30.55312499938547788, 101.5914258081833879 ) ) ;
#14485=ADVANCED_FACE ( 'NONE', ( #15145 ), #15538, .F. ) ;
#14487=CARTESIAN_POINT ( 'NONE',  ( 232.5999999999999375, -34.07812499938548001, -46.81714838363331666 ) ) ;
#14490=EDGE_CURVE ( 'NONE', #12222, #4900, #4098, .T. ) ;
#14500=CARTESIAN_POINT ( 'NONE',  ( 235.3564303562499447, -32.12812499938547717, 98.40857419181659793 ) ) ;
#14511=CARTESIAN_POINT ( 'NONE',  ( 231.0999999999999375, -34.12499999999999289, 97.40192378864668399 ) ) ;
#14514=( BOUNDED_CURVE ( )  B_SPLINE_CURVE ( 2, ( #15058, #32, #6083, #9004, #16337, #11934, #4324, #133, #10376 ),
 .UNSPECIFIED., .F., .F. ) 
 B_SPLINE_CURVE_WITH_KNOTS ( ( 3, 2, 2, 2, 3 ),
 ( 0.7708333333333332593, 0.7777777777777777901, 0.7916666666666666297, 0.8055555555555555802, 0.8125000000000000000 ),
 .UNSPECIFIED. ) 
 CURVE ( )  GEOMETRIC_REPRESENTATION_ITEM ( )  RATIONAL_B_SPLINE_CURVE ( ( 0.9330127018922192983, 0.9330127018922187432, 1.000000000000000000, 0.8660254037844387076, 1.000000000000000000, 0.8660254037844387076, 1.000000000000000000, 0.9330127018922194093, 0.9330127018922194093 ) ) 
 REPRESENTATION_ITEM ( '' )  );
#14517=CARTESIAN_POINT ( 'NONE',  ( 230.4884461346514968, -35.25364837475780178, 98.22820752270799005 ) ) ;
#14526=DIRECTION ( 'NONE',  ( 0.000000000000000000, 0.000000000000000000, 1.000000000000000000 ) ) ;
#14527=EDGE_CURVE ( 'NONE', #16633, #1370, #11347, .T. ) ;
#14535=CARTESIAN_POINT ( 'NONE',  ( 231.0999999999999375, -32.17499999999999716, -47.40192378864679768 ) ) ;
#14537=CARTESIAN_POINT ( 'NONE',  ( 235.5999999999999943, -31.16249999999999432, 101.7320508075688537 ) ) ;
#14540=CARTESIAN_POINT ( 'NONE',  ( 231.0999999999999375, -33.61874999877096570, 97.40192378864668399 ) ) ;
#14541=CARTESIAN_POINT ( 'NONE',  ( 235.5999999999999375, -31.06874999877096144, -50.00000000000011369 ) ) ;
#14542=CARTESIAN_POINT ( 'NONE',  ( 232.5999999999999091, -34.38749999999999574, 102.9999999999999858 ) ) ;
#14544=ORIENTED_EDGE ( 'NONE', *, *, #16870, .T. ) ;
#14547=DIRECTION ( 'NONE',  ( -0.000000000000000000, -1.000000000000000000, -0.000000000000000000 ) ) ;
#14558=CARTESIAN_POINT ( 'NONE',  ( 231.2217848218749339, -31.11562499938547788, 97.61286128772489690 ) ) ;
#14559=ORIENTED_EDGE ( 'NONE', *, *, #13471, .T. ) ;
#14564=CARTESIAN_POINT ( 'NONE',  ( 234.6787480663870156, -35.00000000000000711, 97.97655282300767965 ) ) ;
#14566=CARTESIAN_POINT ( 'NONE',  ( 235.3564303562499447, -34.04062499938548569, 98.40857419181659793 ) ) ;
#14568=CARTESIAN_POINT ( 'NONE',  ( 231.2217848218749339, -32.91562499938547148, -52.38713871227520968 ) ) ;
#14575=B_SPLINE_CURVE_WITH_KNOTS ( 'NONE', 3,
 ( #17699, #7049, #10276, #18783, #16238, #2843, #13008, #14276, #912, #18977, #6871, #11351, #2461, #12913, #18881, #317, #5881, #17991 ),
 .UNSPECIFIED., .F., .F.,
 ( 4, 2, 2, 2, 2, 2, 2, 2, 4 ),
 ( 0.000000000000000000, 0.0007089252359835750269, 0.001417850471967150054, 0.002126775707950724972, 0.002835700943934300108, 0.003544626179917875243, 0.004253551415901449945, 0.004962476651885025514, 0.005671401887868600215 ),
 .UNSPECIFIED. ) ;
#14577=CARTESIAN_POINT ( 'NONE',  ( 235.3564303562499447, -32.16562499938547859, 99.99999999999998579 ) ) ;
#14578=CARTESIAN_POINT ( 'NONE',  ( 235.3564303562499447, -32.57812499938548001, -51.59142580818350154 ) ) ;
#14579=CYLINDRICAL_SURFACE ( 'NONE', #11762, 3.000000000000002665 ) ;
#14588=CARTESIAN_POINT ( 'NONE',  ( 231.0999999999999375, -30.07499999999999574, -52.59807621135342970 ) ) ;
#14593=CARTESIAN_POINT ( 'NONE',  ( 235.5999999999999943, -34.18124999877096570, -51.73205080756900287 ) ) ;
#14597=CARTESIAN_POINT ( 'NONE',  ( 232.5999999999999375, -29.99999999999999645, -50.00000000000011369 ) ) ;
#14598=VECTOR ( 'NONE', #16814, 1000.000000000000000 ) ;
#14601=EDGE_CURVE ( 'NONE', #17445, #18941, #16998, .T. ) ;
#14602=CARTESIAN_POINT ( 'NONE',  ( 231.2217848218749339, -33.66562499938547859, 102.3871387122750889 ) ) ;
#14606=CARTESIAN_POINT ( 'NONE',  ( 235.0681666926251410, -32.00000000000000000, -48.31447495408071546 ) ) ;
#14610=EDGE_CURVE ( 'NONE', #3788, #11625, #19263, .T. ) ;
#14614=ORIENTED_EDGE ( 'NONE', *, *, #12687, .F. ) ;
#14617=CARTESIAN_POINT ( 'NONE',  ( 235.2218879900010506, -35.00000000000000000, -49.14934632385183022 ) ) ;
#14618=PLANE ( 'NONE',  #7418 ) ;
#14629=CARTESIAN_POINT ( 'NONE',  ( 229.8435696437499303, -31.15312499938548285, 99.99999999999998579 ) ) ;
#14637=CARTESIAN_POINT ( 'NONE',  ( 232.5999999999999375, -31.01249999999999218, 96.53589838486223584 ) ) ;
#14640=EDGE_CURVE ( 'NONE', #5496, #11985, #6364, .T. ) ;
#14641=CARTESIAN_POINT ( 'NONE',  ( 232.5999999999999375, -33.43124999877096570, 103.4641016151377499 ) ) ;
#14642=CARTESIAN_POINT ( 'NONE',  ( 232.5999999999999375, -33.43124999877096570, -46.53589838486234953 ) ) ;
#14649=VERTEX_POINT ( 'NONE', #2822 ) ;
#14656=CARTESIAN_POINT ( 'NONE',  ( 232.3466685930879123, -34.99995246259152282, -52.98928446312130802 ) ) ;
#14658=ADVANCED_FACE ( 'NONE', ( #4002 ), #10059, .F. ) ;
#14661=CARTESIAN_POINT ( 'NONE',  ( 229.8435696437499871, -30.62812499938547717, 98.40857419181659793 ) ) ;
#14667=CARTESIAN_POINT ( 'NONE',  ( 232.5999999999999943, -34.86562499938548143, 96.81714838363319586 ) ) ;
#14669=DIRECTION ( 'NONE',  ( -0.000000000000000000, -1.000000000000000000, -0.000000000000000000 ) ) ;
#14670=CARTESIAN_POINT ( 'NONE',  ( 229.8435696437499303, -33.74062499938548143, -50.00000000000011369 ) ) ;
#14671=ORIENTED_EDGE ( 'NONE', *, *, #2844, .T. ) ;
#14678=CARTESIAN_POINT ( 'NONE',  ( 229.8435696437499871, -30.62812499938547717, 98.40857419181659793 ) ) ;
#14679=CARTESIAN_POINT ( 'NONE',  ( 232.5999999999999943, -33.85312499938547859, -53.18285161636690361 ) ) ;
#14684=CARTESIAN_POINT ( 'NONE',  ( 232.5999999999999375, -30.56250000000000000, -53.46410161513786363 ) ) ;
#14690=CARTESIAN_POINT ( 'NONE',  ( 235.3564303562499447, -31.86562499938547788, -48.40857419181671162 ) ) ;
#14694=CARTESIAN_POINT ( 'NONE',  ( 105.1999999999999886, -32.00000000000000711, -97.80000000000002558 ) ) ;
#14699=CARTESIAN_POINT ( 'NONE',  ( 230.5523683116323355, -32.00000000000000000, -48.15470523285603832 ) ) ;
#14701=PLANE ( 'NONE',  #525 ) ;
#14707=ORIENTED_EDGE ( 'NONE', *, *, #16190, .F. ) ;
#14710=DIRECTION ( 'NONE',  ( -0.000000000000000000, 0.000000000000000000, -1.000000000000000000 ) ) ;
#14711=VECTOR ( 'NONE', #12762, 1000.000000000000000 ) ;
#14724=CARTESIAN_POINT ( 'NONE',  ( 229.8435696437499871, -30.74062499938547433, 98.40857419181659793 ) ) ;
#14729=VECTOR ( 'NONE', #13116, 1000.000000000000000 ) ;
#14730=CARTESIAN_POINT ( 'NONE',  ( 234.9210568921013191, -34.99999999999998579, 101.4973817956047668 ) ) ;
#14733=CARTESIAN_POINT ( 'NONE',  ( 231.0999999999999375, -33.52499999999999147, 102.5980762113533018 ) ) ;
#14735=ORIENTED_EDGE ( 'NONE', *, *, #4601, .F. ) ;
#14737=CARTESIAN_POINT ( 'NONE',  ( 235.5999999999999943, -33.80624999877096570, 101.7320508075688537 ) ) ;
#14738=CARTESIAN_POINT ( 'NONE',  ( 231.0999999999999375, -32.56874999877096144, -47.40192378864679768 ) ) ;
#14754=EDGE_CURVE ( 'NONE', #5593, #15949, #4620, .T. ) ;
#14760=( BOUNDED_CURVE ( )  B_SPLINE_CURVE ( 2, ( #1332, #10314, #18921, #2494, #7278, #14500, #19207, #8452, #11582, #7185, #5822, #1231, #1132, #11677, #17748, #17643, #4351, #18827, #14405, #2883, #1044, #16271, #8839, #7375, #5450, #6996, #17547, #12949, #8548, #10215, #2587, #16077, #7091, #17353, #19108, #10121, #13048, #3963, #13134, #19016, #5542, #5728, #4163, #17453, #4066, #8642, #14602, #10690, #12160, #14996, #3072, #7764, #4543, #4743, #14894, #13717, #4842, #19309, #7474, #7568, #3165, #1705, #15281, #358, #5920, #6213, #1896, #10598, #3361, #4649, #10403, #13522, #9217, #10785, #13431, #16367, #3259, #9032, #16657, #2975, #159, #16562, #8931 ),
 .UNSPECIFIED., .F., .F. ) 
 B_SPLINE_CURVE_WITH_KNOTS ( ( 3, 2, 2, 2, 2, 2, 2, 2, 2, 2, 2, 2, 2, 2, 2, 2, 2, 2, 2, 2, 2, 2, 2, 2, 2, 2, 2, 2, 2, 2, 2, 2, 2, 2, 2, 2, 2, 2, 2, 2, 2, 3 ),
 ( 0.3716916592826012278, 0.3750191855951753306, 0.3900199530189823460, 0.4050207204427893615, 0.4200214878665964324, 0.4350222552904034479, 0.4500230227142104633, 0.4650237901380174788, 0.4800245575618244387, 0.4950253249856314541, 0.5100260924094385251, 0.5250268598332454850, 0.5400276272570525560, 0.5550283946808595159, 0.5700291621046665869, 0.5850299295284735468, 0.6000306969522806178, 0.6150314643760875777, 0.6300322317998946486, 0.6450329992237016086, 0.6600337666475086795, 0.6750345340713157505, 0.6900353014951225994, 0.7050360689189296703, 0.7200368363427367413, 0.7350376037665438123, 0.7500383711903507722, 0.7650391386141577321, 0.7800399060379648031, 0.7950406734617718740, 0.8100414408855788340, 0.8250422083093857939, 0.8400429757331928649, 0.8550437431569999358, 0.8700445105808070068, 0.8850452780046138557, 0.9000460454284209266, 0.9150468128522277755, 0.9300475802760350685, 0.9450483476998419174, 0.9600491151236489884, 0.9717223562348840105 ),
 .UNSPECIFIED. ) 
 CURVE ( )  GEOMETRIC_REPRESENTATION_ITEM ( )  RATIONAL_B_SPLINE_CURVE ( ( 0.9537471549767004841, 0.9702812541832854798, 1.000000000000000000, 0.8660254037844387076, 1.000000000000000000, 0.8660254037844387076, 1.000000000000000000, 0.8660254037844387076, 1.000000000000000000, 0.8660254037844387076, 1.000000000000000000, 0.8660254037844387076, 1.000000000000000000, 0.8660254037844387076, 1.000000000000000000, 0.8660254037844387076, 1.000000000000000000, 0.8660254037844387076, 1.000000000000000000, 0.8660254037844387076, 1.000000000000000000, 0.8660254037844387076, 1.000000000000000000, 0.8660254037844387076, 1.000000000000000000, 0.8660254037844387076, 1.000000000000000000, 0.8660254037844387076, 1.000000000000000000, 0.8660254037844387076, 1.000000000000000000, 0.8660254037844387076, 1.000000000000000000, 0.8660254037844387076, 1.000000000000000000, 0.8660254037844387076, 1.000000000000000000, 0.8660254037844387076, 1.000000000000000000, 0.8660254037844387076, 1.000000000000000000, 0.8660254037844387076, 1.000000000000000000, 0.8660254037844387076, 1.000000000000000000, 0.8660254037844387076, 1.000000000000000000, 0.8660254037844387076, 1.000000000000000000, 0.8660254037844387076, 1.000000000000000000, 0.8660254037844387076, 1.000000000000000000, 0.8660254037844387076, 1.000000000000000000, 0.8660254037844387076, 1.000000000000000000, 0.8660254037844387076, 1.000000000000000000, 0.8660254037844387076, 1.000000000000000000, 0.8660254037844387076, 1.000000000000000000, 0.8660254037844387076, 1.000000000000000000, 0.8660254037844387076, 1.000000000000000000, 0.8660254037844387076, 1.000000000000000000, 0.8660254037844387076, 1.000000000000000000, 0.8660254037844387076, 1.000000000000000000, 0.8660254037844387076, 1.000000000000000000, 0.8660254037844387076, 1.000000000000000000, 0.8660254037844387076, 1.000000000000000000, 0.8660254037844387076, 1.000000000000000000, 0.8957441496011343540, 0.9537471549767215784 ) ) 
 REPRESENTATION_ITEM ( '' )  );
#14761=CARTESIAN_POINT ( 'NONE',  ( 233.9782151781249411, -30.44062499938548072, 102.3871387122750889 ) ) ;
#14765=CARTESIAN_POINT ( 'NONE',  ( 232.5999999999999375, -33.93749999999999289, 103.0000000000000000 ) ) ;
#14770=CARTESIAN_POINT ( 'NONE',  ( 229.8435696437499303, -33.29062499938547148, -50.00000000000011369 ) ) ;
#14771=ORIENTED_EDGE ( 'NONE', *, *, #8320, .T. ) ;
#14772=EDGE_LOOP ( 'NONE', ( #17345, #5868, #10310, #476 ) ) ;
#14777=EDGE_CURVE ( 'NONE', #1022, #15818, #15388, .T. ) ;
#14780=CARTESIAN_POINT ( 'NONE',  ( 231.2217848218749339, -32.31562499938547717, 102.3871387122750889 ) ) ;
#14781=CARTESIAN_POINT ( 'NONE',  ( 231.2217848218749339, -34.26562499938548001, -52.38713871227520968 ) ) ;
#14785=CARTESIAN_POINT ( 'NONE',  ( 234.0999999999999375, -30.14999999999999503, -52.59807621135342970 ) ) ;
#14788=ORIENTED_EDGE ( 'NONE', *, *, #4540, .F. ) ;
#14790=CYLINDRICAL_SURFACE ( 'NONE', #11791, 3.000000000000002665 ) ;
#14791=CARTESIAN_POINT ( 'NONE',  ( 232.5999999999999375, -31.04062499938547859, -46.81714838363331666 ) ) ;
#14793=EDGE_LOOP ( 'NONE', ( #13380, #13246, #10632, #11905, #16715, #14707, #7628, #4708, #1082, #9459, #12205, #7924, #7296, #18200, #243, #12108, #3864 ) ) ;
#14804=CARTESIAN_POINT ( 'NONE',  ( 231.0999999999999375, -33.07499999999999574, -47.40192378864679768 ) ) ;
#14810=CARTESIAN_POINT ( 'NONE',  ( 231.2217848218749339, -34.82812499938548001, -52.38713871227520968 ) ) ;
#14816=LINE ( 'NONE', #16490, #1929 ) ;
#14817=CARTESIAN_POINT ( 'NONE',  ( 232.5999999999999375, -33.71249999999999147, -53.00000000000010658 ) ) ;
#14819=DIRECTION ( 'NONE',  ( -0.000000000000000000, -1.000000000000000000, 3.597944987211154374E-15 ) ) ;
#14821=CARTESIAN_POINT ( 'NONE',  ( 229.8435696437499871, -32.99062499938548143, 98.40857419181659793 ) ) ;
#14826=DIRECTION ( 'NONE',  ( -1.000000000000000000, 0.000000000000000000, 0.000000000000000000 ) ) ;
#14830=CARTESIAN_POINT ( 'NONE',  ( 231.0999999999999375, -32.77499999999999147, 97.40192378864668399 ) ) ;
#14831=EDGE_CURVE ( 'NONE', #1510, #14649, #8717, .T. ) ;
#14835=CARTESIAN_POINT ( 'NONE',  ( 231.2217848218749339, -30.77812499938548285, 97.61286128772489690 ) ) ;
#14836=CARTESIAN_POINT ( 'NONE',  ( 235.5999999999999375, -34.66874999877096286, -50.00000000000011369 ) ) ;
#14842=FACE_OUTER_BOUND ( 'NONE', #15213, .T. ) ;
#14843=CARTESIAN_POINT ( 'NONE',  ( 234.0999999999999375, -34.19999999999999574, -52.59807621135342970 ) ) ;
#14846=FACE_OUTER_BOUND ( 'NONE', #18577, .T. ) ;
#14847=EDGE_CURVE ( 'NONE', #6709, #3185, #5857, .T. ) ;
#14856=VECTOR ( 'NONE', #16517, 1000.000000000000000 ) ;
#14857=DIRECTION ( 'NONE',  ( -0.000000000000000000, -0.000000000000000000, 1.000000000000000000 ) ) ;
#14861=CARTESIAN_POINT ( 'NONE',  ( 235.5999999999999375, -32.47499999999999432, -50.00000000000011369 ) ) ;
#14863=DIRECTION ( 'NONE',  ( -1.000000000000000000, 4.625929269271485791E-17, -5.836151346627967635E-31 ) ) ;
#14866=CARTESIAN_POINT ( 'NONE',  ( 229.8435696437499871, -33.25312499938547717, -48.40857419181671162 ) ) ;
#14875=CARTESIAN_POINT ( 'NONE',  ( 235.3564303562499447, -33.51562499938548001, 99.99999999999998579 ) ) ;
#14877=CARTESIAN_POINT ( 'NONE',  ( 233.9782151781249411, -33.59062499938547575, -47.61286128772501769 ) ) ;
#14881=ORIENTED_EDGE ( 'NONE', *, *, #16870, .F. ) ;
#14882=CARTESIAN_POINT ( 'NONE',  ( 229.5999999999999375, -30.44999999999999574, -50.00000000000011369 ) ) ;
#14883=LINE ( 'NONE', #13423, #1649 ) ;
#14885=AXIS2_PLACEMENT_3D ( 'NONE', #15612, #578, #6532 ) ;
#14894=CARTESIAN_POINT ( 'NONE',  ( 235.3564303562499447, -33.96562499938547575, 99.99999999999998579 ) ) ;
#14898=COLOUR_RGB ( '',0.8941176470588234615, 0.8941176470588234615, 0.8941176470588234615 ) ;
#14900=B_SPLINE_CURVE_WITH_KNOTS ( 'NONE', 3,
 ( #14617, #12778, #3981, #9947, #869, #5741, #1248, #6834, #2509, #8466, #14423, #19123, #3883, #17659, #9847, #4271 ),
 .UNSPECIFIED., .F., .F.,
 ( 4, 2, 2, 2, 2, 2, 2, 4 ),
 ( 0.000000000000000000, 0.0005391024520903885250, 0.001078204904180777050, 0.002156409808361623923, 0.002695512260452052021, 0.003234614712542480553, 0.003773717164632909085, 0.004312819616723337184 ),
 .UNSPECIFIED. ) ;
#14903=CARTESIAN_POINT ( 'NONE',  ( 229.8966310988167550, -35.00000000000000711, 100.9939266215705089 ) ) ;
#14913=CARTESIAN_POINT ( 'NONE',  ( 229.8435696437499871, -34.71562499938548285, -48.40857419181671162 ) ) ;
#14925=CARTESIAN_POINT ( 'NONE',  ( 231.7961524227065979, -33.45134618820330275, -47.00000000000012079 ) ) ;
#14927=CARTESIAN_POINT ( 'NONE',  ( 231.2217848218749339, -32.42812499938548143, 102.3871387122750889 ) ) ;
#14936=CARTESIAN_POINT ( 'NONE',  ( 234.0999999999999375, -32.54999999999999716, 102.5980762113533018 ) ) ;
#14937=ORIENTED_EDGE ( 'NONE', *, *, #15830, .F. ) ;
#14938=CARTESIAN_POINT ( 'NONE',  ( 235.3564303562499447, -34.07812499938548001, -50.00000000000011369 ) ) ;
#14940=CARTESIAN_POINT ( 'NONE',  ( 231.0999999999999375, -34.36874999877096570, 102.5980762113533018 ) ) ;
#14941=CARTESIAN_POINT ( 'NONE',  ( 231.0999999999999375, -33.16874999877095576, -52.59807621135342970 ) ) ;
#14944=ORIENTED_EDGE ( 'NONE', *, *, #8764, .F. ) ;
#14958=CARTESIAN_POINT ( 'NONE',  ( 229.8435696437499303, -30.59062499938547575, 99.99999999999998579 ) ) ;
#14960=( NAMED_UNIT ( * ) SI_UNIT ( $, .STERADIAN. ) SOLID_ANGLE_UNIT ( ) );
#14966=CARTESIAN_POINT ( 'NONE',  ( 232.5999999999999375, -34.55624999877095860, 97.00000000000000000 ) ) ;
#14969=CARTESIAN_POINT ( 'NONE',  ( 233.9782151781249411, -33.59062499938547575, -47.61286128772501769 ) ) ;
#14971=ORIENTED_EDGE ( 'NONE', *, *, #756, .F. ) ;
#14978=CARTESIAN_POINT ( 'NONE',  ( 233.9782151781249411, -33.14062499938548001, 102.3871387122750889 ) ) ;
#14979=CARTESIAN_POINT ( 'NONE',  ( 229.8435696437499303, -33.29062499938547148, -50.00000000000011369 ) ) ;
#14983=CARTESIAN_POINT ( 'NONE',  ( 235.5999999999999943, -31.16249999999999432, -48.26794919243124582 ) ) ;
#14990=CARTESIAN_POINT ( 'NONE',  ( 229.8435696437499303, -30.25312499938548072, -50.00000000000011369 ) ) ;
#14996=CARTESIAN_POINT ( 'NONE',  ( 229.8435696437499587, -33.77812499938547575, 98.40857419181659793 ) ) ;
#15003=CARTESIAN_POINT ( 'NONE',  ( 229.6880761451935484, -34.99999999999999289, 99.60674545263957214 ) ) ;
#15009=ORIENTED_EDGE ( 'NONE', *, *, #757, .T. ) ;
#15016=ADVANCED_FACE ( 'NONE', ( #7889 ), #4975, .T. ) ;
#15019=LINE ( 'NONE', #12181, #19206 ) ;
#15021=LINE ( 'NONE', #1641, #10496 ) ;
#15022=CARTESIAN_POINT ( 'NONE',  ( 235.3564303562499447, -32.24062499938548143, 98.40857419181659793 ) ) ;
#15030=CARTESIAN_POINT ( 'NONE',  ( 229.5999999999999375, -34.04999999999999716, 99.99999999999998579 ) ) ;
#15031=VERTEX_POINT ( 'NONE', #17071 ) ;
#15032=CARTESIAN_POINT ( 'NONE',  ( 232.5999999999999943, -32.39062499938548001, -46.81714838363331666 ) ) ;
#15033=CARTESIAN_POINT ( 'NONE',  ( 233.9782151781249411, -30.85312499938547859, 97.61286128772489690 ) ) ;
#15034=CARTESIAN_POINT ( 'NONE',  ( 235.5999999999999375, -32.86874999877096570, -50.00000000000011369 ) ) ;
#15044=VECTOR ( 'NONE', #2931, 1000.000000000000000 ) ;
#15048=CARTESIAN_POINT ( 'NONE',  ( 231.0999999999999375, -33.52499999999999147, 102.5980762113533018 ) ) ;
#15050=DIRECTION ( 'NONE',  ( 1.735459783503185124E-31, 3.491481338843133355E-15, 1.000000000000000000 ) ) ;
#15052=CARTESIAN_POINT ( 'NONE',  ( 229.8435696437499871, -31.97812499938548214, 98.40857419181659793 ) ) ;
#15053=ORIENTED_EDGE ( 'NONE', *, *, #18718, .F. ) ;
#15058=CARTESIAN_POINT ( 'NONE',  ( 232.5999999999999375, -34.55624999877095860, -53.00000000000011369 ) ) ;
#15061=CARTESIAN_POINT ( 'NONE',  ( 230.9316747517381430, -35.00000000000000000, -47.74327260034019105 ) ) ;
#15069=DIRECTION ( 'NONE',  ( -0.000000000000000000, 0.000000000000000000, -1.000000000000000000 ) ) ;
#15071=CARTESIAN_POINT ( 'NONE',  ( 229.8435696437499871, -34.60312499938547859, 101.5914258081833879 ) ) ;
#15072=CARTESIAN_POINT ( 'NONE',  ( 231.2217848218749339, -34.56562499938547717, -47.61286128772501769 ) ) ;
#15077=CARTESIAN_POINT ( 'NONE',  ( 231.0999999999999375, -32.62499999999999289, -47.40192378864679768 ) ) ;
#15084=CARTESIAN_POINT ( 'NONE',  ( 233.9782151781249411, -30.55312499938548143, -47.61286128772501769 ) ) ;
#15088=CARTESIAN_POINT ( 'NONE',  ( 232.5999999999999375, -29.99999999999999645, -50.00000000000011369 ) ) ;
#15095=CARTESIAN_POINT ( 'NONE',  ( 235.5999999999999375, -32.02499999999999858, 99.99999999999998579 ) ) ;
#15099=CARTESIAN_POINT ( 'NONE',  ( 235.3564303562499447, -30.36562499938547788, -50.00000000000011369 ) ) ;
#15114=CARTESIAN_POINT ( 'NONE',  ( 235.3564303562499447, -34.49062499938548143, 98.40857419181659793 ) ) ;
#15125=CARTESIAN_POINT ( 'NONE',  ( 234.0999999999999375, -33.89999999999999147, 102.5980762113533018 ) ) ;
#15127=CARTESIAN_POINT ( 'NONE',  ( 232.5999999999999943, -34.19062499938547717, -46.81714838363331666 ) ) ;
#15129=CARTESIAN_POINT ( 'NONE',  ( 229.5999999999999375, -34.48124999877096286, 98.26794919243111792 ) ) ;
#15130=CARTESIAN_POINT ( 'NONE',  ( 234.0999999999999375, -35.19374999877096855, -47.40192378864679768 ) ) ;
#15133=ADVANCED_FACE ( 'NONE', ( #7984 ), #13939, .F. ) ;
#15137=VERTEX_POINT ( 'NONE', #12478 ) ;
#15145=FACE_OUTER_BOUND ( 'NONE', #6471, .T. ) ;
#15146=LINE ( 'NONE', #4897, #8051 ) ;
#15147=CARTESIAN_POINT ( 'NONE',  ( 244.7999999999999545, -29.80000000000002203, 147.7999999999999829 ) ) ;
#15148=CARTESIAN_POINT ( 'NONE',  ( 229.8435696437499871, -31.45312499938547290, 101.5914258081833879 ) ) ;
#15149=ORIENTED_EDGE ( 'NONE', *, *, #14847, .F. ) ;
#15151=CARTESIAN_POINT ( 'NONE',  ( 231.7961524227065695, -32.28615380933862156, 96.99999999999997158 ) ) ;
#15156=CARTESIAN_POINT ( 'NONE',  ( 229.8435696437499871, -34.15312499938547575, -48.40857419181671162 ) ) ;
#15157=EDGE_LOOP ( 'NONE', ( #3108, #6089, #13146, #3014 ) ) ;
#15158=ORIENTED_EDGE ( 'NONE', *, *, #16190, .T. ) ;
#15164=CARTESIAN_POINT ( 'NONE',  ( 233.9782151781249411, -33.59062499938547575, 102.3871387122750889 ) ) ;
#15171=CARTESIAN_POINT ( 'NONE',  ( 229.5999999999999375, -33.63749999999998863, -51.73205080756898866 ) ) ;
#15177=CARTESIAN_POINT ( 'NONE',  ( 235.3564303562499447, -34.11562499938548143, -48.40857419181671162 ) ) ;
#15184=CARTESIAN_POINT ( 'NONE',  ( 230.0213320530828582, -31.99999999999997868, -50.98998077060178247 ) ) ;
#15190=CARTESIAN_POINT ( 'NONE',  ( 235.3564303562499447, -30.40312499938547575, -48.40857419181671162 ) ) ;
#15195=AXIS2_PLACEMENT_3D ( 'NONE', #7921, #9380, #331 ) ;
#15198=EDGE_CURVE ( 'NONE', #18970, #5195, #3984, .T. ) ;
#15203=VECTOR ( 'NONE', #14164, 1000.000000000000000 ) ;
#15208=CARTESIAN_POINT ( 'NONE',  ( 232.5999999999999375, -33.65624999877096002, 97.00000000000000000 ) ) ;
#15209=EDGE_CURVE ( 'NONE', #12222, #7898, #18930, .T. ) ;
#15210=CARTESIAN_POINT ( 'NONE',  ( 232.5999999999999375, -34.64062499938548001, 103.1828516163667899 ) ) ;
#15213=EDGE_LOOP ( 'NONE', ( #7583, #14944, #12738, #18057, #1198, #6568 ) ) ;
#15214=CARTESIAN_POINT ( 'NONE',  ( 232.5999999999999659, -32.58749999999999858, 102.9999999999999858 ) ) ;
#15220=AXIS2_PLACEMENT_3D ( 'NONE', #3225, #6271, #10462 ) ;
#15223=CIRCLE ( 'NONE', #6815, 3.000000000000002665 ) ;
#15225=CARTESIAN_POINT ( 'NONE',  ( 235.3564303562499447, -33.14062499938548001, -51.59142580818350154 ) ) ;
#15227=CARTESIAN_POINT ( 'NONE',  ( 229.5999999999999375, -35.34374999877096002, 99.99999999999998579 ) ) ;
#15228=CARTESIAN_POINT ( 'NONE',  ( 231.2217848218749339, -30.77812499938548285, -52.38713871227520968 ) ) ;
#15230=VECTOR ( 'NONE', #12199, 1000.000000000000000 ) ;
#15232=VERTEX_POINT ( 'NONE', #17652 ) ;
#15234=DIRECTION ( 'NONE',  ( 0.000000000000000000, 0.000000000000000000, 1.000000000000000000 ) ) ;
#15238=CARTESIAN_POINT ( 'NONE',  ( 231.0999999999999375, -33.91874999877096286, 102.5980762113533018 ) ) ;
#15248=CARTESIAN_POINT ( 'NONE',  ( 231.2217848218749339, -35.01562499938548001, 102.3871387122750889 ) ) ;
#15249=CARTESIAN_POINT ( 'NONE',  ( 231.2217848218749339, -31.41562499938547859, 102.3871387122750889 ) ) ;
#15255=DIRECTION ( 'NONE',  ( 0.000000000000000000, -1.000000000000000000, 0.000000000000000000 ) ) ;
#15256=CARTESIAN_POINT ( 'NONE',  ( 229.7064227204516556, -35.00000000000002132, -49.68450386720867584 ) ) ;
#15265=CARTESIAN_POINT ( 'NONE',  ( 232.5999999999999375, -33.85312499938547859, 96.81714838363319586 ) ) ;
#15270=( BOUNDED_CURVE ( )  B_SPLINE_CURVE ( 2, ( #16230, #5771, #14843, #7326, #4204, #16322, #4110, #10073, #19254 ),
 .UNSPECIFIED., .F., .F. ) 
 B_SPLINE_CURVE_WITH_KNOTS ( ( 3, 2, 2, 2, 3 ),
 ( 0.7708333333333332593, 0.7777777777777777901, 0.7916666666666666297, 0.8055555555555555802, 0.8125000000000000000 ),
 .UNSPECIFIED. ) 
 CURVE ( )  GEOMETRIC_REPRESENTATION_ITEM ( )  RATIONAL_B_SPLINE_CURVE ( ( 0.9330127018922192983, 0.9330127018922187432, 1.000000000000000000, 0.8660254037844387076, 1.000000000000000000, 0.8660254037844387076, 1.000000000000000000, 0.9330127018922194093, 0.9330127018922194093 ) ) 
 REPRESENTATION_ITEM ( '' )  );
#15271=CARTESIAN_POINT ( 'NONE',  ( 235.5999999999999375, -32.92499999999999716, -50.00000000000011369 ) ) ;
#15275=CARTESIAN_POINT ( 'NONE',  ( 230.5523683116323355, -32.00000000000000000, 101.8452947671440540 ) ) ;
#15277=CARTESIAN_POINT ( 'NONE',  ( 231.2217848218749339, -34.37812499938547717, -52.38713871227520968 ) ) ;
#15281=CARTESIAN_POINT ( 'NONE',  ( 231.2217848218749339, -34.26562499938548001, 97.61286128772489690 ) ) ;
#15283=CARTESIAN_POINT ( 'NONE',  ( 229.9620029755564588, -32.00000000000001421, -50.81878454495714692 ) ) ;
#15285=DIRECTION ( 'NONE',  ( 0.000000000000000000, 1.000000000000000000, 0.000000000000000000 ) ) ;
#15288=CARTESIAN_POINT ( 'NONE',  ( 235.5999999999999943, -32.88749999999999574, -51.73205080756900287 ) ) ;
#15304=CARTESIAN_POINT ( 'NONE',  ( 232.5999999999999375, -32.98124999877095576, -47.00000000000011369 ) ) ;
#15305=CARTESIAN_POINT ( 'NONE',  ( 235.3564303562499447, -34.04062499938547859, 98.40857419181659793 ) ) ;
#15308=CARTESIAN_POINT ( 'NONE',  ( 232.5999999999999375, -33.26249999999999574, -53.00000000000011369 ) ) ;
#15310=CARTESIAN_POINT ( 'NONE',  ( 229.8787539177868098, -32.00000000000000000, 99.52644304241978546 ) ) ;
#15316=CARTESIAN_POINT ( 'NONE',  ( 235.3564303562499447, -32.69062499938547717, -51.59142580818350154 ) ) ;
#15318=CARTESIAN_POINT ( 'NONE',  ( 229.8435696437499871, -32.54062499938547859, 98.40857419181659793 ) ) ;
#15319=CARTESIAN_POINT ( 'NONE',  ( 232.5999999999999375, -30.36562499938548498, -53.18285161636690361 ) ) ;
#15320=ADVANCED_FACE ( 'NONE', ( #2310 ), #17270, .F. ) ;
#15323=EDGE_LOOP ( 'NONE', ( #6343, #10845, #1811, #904 ) ) ;
#15333=DIRECTION ( 'NONE',  ( -4.625929269271485791E-17, -1.000000000000000000, 0.000000000000000000 ) ) ;
#15335=EDGE_CURVE ( 'NONE', #18607, #15232, #14224, .T. ) ;
#15336=CARTESIAN_POINT ( 'NONE',  ( 234.0999999999999375, -32.49374999877096570, 102.5980762113533018 ) ) ;
#15339=CARTESIAN_POINT ( 'NONE',  ( 230.4884450829329694, -35.14114833091483803, 98.22820877610629964 ) ) ;
#15340=EDGE_CURVE ( 'NONE', #138, #12892, #16082, .T. ) ;
#15345=VERTEX_POINT ( 'NONE', #8460 ) ;
#15360=CARTESIAN_POINT ( 'NONE',  ( 229.5999999999999375, -33.11249999999999716, 101.7320508075688821 ) ) ;
#15365=AXIS2_PLACEMENT_3D ( 'NONE', #17784, #11713, #8689 ) ;
#15368=CARTESIAN_POINT ( 'NONE',  ( 235.5999999999999943, -32.06249999999999289, -48.26794919243124582 ) ) ;
#15372=CARTESIAN_POINT ( 'NONE',  ( 232.5999999999999943, -33.06562499938547717, 96.81714838363319586 ) ) ;
#15374=CARTESIAN_POINT ( 'NONE',  ( 229.8435696437499303, -33.40312499938547575, -50.00000000000011369 ) ) ;
#15376=ORIENTED_EDGE ( 'NONE', *, *, #3904, .F. ) ;
#15378=EDGE_CURVE ( 'NONE', #3413, #5719, #7287, .T. ) ;
#15388=B_SPLINE_CURVE_WITH_KNOTS ( 'NONE', 3,
 ( #12889, #1072, #19046, #14730, #5670, #6849, #12983, #983, #18860, #7030, #18954, #5578, #4095, #11613, #17580, #4191 ),
 .UNSPECIFIED., .F., .F.,
 ( 4, 2, 2, 2, 2, 2, 2, 4 ),
 ( 0.000000000000000000, 0.0005391024520904045712, 0.001078204904180809142, 0.002156409808361649943, 0.002695512260452069802, 0.003234614712542490094, 0.003773717164632910820, 0.004312819616723331112 ),
 .UNSPECIFIED. ) ;
#15393=( BOUNDED_SURFACE ( )  B_SPLINE_SURFACE ( 1, 2, ( 
 ( #7025, #18662, #979, #12979, #2331, #6934, #5573, #10052, #10147, #16011, #8202, #6045, #1449, #14724, #19235, #3097, #16495, #8864, #12088, #10429, #16211, #4673, #6138, #10249, #14629, #8676, #2817, #7595, #8774, #10527, #17865, #4284, #5753, #13457, #1642, #11992, #92, #1360, #11894, #4381, #13548, #19136, #4476, #18062, #9057, #3003, #16393, #7304, #13261, #10622, #2716, #17960, #4570, #15022, #8959, #1264, #188, #7211, #14927, #13164, #1774, #11702, #13365, #17671, #2912, #5851, #11805, #17774, #10338, #1553, #7501, #7402, #16302, #14821, #5947, #3578, #18345, #12284, #9439, #9538, #15405, #570, #16588, #7688, #668, #13644, #4967, #12184, #6332, #1918, #3192, #3391, #10909, #285, #7787, #4774, #2015, #18534, #6236, #12566, #6525, #15305, #9246, #13741, #16967, #11000, #9342, #6617, #16875, #10717, #5150, #9151, #16681, #15114, #1730, #3287, #2119, #15210, #5058, #12379, #18152, #1827, #7975, #15504, #12471, #13931, #379, #6423, #18248, #4866, #10810, #13832, #18439, #16776, #474 ),
 ( #7881, #3479, #8079, #14032, #7170, #2663, #4047, #17726, #8530, #17528, #2770, #14480, #5620, #14678, #15606, #761, #11565, #13216, #17623, #18633, #11096, #19187, #4238, #1110, #17166, #6714, #1313, #2865, #16059, #16256, #11659, #13028, #8823, #8176, #1213, #1406, #5803, #10195, #13119, #11200, #10006, #19290, #7358, #8725, #7261, #4336, #19090, #13315, #11755, #17065, #16159, #3680, #8624, #9645, #14577, #14123, #4140, #10296, #14780, #15961, #2212, #12660, #5254, #10103, #2568, #5711, #7069, #18999, #7642, #1601, #18113, #18208, #4727, #9201, #5904, #16349, #9301, #2960, #13597, #1505, #14978, #10583, #11850, #12042, #238, #8914, #16446, #13414, #10670, #7839, #14875, #1880, #15164, #4630, #17917, #3056, #6290, #343, #18018, #15265, #6196, #44, #13793, #17818, #5995, #4428, #10388, #11947, #10766, #4524, #13703, #1691, #7456, #10482, #16640, #4826, #1782, #3243, #9018, #15071, #7548, #13507, #145, #3147, #7746, #6095, #9107, #12144, #12239, #16548, #16731, #3340, #5208, #14180, #3730 ) ),
 .UNSPECIFIED., .F., .F., .F. ) 
 B_SPLINE_SURFACE_WITH_KNOTS ( ( 2, 2 ),
 ( 3, 2, 2, 2, 2, 2, 2, 2, 2, 2, 2, 2, 2, 2, 2, 2, 2, 2, 2, 2, 2, 2, 2, 2, 2, 2, 2, 2, 2, 2, 2, 2, 2, 2, 2, 2, 2, 2, 2, 2, 2, 2, 2, 2, 2, 2, 2, 2, 2, 2, 2, 2, 2, 2, 2, 2, 2, 2, 2, 2, 2, 2, 2, 2, 2, 2, 2, 3 ),
 ( 0.000000000000000000, 1.000000000000000000 ),
 ( 0.000000000000000000, 0.01388888888888888812, 0.02777777777777777624, 0.04166666666666666435, 0.05555555555555555247, 0.06944444444444444753, 0.08333333333333332871, 0.09722222222222222376, 0.1111111111111111049, 0.1250000000000000000, 0.1388888888888888951, 0.1527777777777777901, 0.1666666666666666574, 0.1805555555555555525, 0.1944444444444444475, 0.2083333333333333426, 0.2222222222222222099, 0.2361111111111111049, 0.2500000000000000000, 0.2638888888888888951, 0.2777777777777777901, 0.2916666666666666852, 0.3055555555555555802, 0.3194444444444444198, 0.3333333333333333148, 0.3472222222222222099, 0.3611111111111111049, 0.3750000000000000000, 0.3888888888888888951, 0.4027777777777777901, 0.4166666666666666852, 0.4305555555555555802, 0.4444444444444444198, 0.4583333333333333148, 0.4722222222222222099, 0.4861111111111111049, 0.5000000000000000000, 0.5138888888888888395, 0.5277777777777777901, 0.5416666666666666297, 0.5555555555555555802, 0.5694444444444444198, 0.5833333333333333703, 0.5972222222222222099, 0.6111111111111111605, 0.6250000000000000000, 0.6388888888888888395, 0.6527777777777777901, 0.6666666666666666297, 0.6805555555555555802, 0.6944444444444444198, 0.7083333333333333703, 0.7222222222222222099, 0.7361111111111111605, 0.7500000000000000000, 0.7638888888888888395, 0.7777777777777777901, 0.7916666666666666297, 0.8055555555555555802, 0.8194444444444444198, 0.8333333333333333703, 0.8472222222222222099, 0.8611111111111111605, 0.8750000000000000000, 0.8888888888888888395, 0.9027777777777777901, 0.9166666666666666297, 0.9258785565094813652 ),
 .UNSPECIFIED. ) 
 GEOMETRIC_REPRESENTATION_ITEM ( )  RATIONAL_B_SPLINE_SURFACE ( (
 ( 1.000000000000000000, 0.8660254037844387076, 1.000000000000000000, 0.8660254037844387076, 1.000000000000000000, 0.8660254037844387076, 1.000000000000000000, 0.8660254037844387076, 1.000000000000000000, 0.8660254037844387076, 1.000000000000000000, 0.8660254037844387076, 1.000000000000000000, 0.8660254037844387076, 1.000000000000000000, 0.8660254037844387076, 1.000000000000000000, 0.8660254037844387076, 1.000000000000000000, 0.8660254037844387076, 1.000000000000000000, 0.8660254037844387076, 1.000000000000000000, 0.8660254037844387076, 1.000000000000000000, 0.8660254037844387076, 1.000000000000000000, 0.8660254037844387076, 1.000000000000000000, 0.8660254037844387076, 1.000000000000000000, 0.8660254037844387076, 1.000000000000000000, 0.8660254037844387076, 1.000000000000000000, 0.8660254037844387076, 1.000000000000000000, 0.8660254037844387076, 1.000000000000000000, 0.8660254037844387076, 1.000000000000000000, 0.8660254037844387076, 1.000000000000000000, 0.8660254037844387076, 1.000000000000000000, 0.8660254037844387076, 1.000000000000000000, 0.8660254037844387076, 1.000000000000000000, 0.8660254037844387076, 1.000000000000000000, 0.8660254037844387076, 1.000000000000000000, 0.8660254037844387076, 1.000000000000000000, 0.8660254037844387076, 1.000000000000000000, 0.8660254037844387076, 1.000000000000000000, 0.8660254037844387076, 1.000000000000000000, 0.8660254037844387076, 1.000000000000000000, 0.8660254037844387076, 1.000000000000000000, 0.8660254037844387076, 1.000000000000000000, 0.8660254037844387076, 1.000000000000000000, 0.8660254037844387076, 1.000000000000000000, 0.8660254037844387076, 1.000000000000000000, 0.8660254037844387076, 1.000000000000000000, 0.8660254037844387076, 1.000000000000000000, 0.8660254037844387076, 1.000000000000000000, 0.8660254037844387076, 1.000000000000000000, 0.8660254037844387076, 1.000000000000000000, 0.8660254037844387076, 1.000000000000000000, 0.8660254037844387076, 1.000000000000000000, 0.8660254037844387076, 1.000000000000000000, 0.8660254037844387076, 1.000000000000000000, 0.8660254037844387076, 1.000000000000000000, 0.8660254037844387076, 1.000000000000000000, 0.8660254037844387076, 1.000000000000000000, 0.8660254037844387076, 1.000000000000000000, 0.8660254037844387076, 1.000000000000000000, 0.8660254037844387076, 1.000000000000000000, 0.8660254037844387076, 1.000000000000000000, 0.8660254037844387076, 1.000000000000000000, 0.8660254037844387076, 1.000000000000000000, 0.8660254037844387076, 1.000000000000000000, 0.8660254037844387076, 1.000000000000000000, 0.8660254037844387076, 1.000000000000000000, 0.8660254037844387076, 1.000000000000000000, 0.8660254037844387076, 1.000000000000000000, 0.8660254037844387076, 1.000000000000000000, 0.8660254037844387076, 1.000000000000000000, 0.8660254037844387076, 1.000000000000000000, 0.8660254037844387076, 1.000000000000000000, 0.8660254037844387076, 1.000000000000000000, 0.8660254037844387076, 1.000000000000000000, 0.8660254037844387076, 1.000000000000000000, 0.9111405360107203144, 0.9401542295229963209),
 ( 1.000000000000000000, 0.8660254037844387076, 1.000000000000000000, 0.8660254037844387076, 1.000000000000000000, 0.8660254037844387076, 1.000000000000000000, 0.8660254037844387076, 1.000000000000000000, 0.8660254037844387076, 1.000000000000000000, 0.8660254037844387076, 1.000000000000000000, 0.8660254037844387076, 1.000000000000000000, 0.8660254037844387076, 1.000000000000000000, 0.8660254037844387076, 1.000000000000000000, 0.8660254037844387076, 1.000000000000000000, 0.8660254037844387076, 1.000000000000000000, 0.8660254037844387076, 1.000000000000000000, 0.8660254037844387076, 1.000000000000000000, 0.8660254037844387076, 1.000000000000000000, 0.8660254037844387076, 1.000000000000000000, 0.8660254037844387076, 1.000000000000000000, 0.8660254037844387076, 1.000000000000000000, 0.8660254037844387076, 1.000000000000000000, 0.8660254037844387076, 1.000000000000000000, 0.8660254037844387076, 1.000000000000000000, 0.8660254037844387076, 1.000000000000000000, 0.8660254037844387076, 1.000000000000000000, 0.8660254037844387076, 1.000000000000000000, 0.8660254037844387076, 1.000000000000000000, 0.8660254037844387076, 1.000000000000000000, 0.8660254037844387076, 1.000000000000000000, 0.8660254037844387076, 1.000000000000000000, 0.8660254037844387076, 1.000000000000000000, 0.8660254037844387076, 1.000000000000000000, 0.8660254037844387076, 1.000000000000000000, 0.8660254037844387076, 1.000000000000000000, 0.8660254037844387076, 1.000000000000000000, 0.8660254037844387076, 1.000000000000000000, 0.8660254037844387076, 1.000000000000000000, 0.8660254037844387076, 1.000000000000000000, 0.8660254037844387076, 1.000000000000000000, 0.8660254037844387076, 1.000000000000000000, 0.8660254037844387076, 1.000000000000000000, 0.8660254037844387076, 1.000000000000000000, 0.8660254037844387076, 1.000000000000000000, 0.8660254037844387076, 1.000000000000000000, 0.8660254037844387076, 1.000000000000000000, 0.8660254037844387076, 1.000000000000000000, 0.8660254037844387076, 1.000000000000000000, 0.8660254037844387076, 1.000000000000000000, 0.8660254037844387076, 1.000000000000000000, 0.8660254037844387076, 1.000000000000000000, 0.8660254037844387076, 1.000000000000000000, 0.8660254037844387076, 1.000000000000000000, 0.8660254037844387076, 1.000000000000000000, 0.8660254037844387076, 1.000000000000000000, 0.8660254037844387076, 1.000000000000000000, 0.8660254037844387076, 1.000000000000000000, 0.8660254037844387076, 1.000000000000000000, 0.8660254037844387076, 1.000000000000000000, 0.8660254037844387076, 1.000000000000000000, 0.8660254037844387076, 1.000000000000000000, 0.8660254037844387076, 1.000000000000000000, 0.8660254037844387076, 1.000000000000000000, 0.8660254037844387076, 1.000000000000000000, 0.8660254037844387076, 1.000000000000000000, 0.8660254037844387076, 1.000000000000000000, 0.8660254037844387076, 1.000000000000000000, 0.8660254037844387076, 1.000000000000000000, 0.8660254037844387076, 1.000000000000000000, 0.8660254037844387076, 1.000000000000000000, 0.9111405360107203144, 0.9401542295229963209) ) ) 
 REPRESENTATION_ITEM ( '' )  SURFACE ( )  );
#15402=CARTESIAN_POINT ( 'NONE',  ( 246.9999999999999716, -35.00000000000000000, 150.0000000000000000 ) ) ;
#15403=DIRECTION ( 'NONE',  ( 0.000000000000000000, 0.000000000000000000, 1.000000000000000000 ) ) ;
#15405=CARTESIAN_POINT ( 'NONE',  ( 233.9782151781249411, -33.25312499938547717, 102.3871387122750889 ) ) ;
#15419=CARTESIAN_POINT ( 'NONE',  ( 229.8435696437499303, -32.05312499938548143, 99.99999999999998579 ) ) ;
#15420=CARTESIAN_POINT ( 'NONE',  ( 232.5999999999999375, -35.23124999877096286, -46.53589838486234953 ) ) ;
#15427=FACE_OUTER_BOUND ( 'NONE', #975, .T. ) ;
#15438=CARTESIAN_POINT ( 'NONE',  ( 232.6092389720418510, -31.99999999999999289, 102.8695224571928719 ) ) ;
#15439=CARTESIAN_POINT ( 'NONE',  ( 232.5999999999999375, -34.75312499938547717, 96.81714838363319586 ) ) ;
#15440=VERTEX_POINT ( 'NONE', #11876 ) ;
#15446=UNCERTAINTY_MEASURE_WITH_UNIT (LENGTH_MEASURE( 1.000000000000000082E-05 ), #7533, 'distance_accuracy_value', 'NONE');
#15451=CIRCLE ( 'NONE', #9859, 2.199999999999993516 ) ;
#15452=VERTEX_POINT ( 'NONE', #16572 ) ;
#15454=ORIENTED_EDGE ( 'NONE', *, *, #13559, .T. ) ;
#15467=VECTOR ( 'NONE', #18712, 1000.000000000000000 ) ;
#15470=CARTESIAN_POINT ( 'NONE',  ( 235.5999999999999943, -31.61249999999999716, -48.26794919243124582 ) ) ;
#15473=CARTESIAN_POINT ( 'NONE',  ( 233.9782151781249411, -33.25312499938547717, 102.3871387122750889 ) ) ;
#15475=CARTESIAN_POINT ( 'NONE',  ( 235.3564303562499447, -32.27812499938548285, -50.00000000000011369 ) ) ;
#15482=CARTESIAN_POINT ( 'NONE',  ( 230.1700715539191719, -31.99999999999998579, -51.31340704031387645 ) ) ;
#15489=CARTESIAN_POINT ( 'NONE',  ( 233.9782151781249411, -30.44062499938548072, -47.61286128772501769 ) ) ;
#15498=ORIENTED_EDGE ( 'NONE', *, *, #12826, .F. ) ;
#15501=CARTESIAN_POINT ( 'NONE',  ( 231.7961524227065695, -34.53615380933862866, -53.00000000000011369 ) ) ;
#15504=CARTESIAN_POINT ( 'NONE',  ( 232.5999999999999375, -34.86562499938548143, 96.81714838363319586 ) ) ;
#15514=CARTESIAN_POINT ( 'NONE',  ( 230.9855258467272563, -35.02670941564509377, 97.25687757881057394 ) ) ;
#15516=CARTESIAN_POINT ( 'NONE',  ( 232.5999999999999943, -34.64062499938548001, -46.81714838363331666 ) ) ;
#15518=CARTESIAN_POINT ( 'NONE',  ( 232.5999999999999375, -33.51562499938548001, 96.81714838363319586 ) ) ;
#15519=CARTESIAN_POINT ( 'NONE',  ( 229.5999999999999375, -34.93124999877095860, -51.73205080756898866 ) ) ;
#15520=AXIS2_PLACEMENT_3D ( 'NONE', #4368, #13444, #11789 ) ;
#15522=CARTESIAN_POINT ( 'NONE',  ( 232.5999999999999375, -34.83749999999999147, -47.00000000000011369 ) ) ;
#15523=ORIENTED_EDGE ( 'NONE', *, *, #111, .T. ) ;
#15538=PLANE ( 'NONE',  #18325 ) ;
#15539=CARTESIAN_POINT ( 'NONE',  ( 234.5796347213265278, -32.00000000000000711, 102.1983759483905772 ) ) ;
#15540=CARTESIAN_POINT ( 'NONE',  ( 232.5999999999999375, -34.52812499938548285, 103.1828516163667899 ) ) ;
#15560=DIRECTION ( 'NONE',  ( 0.000000000000000000, -1.000000000000000000, 0.000000000000000000 ) ) ;
#15566=EDGE_CURVE ( 'NONE', #12940, #17012, #10411, .T. ) ;
#15569=CARTESIAN_POINT ( 'NONE',  ( 234.0999999999999375, -32.04374999877096286, -47.40192378864679768 ) ) ;
#15572=CARTESIAN_POINT ( 'NONE',  ( 231.2217848218749339, -33.02812499938547575, 97.61286128772489690 ) ) ;
#15574=CARTESIAN_POINT ( 'NONE',  ( 233.9782151781249411, -31.19062499938547717, -52.38713871227520968 ) ) ;
#15582=CARTESIAN_POINT ( 'NONE',  ( 230.1427008797911924, -31.99999999999998579, -48.73859666561349968 ) ) ;
#15589=CARTESIAN_POINT ( 'NONE',  ( 235.3564303562499447, -33.51562499938548001, -50.00000000000011369 ) ) ;
#15603=CARTESIAN_POINT ( 'NONE',  ( 231.5800379434388674, -35.00000000000000000, -52.82826157480266005 ) ) ;
#15606=CARTESIAN_POINT ( 'NONE',  ( 231.2217848218749339, -30.66562499938547859, 97.61286128772489690 ) ) ;
#15610=CARTESIAN_POINT ( 'NONE',  ( 249.9999999999999716, -29.80000000000000426, -100.0000000000000000 ) ) ;
#15612=CARTESIAN_POINT ( 'NONE',  ( 232.5999999999999375, -29.99999999999999645, 99.99999999999998579 ) ) ;
#15617=CARTESIAN_POINT ( 'NONE',  ( 229.8435696437499303, -31.60312499938548214, 99.99999999999998579 ) ) ;
#15618=EDGE_CURVE ( 'NONE', #7254, #3907, #15661, .T. ) ;
#15619=CARTESIAN_POINT ( 'NONE',  ( 233.9782151781249411, -34.15312499938547575, -47.61286128772501769 ) ) ;
#15635=CARTESIAN_POINT ( 'NONE',  ( 244.7999999999999545, -29.80000000000002203, 147.7999999999999829 ) ) ;
#15637=CARTESIAN_POINT ( 'NONE',  ( 235.3564303562499447, -34.82812499938548001, 98.40857419181659793 ) ) ;
#15642=CARTESIAN_POINT ( 'NONE',  ( 235.5999999999999375, -30.61874999877096215, -50.00000000000011369 ) ) ;
#15644=CARTESIAN_POINT ( 'NONE',  ( 244.7999999999999545, -29.80000000000000426, 150.0000000000000000 ) ) ;
#15656=DIRECTION ( 'NONE',  ( 1.000000000000000000, -9.941108744852765039E-17, 1.788378118793199314E-31 ) ) ;
#15657=FACE_OUTER_BOUND ( 'NONE', #16268, .T. ) ;
#15659=LINE ( 'NONE', #2266, #1814 ) ;
#15661=LINE ( 'NONE', #11160, #17410 ) ;
#15663=LINE ( 'NONE', #2273, #11775 ) ;
#15666=DIRECTION ( 'NONE',  ( 0.000000000000000000, 0.000000000000000000, -1.000000000000000000 ) ) ;
#15669=CARTESIAN_POINT ( 'NONE',  ( 235.3564303562499447, -34.94062499938547717, -51.59142580818350865 ) ) ;
#15686=CARTESIAN_POINT ( 'NONE',  ( 232.5999999999999375, -32.72812499938547859, -46.81714838363331666 ) ) ;
#15690=CARTESIAN_POINT ( 'NONE',  ( 235.5999999999999943, -32.83124999877096428, 98.26794919243110371 ) ) ;
#15694=DIRECTION ( 'NONE',  ( 1.000000000000000000, 0.000000000000000000, -0.000000000000000000 ) ) ;
#15698=CARTESIAN_POINT ( 'NONE',  ( 231.0999999999999375, -34.51874999877096428, -52.59807621135342970 ) ) ;
#15699=CARTESIAN_POINT ( 'NONE',  ( 231.7961524227065695, -34.14240381056765017, -53.00000000000011369 ) ) ;
#15709=CARTESIAN_POINT ( 'NONE',  ( 231.6794753800827777, -34.98323688327302960, -52.93263647803299676 ) ) ;
#15714=CARTESIAN_POINT ( 'NONE',  ( 233.9782151781249411, -33.25312499938547717, 102.3871387122750889 ) ) ;
#15715=CARTESIAN_POINT ( 'NONE',  ( 232.5999999999999375, -33.96562499938547575, -53.18285161636690361 ) ) ;
#15717=CARTESIAN_POINT ( 'NONE',  ( 231.0999999999999375, -32.62499999999999289, -47.40192378864679768 ) ) ;
#15720=PLANE ( 'NONE',  #13479 ) ;
#15731=CARTESIAN_POINT ( 'NONE',  ( 232.8441546701661480, -32.00000000000000000, 102.8696726379688755 ) ) ;
#15732=CARTESIAN_POINT ( 'NONE',  ( 229.5999999999999375, -30.44999999999999574, 99.99999999999998579 ) ) ;
#15737=CARTESIAN_POINT ( 'NONE',  ( 232.5999999999999375, -30.73124999877096286, 103.4641016151377499 ) ) ;
#15744=CARTESIAN_POINT ( 'NONE',  ( 231.0999999999999375, -33.61874999877096570, 97.40192378864668399 ) ) ;
#15746=EDGE_LOOP ( 'NONE', ( #15814, #16969, #17583, #7040 ) ) ;
#15747=DIRECTION ( 'NONE',  ( 1.000000000000000000, 0.000000000000000000, 0.000000000000000000 ) ) ;
#15749=CARTESIAN_POINT ( 'NONE',  ( 105.2000000000000739, -32.00000000000002842, 147.7999999999999829 ) ) ;
#15757=DIRECTION ( 'NONE',  ( 1.000000000000000000, 0.000000000000000000, 0.000000000000000000 ) ) ;
#15759=CARTESIAN_POINT ( 'NONE',  ( 235.5999999999999943, -33.86249999999999716, -48.26794919243124582 ) ) ;
#15760=CARTESIAN_POINT ( 'NONE',  ( 234.5119179762161536, -35.00000000000002132, 97.80480077079613466 ) ) ;
#15763=CARTESIAN_POINT ( 'NONE',  ( 229.8435696437499587, -34.71562499938547575, 101.5914258081833879 ) ) ;
#15765=CARTESIAN_POINT ( 'NONE',  ( 235.3564303562499447, -31.26562499938547646, -50.00000000000011369 ) ) ;
#15772=AXIS2_PLACEMENT_3D ( 'NONE', #495, #9175, #13957 ) ;
#15773=LINE ( 'NONE', #15874, #15467 ) ;
#15778=CARTESIAN_POINT ( 'NONE',  ( 231.2217848218749339, -32.31562499938547717, -47.61286128772501769 ) ) ;
#15781=VERTEX_POINT ( 'NONE', #14374 ) ;
#15789=CARTESIAN_POINT ( 'NONE',  ( 244.7999999999999545, -29.80000000000000426, 150.0000000000000000 ) ) ;
#15792=EDGE_CURVE ( 'NONE', #5767, #11694, #3047, .T. ) ;
#15794=CARTESIAN_POINT ( 'NONE',  ( 231.0999999999999375, -33.97500000000000142, -47.40192378864679768 ) ) ;
#15797=DIRECTION ( 'NONE',  ( 0.000000000000000000, 0.000000000000000000, 1.000000000000000000 ) ) ;
#15802=VECTOR ( 'NONE', #5775, 1000.000000000000000 ) ;
#15804=DIRECTION ( 'NONE',  ( -0.000000000000000000, -1.000000000000000000, -0.000000000000000000 ) ) ;
#15809=CARTESIAN_POINT ( 'NONE',  ( 229.8435696437499587, -34.79062499938547859, -51.59142580818350154 ) ) ;
#15810=CARTESIAN_POINT ( 'NONE',  ( 231.2217848218749339, -34.22812499938548569, 102.3871387122750889 ) ) ;
#15811=CARTESIAN_POINT ( 'NONE',  ( 231.2217848218749339, -32.87812499938547717, -47.61286128772501769 ) ) ;
#15814=ORIENTED_EDGE ( 'NONE', *, *, #9832, .F. ) ;
#15816=CARTESIAN_POINT ( 'NONE',  ( 105.1999999999999886, -4.999999999999993783, -103.0000000000000995 ) ) ;
#15818=VERTEX_POINT ( 'NONE', #4218 ) ;
#15827=CARTESIAN_POINT ( 'NONE',  ( 231.4702054326072016, -32.00000000000000711, 102.5803447510189699 ) ) ;
#15829=CARTESIAN_POINT ( 'NONE',  ( 232.5999999999999375, -31.23749999999999361, 103.4641016151377499 ) ) ;
#15830=EDGE_CURVE ( 'NONE', #18941, #6967, #3983, .T. ) ;
#15833=CARTESIAN_POINT ( 'NONE',  ( 232.5999999999999375, -32.98124999877096286, 103.4641016151377499 ) ) ;
#15834=CARTESIAN_POINT ( 'NONE',  ( 229.5999999999999375, -30.84374999877096357, -50.00000000000011369 ) ) ;
#15835=EDGE_LOOP ( 'NONE', ( #13281, #17177, #11464, #12647 ) ) ;
#15842=CARTESIAN_POINT ( 'NONE',  ( 232.5999999999999375, -32.00000000000000000, -50.00000000000011369 ) ) ;
#15846=LINE ( 'NONE', #19161, #15802 ) ;
#15852=CARTESIAN_POINT ( 'NONE',  ( 235.3995413886006247, -34.99999999999998579, -50.31174157908983346 ) ) ;
#15854=CARTESIAN_POINT ( 'NONE',  ( 244.7999999999999545, -32.00000000000002842, 147.7999999999999829 ) ) ;
#15859=ORIENTED_EDGE ( 'NONE', *, *, #9014, .T. ) ;
#15860=CARTESIAN_POINT ( 'NONE',  ( 232.8256241621687366, -34.99999999999999289, 97.01974242045224628 ) ) ;
#15863=CARTESIAN_POINT ( 'NONE',  ( 235.3564303562499447, -33.66562499938548569, 101.5914258081833879 ) ) ;
#15865=CARTESIAN_POINT ( 'NONE',  ( 233.9782151781249411, -30.89062499938548001, -47.61286128772501769 ) ) ;
#15866=ORIENTED_EDGE ( 'NONE', *, *, #17045, .T. ) ;
#15868=AXIS2_PLACEMENT_3D ( 'NONE', #3383, #3961, #11486 ) ;
#15874=CARTESIAN_POINT ( 'NONE',  ( 102.9999999999999858, -5.200000000000008171, -100.0000000000000000 ) ) ;
#15879=CARTESIAN_POINT ( 'NONE',  ( 232.5999999999999375, -32.27812499938547575, -46.81714838363331666 ) ) ;
#15889=CARTESIAN_POINT ( 'NONE',  ( 105.1999999999999886, -29.80000000000001492, -97.80000000000002558 ) ) ;
#15894=DIRECTION ( 'NONE',  ( -0.000000000000000000, -1.000000000000000000, -0.000000000000000000 ) ) ;
#15895=ADVANCED_FACE ( 'NONE', ( #4411 ), #6103, .F. ) ;
#15896=CARTESIAN_POINT ( 'NONE',  ( 234.9223452063436355, -31.99999999999999289, 98.15128725331840087 ) ) ;
#15897=DIRECTION ( 'NONE',  ( -1.000000000000000000, -0.000000000000000000, -0.000000000000000000 ) ) ;
#15900=VERTEX_POINT ( 'NONE', #12576 ) ;
#15904=CARTESIAN_POINT ( 'NONE',  ( 229.8435696437499871, -34.26562499938548001, 101.5914258081833879 ) ) ;
#15905=CARTESIAN_POINT ( 'NONE',  ( 233.9782151781249411, -33.10312499938547859, -52.38713871227520968 ) ) ;
#15908=ORIENTED_EDGE ( 'NONE', *, *, #18718, .T. ) ;
#15920=PRODUCT_DEFINITION_SHAPE ( 'NONE', 'NONE',  #18016 ) ;
#15923=CARTESIAN_POINT ( 'NONE',  ( 231.0999999999999375, -31.87499999999999289, 97.40192378864668399 ) ) ;
#15924=ADVANCED_FACE ( 'NONE', ( #676 ), #1836, .F. ) ;
#15926=CARTESIAN_POINT ( 'NONE',  ( 235.5999999999999375, -34.66874999877096286, 99.99999999999998579 ) ) ;
#15927=CARTESIAN_POINT ( 'NONE',  ( 234.0999999999999375, -32.04374999877096286, 102.5980762113533018 ) ) ;
#15928=CARTESIAN_POINT ( 'NONE',  ( 229.5999999999999375, -31.25624999877096144, -48.26794919243123161 ) ) ;
#15939=EDGE_CURVE ( 'NONE', #8256, #10239, #16689, .T. ) ;
#15945=CARTESIAN_POINT ( 'NONE',  ( 232.5999999999999375, -32.30624999877096570, -53.00000000000011369 ) ) ;
#15949=VERTEX_POINT ( 'NONE', #2024 ) ;
#15950=CARTESIAN_POINT ( 'NONE',  ( 229.5999999999999375, -34.04999999999999716, -50.00000000000011369 ) ) ;
#15955=CARTESIAN_POINT ( 'NONE',  ( 235.3564303562499447, -34.52812499938547575, -50.00000000000011369 ) ) ;
#15961=CARTESIAN_POINT ( 'NONE',  ( 229.8435696437499871, -32.35312499938547859, 101.5914258081833879 ) ) ;
#15962=CARTESIAN_POINT ( 'NONE',  ( 235.3564303562499447, -32.20312499938548001, -48.40857419181671162 ) ) ;
#15970=CARTESIAN_POINT ( 'NONE',  ( 235.3564303562499447, -33.55312499938548143, -48.40857419181671162 ) ) ;
#15975=CARTESIAN_POINT ( 'NONE',  ( 232.5999999999999375, -29.99999999999999645, 103.0000000000000000 ) ) ;
#15981=ORIENTED_EDGE ( 'NONE', *, *, #6542, .T. ) ;
#15983=AXIS2_PLACEMENT_3D ( 'NONE', #10356, #14547, #8699 ) ;
#15984=CYLINDRICAL_SURFACE ( 'NONE', #12855, 3.000000000000002665 ) ;
#15995=VECTOR ( 'NONE', #3923, 1000.000000000000000 ) ;
#15997=ORIENTED_EDGE ( 'NONE', *, *, #15335, .T. ) ;
#15999=CARTESIAN_POINT ( 'NONE',  ( 235.3564303562499447, -34.07812499938548001, 99.99999999999998579 ) ) ;
#16000=CARTESIAN_POINT ( 'NONE',  ( 229.8435696437499871, -33.81562499938547717, -48.40857419181671162 ) ) ;
#16011=CARTESIAN_POINT ( 'NONE',  ( 232.5999999999999375, -30.59062499938547930, 103.1828516163667899 ) ) ;
#16017=CARTESIAN_POINT ( 'NONE',  ( 232.5999999999999375, -29.99999999999999645, 99.99999999999998579 ) ) ;
#16019=CARTESIAN_POINT ( 'NONE',  ( 234.0999999999999375, -30.29999999999999716, 102.5980762113533018 ) ) ;
#16020=ORIENTED_EDGE ( 'NONE', *, *, #9427, .F. ) ;
#16021=CARTESIAN_POINT ( 'NONE',  ( 229.8435696437499587, -32.09062499938548285, -51.59142580818350154 ) ) ;
#16023=CARTESIAN_POINT ( 'NONE',  ( 229.5999999999999375, -33.54374999877096286, 99.99999999999998579 ) ) ;
#16025=LINE ( 'NONE', #8589, #6465 ) ;
#16028=EDGE_LOOP ( 'NONE', ( #7636, #10270, #509, #18424 ) ) ;
#16038=CARTESIAN_POINT ( 'NONE',  ( 235.3058334582606506, -35.00000000000002132, -49.37250936986590943 ) ) ;
#16052=CARTESIAN_POINT ( 'NONE',  ( 231.2217848218749339, -32.76562499938548001, -47.61286128772501769 ) ) ;
#16053=VERTEX_POINT ( 'NONE', #16885 ) ;
#16056=CARTESIAN_POINT ( 'NONE',  ( 246.9999999999999716, -29.80000000000000426, 150.0000000000000000 ) ) ;
#16059=CARTESIAN_POINT ( 'NONE',  ( 233.9782151781249411, -31.19062499938547717, 97.61286128772489690 ) ) ;
#16063=PLANE ( 'NONE',  #8374 ) ;
#16065=CARTESIAN_POINT ( 'NONE',  ( 234.0999999999999375, -30.59999999999999432, -52.59807621135342970 ) ) ;
#16077=CARTESIAN_POINT ( 'NONE',  ( 235.3564303562499447, -33.10312499938547859, 101.5914258081833879 ) ) ;
#16080=( BOUNDED_CURVE ( )  B_SPLINE_CURVE ( 2, ( #8164, #14022, #13731, #1908, #18237, #2006, #12274, #657, #370 ),
 .UNSPECIFIED., .F., .F. ) 
 B_SPLINE_CURVE_WITH_KNOTS ( ( 3, 2, 2, 2, 3 ),
 ( 0.7708333333333332593, 0.7777777777777777901, 0.7916666666666666297, 0.8055555555555555802, 0.8125000000000000000 ),
 .UNSPECIFIED. ) 
 CURVE ( )  GEOMETRIC_REPRESENTATION_ITEM ( )  RATIONAL_B_SPLINE_CURVE ( ( 0.9330127018922192983, 0.9330127018922187432, 1.000000000000000000, 0.8660254037844387076, 1.000000000000000000, 0.8660254037844387076, 1.000000000000000000, 0.9330127018922194093, 0.9330127018922194093 ) ) 
 REPRESENTATION_ITEM ( '' )  );
#16082=B_SPLINE_CURVE_WITH_KNOTS ( 'NONE', 3,
 ( #2694, #6917, #9938, #2407, #16088, #862, #12866, #8652, #12771, #12959, #2596, #8556, #17363, #3972, #15896, #8274, #2502, #7005 ),
 .UNSPECIFIED., .F., .F.,
 ( 4, 2, 2, 2, 2, 2, 2, 2, 4 ),
 ( 0.000000000000000000, 0.0007089252359835998551, 0.001417850471967199710, 0.002126775707950799565, 0.002835700943934399421, 0.003544626179917999276, 0.004253551415901599131, 0.004962476651885198986, 0.005671401887868798841 ),
 .UNSPECIFIED. ) ;
#16085=DIRECTION ( 'NONE',  ( -0.000000000000000000, -1.000000000000000000, -0.000000000000000000 ) ) ;
#16088=CARTESIAN_POINT ( 'NONE',  ( 231.6947747743589616, -31.99999999999999289, 97.33297554273077878 ) ) ;
#16091=CARTESIAN_POINT ( 'NONE',  ( 231.7961524227065695, -33.95759618943232283, 102.9999999999999716 ) ) ;
#16092=CIRCLE ( 'NONE', #4239, 5.200000000000009948 ) ;
#16096=CARTESIAN_POINT ( 'NONE',  ( 235.3564303562499447, -34.49062499938548143, 98.40857419181659793 ) ) ;
#16097=CARTESIAN_POINT ( 'NONE',  ( 231.2217848218749339, -35.12812499938548427, -47.61286128772501769 ) ) ;
#16098=CARTESIAN_POINT ( 'NONE',  ( 244.7999999999999545, -35.00000000000000000, -100.0000000000000000 ) ) ;
#16100=ORIENTED_EDGE ( 'NONE', *, *, #19145, .T. ) ;
#16116=CARTESIAN_POINT ( 'NONE',  ( 229.5999999999999375, -30.03749999999999432, 98.26794919243111792 ) ) ;
#16121=CARTESIAN_POINT ( 'NONE',  ( 235.5999999999999375, -32.86874999877096570, 99.99999999999998579 ) ) ;
#16122=CARTESIAN_POINT ( 'NONE',  ( 234.0999999999999375, -32.49374999877096570, -47.40192378864679768 ) ) ;
#16125=ORIENTED_EDGE ( 'NONE', *, *, #6272, .T. ) ;
#16126=VERTEX_POINT ( 'NONE', #10036 ) ;
#16127=CARTESIAN_POINT ( 'NONE',  ( 105.1999999999999744, -4.999999999999976907, 153.0000000000000000 ) ) ;
#16128=CARTESIAN_POINT ( 'NONE',  ( 244.7999999999999545, -32.00000000000000000, -100.0000000000000000 ) ) ;
#16135=CARTESIAN_POINT ( 'NONE',  ( 234.0999999999999375, -32.49374999877096570, -47.40192378864679768 ) ) ;
#16145=CARTESIAN_POINT ( 'NONE',  ( 235.3564303562499447, -34.94062499938547717, 98.40857419181659793 ) ) ;
#16148=CARTESIAN_POINT ( 'NONE',  ( 229.8435696437499871, -32.42812499938548143, -51.59142580818350865 ) ) ;
#16150=ORIENTED_EDGE ( 'NONE', *, *, #10557, .T. ) ;
#16151=ORIENTED_EDGE ( 'NONE', *, *, #6132, .T. ) ;
#16159=CARTESIAN_POINT ( 'NONE',  ( 231.2217848218749339, -32.01562499938548001, 97.61286128772489690 ) ) ;
#16160=CARTESIAN_POINT ( 'NONE',  ( 229.8435696437499303, -33.74062499938548143, -50.00000000000011369 ) ) ;
#16162=VECTOR ( 'NONE', #11598, 1000.000000000000000 ) ;
#16163=CARTESIAN_POINT ( 'NONE',  ( 244.7999999999999545, -35.00000000000000000, 150.0000000000000000 ) ) ;
#16166=CARTESIAN_POINT ( 'NONE',  ( 230.4884450829329694, -35.14114833091483803, -51.77179122389379984 ) ) ;
#16170=ORIENTED_EDGE ( 'NONE', *, *, #6640, .F. ) ;
#16171=CYLINDRICAL_SURFACE ( 'NONE', #407, 2.199999999999993516 ) ;
#16174=CARTESIAN_POINT ( 'NONE',  ( 231.2217848218749339, -31.52812499938548285, -47.61286128772501769 ) ) ;
#16179=VECTOR ( 'NONE', #13142, 1000.000000000000000 ) ;
#16183=EDGE_CURVE ( 'NONE', #5568, #1884, #14227, .T. ) ;
#16188=DIRECTION ( 'NONE',  ( 1.000000000000000000, -4.625929269271485791E-17, 0.000000000000000000 ) ) ;
#16190=EDGE_CURVE ( 'NONE', #5681, #5198, #12083, .T. ) ;
#16192=CARTESIAN_POINT ( 'NONE',  ( 231.7961524227065695, -34.80134618820329706, 102.9999999999999858 ) ) ;
#16211=CARTESIAN_POINT ( 'NONE',  ( 233.9782151781249411, -31.00312499938548072, 102.3871387122750889 ) ) ;
#16219=CARTESIAN_POINT ( 'NONE',  ( 229.5999999999999375, -33.63749999999998863, 98.26794919243111792 ) ) ;
#16220=ORIENTED_EDGE ( 'NONE', *, *, #47, .T. ) ;
#16223=CARTESIAN_POINT ( 'NONE',  ( 235.5999999999999943, -33.73124999877096286, 98.26794919243110371 ) ) ;
#16224=CARTESIAN_POINT ( 'NONE',  ( 229.5999999999999375, -34.40624999877096002, -48.26794919243123161 ) ) ;
#16230=CARTESIAN_POINT ( 'NONE',  ( 232.5999999999999375, -34.16249999999999432, -53.00000000000010658 ) ) ;
#16232=LINE ( 'NONE', #11917, #8580 ) ;
#16238=CARTESIAN_POINT ( 'NONE',  ( 231.6947747743591037, -31.99999999999998579, -52.66702445726939885 ) ) ;
#16245=FACE_OUTER_BOUND ( 'NONE', #6603, .T. ) ;
#16248=CARTESIAN_POINT ( 'NONE',  ( 231.2217848218749339, -33.36562499938548143, -52.38713871227520968 ) ) ;
#16249=ORIENTED_EDGE ( 'NONE', *, *, #19189, .T. ) ;
#16255=CARTESIAN_POINT ( 'NONE',  ( 105.2000000000000739, -34.99999999999999289, 147.7999999999999829 ) ) ;
#16256=CARTESIAN_POINT ( 'NONE',  ( 235.3564303562499447, -31.22812499938548214, 98.40857419181659793 ) ) ;
#16258=CARTESIAN_POINT ( 'NONE',  ( 229.8435696437499587, -33.70312499938548001, -48.40857419181671162 ) ) ;
#16261=CARTESIAN_POINT ( 'NONE',  ( 229.8435696437499587, -35.11426541925032296, -51.00325264771200295 ) ) ;
#16268=EDGE_LOOP ( 'NONE', ( #17477, #6224, #7155, #13974 ) ) ;
#16271=CARTESIAN_POINT ( 'NONE',  ( 232.5999999999999943, -32.72812499938547859, 103.1828516163667899 ) ) ;
#16274=EDGE_CURVE ( 'NONE', #11529, #11625, #2053, .T. ) ;
#16275=ADVANCED_FACE ( 'NONE', ( #12700 ), #14080, .F. ) ;
#16279=CARTESIAN_POINT ( 'NONE',  ( 234.0999999999999375, -32.09999999999999432, 102.5980762113533018 ) ) ;
#16282=CARTESIAN_POINT ( 'NONE',  ( 232.3466685930879123, -34.99995246259152282, 97.01071553687879145 ) ) ;
#16288=CYLINDRICAL_SURFACE ( 'NONE', #256, 3.000000000000002665 ) ;
#16290=EDGE_CURVE ( 'NONE', #18412, #10068, #14900, .T. ) ;
#16293=VERTEX_POINT ( 'NONE', #1057 ) ;
#16294=EDGE_CURVE ( 'NONE', #6637, #6661, #7012, .T. ) ;
#16300=CARTESIAN_POINT ( 'NONE',  ( 232.5999999999999091, -34.38749999999999574, -47.00000000000011369 ) ) ;
#16302=CARTESIAN_POINT ( 'NONE',  ( 229.8435696437499303, -32.95312499938548001, 99.99999999999998579 ) ) ;
#16311=CARTESIAN_POINT ( 'NONE',  ( 232.5999999999999375, -33.26249999999999574, 96.53589838486223584 ) ) ;
#16313=CARTESIAN_POINT ( 'NONE',  ( 234.0999999999999375, -34.74374999877096570, 102.5980762113533018 ) ) ;
#16314=CARTESIAN_POINT ( 'NONE',  ( 231.2217848218749339, -30.32812499938548001, 97.61286128772489690 ) ) ;
#16315=CARTESIAN_POINT ( 'NONE',  ( 229.5999999999999375, -33.50624999877096144, -48.26794919243123161 ) ) ;
#16320=VECTOR ( 'NONE', #7806, 1000.000000000000000 ) ;
#16322=CARTESIAN_POINT ( 'NONE',  ( 235.5999999999999943, -34.31249999999999289, -48.26794919243124582 ) ) ;
#16325=CARTESIAN_POINT ( 'NONE',  ( 231.7961524227065695, -33.90134618820329138, 103.0000000000000000 ) ) ;
#16329=CARTESIAN_POINT ( 'NONE',  ( 99.99999999999997158, -29.80000000000000071, -100.0000000000000000 ) ) ;
#16333=CARTESIAN_POINT ( 'NONE',  ( 231.2217848218749339, -30.96562499938547930, 102.3871387122750889 ) ) ;
#16334=ORIENTED_EDGE ( 'NONE', *, *, #16290, .T. ) ;
#16337=CARTESIAN_POINT ( 'NONE',  ( 235.5999999999999375, -34.66874999877096286, -50.00000000000011369 ) ) ;
#16338=CARTESIAN_POINT ( 'NONE',  ( 229.5999999999999375, -34.44374999877096144, 99.99999999999998579 ) ) ;
#16341=CARTESIAN_POINT ( 'NONE',  ( 231.2217848218749339, -33.21562499938547575, -47.61286128772501769 ) ) ;
#16349=CARTESIAN_POINT ( 'NONE',  ( 232.5999999999999375, -32.95312499938548001, 96.81714838363319586 ) ) ;
#16350=CARTESIAN_POINT ( 'NONE',  ( 235.3564303562499447, -34.41562499938547859, -50.00000000000011369 ) ) ;
#16355=CARTESIAN_POINT ( 'NONE',  ( 235.3564303562499447, -34.86562499938547433, -50.00000000000011369 ) ) ;
#16361=CARTESIAN_POINT ( 'NONE',  ( 231.2217848218749339, -30.32812499938548001, -52.38713871227520968 ) ) ;
#16364=FACE_OUTER_BOUND ( 'NONE', #4062, .T. ) ;
#16366=( BOUNDED_CURVE ( )  B_SPLINE_CURVE ( 2, ( #10131, #18640, #7914, #13863, #11402, #6721, #12960, #15709, #2311 ),
 .UNSPECIFIED., .F., .F. ) 
 B_SPLINE_CURVE_WITH_KNOTS ( ( 3, 2, 2, 2, 3 ),
 ( 0.8125000000000000000, 0.8194444444444444198, 0.8333333333333333703, 0.8472222222222222099, 0.8530683953269213582 ),
 .UNSPECIFIED. ) 
 CURVE ( )  GEOMETRIC_REPRESENTATION_ITEM ( )  RATIONAL_B_SPLINE_CURVE ( ( 0.9330127018922194093, 0.9330127018922194093, 1.000000000000000000, 0.8660254037844387076, 1.000000000000000000, 0.8660254037844387076, 1.000000000000000000, 0.9436068149601996025, 0.9346881722405915305 ) ) 
 REPRESENTATION_ITEM ( '' )  );
#16367=CARTESIAN_POINT ( 'NONE',  ( 232.5999999999999943, -34.75312499938547717, 96.81714838363319586 ) ) ;
#16381=CARTESIAN_POINT ( 'NONE',  ( 231.2217848218749339, -34.37812499938547717, -52.38713871227520968 ) ) ;
#16393=CARTESIAN_POINT ( 'NONE',  ( 231.2217848218749339, -31.97812499938548214, 102.3871387122750889 ) ) ;
#16400=ADVANCED_FACE ( 'NONE', ( #7489 ), #7390, .F. ) ;
#16403=CARTESIAN_POINT ( 'NONE',  ( 235.5999999999999943, -34.23749999999999716, 98.26794919243110371 ) ) ;
#16405=CARTESIAN_POINT ( 'NONE',  ( 229.8435696437499587, -33.89062499938548001, -51.59142580818350154 ) ) ;
#16406=CARTESIAN_POINT ( 'NONE',  ( 235.5999999999999943, -34.63124999877096144, 98.26794919243110371 ) ) ;
#16407=CARTESIAN_POINT ( 'NONE',  ( 229.5999999999999375, -33.09374999877096002, -50.00000000000011369 ) ) ;
#16408=ADVANCED_FACE ( 'NONE', ( #4558 ), #78, .F. ) ;
#16412=CARTESIAN_POINT ( 'NONE',  ( 99.99999999999997158, -29.80000000000000071, -100.0000000000000000 ) ) ;
#16426=DIRECTION ( 'NONE',  ( 1.000000000000000000, 0.000000000000000000, 0.000000000000000000 ) ) ;
#16427=EDGE_CURVE ( 'NONE', #15137, #8464, #16579, .T. ) ;
#16429=CARTESIAN_POINT ( 'NONE',  ( 235.3564303562499447, -30.40312499938547575, 101.5914258081833879 ) ) ;
#16436=CARTESIAN_POINT ( 'NONE',  ( 232.5999999999999375, -29.99999999999999645, 103.0000000000000000 ) ) ;
#16437=CARTESIAN_POINT ( 'NONE',  ( 233.9782151781249411, -33.44062499938547717, -52.38713871227520968 ) ) ;
#16446=CARTESIAN_POINT ( 'NONE',  ( 231.2217848218749339, -33.36562499938548143, 97.61286128772489690 ) ) ;
#16447=CARTESIAN_POINT ( 'NONE',  ( 231.2217848218749339, -34.71562499938547575, -52.38713871227520968 ) ) ;
#16452=CARTESIAN_POINT ( 'NONE',  ( 235.3564303562499447, -34.90312499938547575, -48.40857419181671162 ) ) ;
#16459=CARTESIAN_POINT ( 'NONE',  ( 235.5999999999999943, -32.90624999877096002, 101.7320508075688537 ) ) ;
#16460=CARTESIAN_POINT ( 'NONE',  ( 231.2217848218749339, -30.77812499938548285, -52.38713871227520968 ) ) ;
#16465=CARTESIAN_POINT ( 'NONE',  ( 232.5999999999999375, -34.33124999877097139, 103.0000000000000000 ) ) ;
#16473=CARTESIAN_POINT ( 'NONE',  ( 229.7512376763114901, -35.00000000000000711, 100.5466586069346278 ) ) ;
#16475=DIRECTION ( 'NONE',  ( 0.000000000000000000, -1.000000000000000000, 0.000000000000000000 ) ) ;
#16482=CARTESIAN_POINT ( 'NONE',  ( 244.7999999999999545, -5.000000000000000888, -103.0000000000000995 ) ) ;
#16483=AXIS2_PLACEMENT_3D ( 'NONE', #1558, #4575, #4289 ) ;
#16485=VECTOR ( 'NONE', #1194, 1000.000000000000000 ) ;
#16488=ORIENTED_EDGE ( 'NONE', *, *, #6489, .T. ) ;
#16490=CARTESIAN_POINT ( 'NONE',  ( 244.7999999999999545, -32.00000000000000000, 150.0000000000000000 ) ) ;
#16493=CARTESIAN_POINT ( 'NONE',  ( 244.7999999999999545, -32.00000000000000000, -100.0000000000000000 ) ) ;
#16495=CARTESIAN_POINT ( 'NONE',  ( 233.9782151781249411, -30.85312499938547859, 97.61286128772489690 ) ) ;
#16499=CARTESIAN_POINT ( 'NONE',  ( 235.5999999999999943, -33.73124999877096286, 98.26794919243110371 ) ) ;
#16501=PLANE ( 'NONE',  #4309 ) ;
#16504=CARTESIAN_POINT ( 'NONE',  ( 234.0999999999999375, -32.99999999999999289, 102.5980762113533018 ) ) ;
#16506=CARTESIAN_POINT ( 'NONE',  ( 229.8435696437499587, -33.81562499938547717, -48.40857419181671162 ) ) ;
#16507=CARTESIAN_POINT ( 'NONE',  ( 229.8435696437499303, -31.15312499938548285, 99.99999999999998579 ) ) ;
#16508=CARTESIAN_POINT ( 'NONE',  ( 229.5999999999999375, -32.64374999877096428, -50.00000000000011369 ) ) ;
#16517=DIRECTION ( 'NONE',  ( -0.000000000000000000, -1.000000000000000000, -0.000000000000000000 ) ) ;
#16518=ADVANCED_FACE ( 'NONE', ( #5838 ), #4463, .F. ) ;
#16528=CARTESIAN_POINT ( 'NONE',  ( 231.2217848218749339, -31.56562499938547717, 97.61286128772489690 ) ) ;
#16530=PRESENTATION_STYLE_ASSIGNMENT (( #18382 ) ) ;
#16532=CARTESIAN_POINT ( 'NONE',  ( 234.0999999999999375, -32.39999999999999858, -52.59807621135342970 ) ) ;
#16538=CARTESIAN_POINT ( 'NONE',  ( 235.3564303562499447, -34.86562499938547433, -50.00000000000011369 ) ) ;
#16547=FACE_OUTER_BOUND ( 'NONE', #8311, .T. ) ;
#16548=CARTESIAN_POINT ( 'NONE',  ( 232.5999999999999375, -34.97812499938547859, 103.1828516163667899 ) ) ;
#16549=CARTESIAN_POINT ( 'NONE',  ( 233.9782151781249411, -34.94062499938547717, -47.61286128772501769 ) ) ;
#16553=CARTESIAN_POINT ( 'NONE',  ( 234.0999999999999375, -32.54999999999999716, -47.40192378864679768 ) ) ;
#16560=ORIENTED_EDGE ( 'NONE', *, *, #19190, .F. ) ;
#16562=CARTESIAN_POINT ( 'NONE',  ( 232.9413037568957066, -34.96883842999723413, 102.9857998004476087 ) ) ;
#16566=ADVANCED_FACE ( 'NONE', ( #464 ), #16958, .F. ) ;
#16568=DIRECTION ( 'NONE',  ( 0.000000000000000000, 0.000000000000000000, 1.000000000000000000 ) ) ;
#16569=CARTESIAN_POINT ( 'NONE',  ( 235.2033360070649906, -32.00000000000000000, -48.51078102784442336 ) ) ;
#16572=CARTESIAN_POINT ( 'NONE',  ( 102.9999999999999858, -5.200000000000008171, 150.0000000000000000 ) ) ;
#16574=CARTESIAN_POINT ( 'NONE',  ( 235.3564303562499447, -31.30312499938547788, -48.40857419181671162 ) ) ;
#16579=LINE ( 'NONE', #12076, #9592 ) ;
#16587=DIRECTION ( 'NONE',  ( 1.000000000000000000, 0.000000000000000000, 0.000000000000000000 ) ) ;
#16588=CARTESIAN_POINT ( 'NONE',  ( 231.2217848218749339, -33.32812499938548001, 102.3871387122750889 ) ) ;
#16591=CARTESIAN_POINT ( 'NONE',  ( 234.0999999999999375, -33.69374999877096144, 97.40192378864668399 ) ) ;
#16596=CARTESIAN_POINT ( 'NONE',  ( 232.5999999999999375, -33.48749999999999716, 103.4641016151377499 ) ) ;
#16599=CARTESIAN_POINT ( 'NONE',  ( 229.8435696437499587, -33.36562499938548143, -48.40857419181671162 ) ) ;
#16601=CARTESIAN_POINT ( 'NONE',  ( 232.5999999999999375, -30.81562499938547717, 96.81714838363319586 ) ) ;
#16602=CARTESIAN_POINT ( 'NONE',  ( 232.5999999999999375, -34.78124999877096002, -46.53589838486234953 ) ) ;
#16609=ORIENTED_EDGE ( 'NONE', *, *, #1112, .T. ) ;
#16612=AXIS2_PLACEMENT_3D ( 'NONE', #3283, #18341, #7683 ) ;
#16618=CARTESIAN_POINT ( 'NONE',  ( 234.0999999999999375, -33.44999999999999574, 102.5980762113533018 ) ) ;
#16621=CARTESIAN_POINT ( 'NONE',  ( 232.5999999999999375, -31.60312499938548214, 96.81714838363319586 ) ) ;
#16624=CARTESIAN_POINT ( 'NONE',  ( 233.4038475772933339, -32.56740381056765443, -47.00000000000012079 ) ) ;
#16629=DIRECTION ( 'NONE',  ( -0.000000000000000000, -1.000000000000000000, -0.000000000000000000 ) ) ;
#16630=CARTESIAN_POINT ( 'NONE',  ( 235.3564303562499447, -34.45312499938548001, -48.40857419181671162 ) ) ;
#16631=EDGE_CURVE ( 'NONE', #5198, #3185, #16080, .T. ) ;
#16633=VERTEX_POINT ( 'NONE', #18524 ) ;
#16634=ORIENTED_EDGE ( 'NONE', *, *, #10313, .T. ) ;
#16640=CARTESIAN_POINT ( 'NONE',  ( 235.3564303562499447, -34.41562499938547859, 99.99999999999998579 ) ) ;
#16646=( BOUNDED_CURVE ( )  B_SPLINE_CURVE ( 2, ( #5495, #11245, #3815, #8498, #11441, #6567, #12515, #18485, #11048 ),
 .UNSPECIFIED., .F., .F. ) 
 B_SPLINE_CURVE_WITH_KNOTS ( ( 3, 2, 2, 2, 3 ),
 ( 0.6041666666666667407, 0.6111111111111111605, 0.6250000000000000000, 0.6388888888888888395, 0.6458333333333331483 ),
 .UNSPECIFIED. ) 
 CURVE ( )  GEOMETRIC_REPRESENTATION_ITEM ( )  RATIONAL_B_SPLINE_CURVE ( ( 0.9330127018922192983, 0.9330127018922198534, 1.000000000000000000, 0.8660254037844387076, 1.000000000000000000, 0.8660254037844387076, 1.000000000000000000, 0.9330127018922209636, 0.9330127018922194093 ) ) 
 REPRESENTATION_ITEM ( '' )  );
#16647=CARTESIAN_POINT ( 'NONE',  ( 231.0999999999999375, -33.52499999999999147, -47.40192378864679768 ) ) ;
#16652=CARTESIAN_POINT ( 'NONE',  ( 229.8435696437499871, -33.81562499938547717, -48.40857419181671162 ) ) ;
#16657=CARTESIAN_POINT ( 'NONE',  ( 235.3564303562499447, -34.86562499938547433, 99.99999999999998579 ) ) ;
#16668=EDGE_LOOP ( 'NONE', ( #11910, #5745, #2051, #6883 ) ) ;
#16675=ORIENTED_EDGE ( 'NONE', *, *, #10187, .F. ) ;
#16679=EDGE_CURVE ( 'NONE', #10996, #7898, #18092, .T. ) ;
#16680=CARTESIAN_POINT ( 'NONE',  ( 244.7999999999999545, -29.80000000000002203, 147.7999999999999829 ) ) ;
#16681=CARTESIAN_POINT ( 'NONE',  ( 233.9782151781249411, -34.45312499938548001, 97.61286128772489690 ) ) ;
#16687=CARTESIAN_POINT ( 'NONE',  ( 234.0999999999999375, -33.39374999877096428, 102.5980762113533018 ) ) ;
#16689=LINE ( 'NONE', #13841, #12716 ) ;
#16690=VERTEX_POINT ( 'NONE', #5532 ) ;
#16691=CARTESIAN_POINT ( 'NONE',  ( 229.8435696437499587, -34.34062499938547575, -51.59142580818350154 ) ) ;
#16693=CARTESIAN_POINT ( 'NONE',  ( 229.5999999999999375, -34.44374999877096144, 99.99999999999998579 ) ) ;
#16694=CARTESIAN_POINT ( 'NONE',  ( 233.9782151781249411, -30.85312499938547859, -52.38713871227520968 ) ) ;
#16695=CARTESIAN_POINT ( 'NONE',  ( 235.5999999999999943, -34.68749999999999289, -51.73205080756900287 ) ) ;
#16703=DIRECTION ( 'NONE',  ( 0.000000000000000000, -1.000000000000000000, 0.000000000000000000 ) ) ;
#16711=DIRECTION ( 'NONE',  ( 0.000000000000000000, 0.000000000000000000, -1.000000000000000000 ) ) ;
#16714=CARTESIAN_POINT ( 'NONE',  ( 235.3564303562499447, -32.61562499938548143, 99.99999999999998579 ) ) ;
#16715=ORIENTED_EDGE ( 'NONE', *, *, #16631, .F. ) ;
#16718=ORIENTED_EDGE ( 'NONE', *, *, #3518, .F. ) ;
#16724=ORIENTED_EDGE ( 'NONE', *, *, #13630, .T. ) ;
#16725=DIRECTION ( 'NONE',  ( -0.000000000000000000, -1.000000000000000000, -0.000000000000000000 ) ) ;
#16730=DIRECTION ( 'NONE',  ( 1.000000000000000000, 0.000000000000000000, -9.251858538542962756E-15 ) ) ;
#16731=CARTESIAN_POINT ( 'NONE',  ( 231.2217848218749339, -35.01562499938548001, 102.3871387122750889 ) ) ;
#16738=CARTESIAN_POINT ( 'NONE',  ( 232.5999999999999375, -33.48749999999999716, -46.53589838486234953 ) ) ;
#16741=DIRECTION ( 'NONE',  ( -1.000000000000000000, 0.000000000000000000, 0.000000000000000000 ) ) ;
#16743=CARTESIAN_POINT ( 'NONE',  ( 232.5999999999999375, -33.51562499938548001, -53.18285161636690361 ) ) ;
#16752=CARTESIAN_POINT ( 'NONE',  ( 230.1446115142671260, -35.00000000000138556, 98.27756861396923682 ) ) ;
#16756=CARTESIAN_POINT ( 'NONE',  ( 233.9782151781249411, -31.34062499938548285, -47.61286128772501769 ) ) ;
#16759=( BOUNDED_CURVE ( )  B_SPLINE_CURVE ( 2, ( #2091, #6498, #8245, #3653, #5129, #542, #834, #5034, #643 ),
 .UNSPECIFIED., .F., .F. ) 
 B_SPLINE_CURVE_WITH_KNOTS ( ( 3, 2, 2, 2, 3 ),
 ( 0.6875000000000000000, 0.6944444444444444198, 0.7083333333333333703, 0.7222222222222222099, 0.7291666666666667407 ),
 .UNSPECIFIED. ) 
 CURVE ( )  GEOMETRIC_REPRESENTATION_ITEM ( )  RATIONAL_B_SPLINE_CURVE ( ( 0.9330127018922194093, 0.9330127018922194093, 1.000000000000000000, 0.8660254037844387076, 1.000000000000000000, 0.8660254037844387076, 1.000000000000000000, 0.9330127018922187432, 0.9330127018922192983 ) ) 
 REPRESENTATION_ITEM ( '' )  );
#16766=PLANE ( 'NONE',  #15868 ) ;
#16767=EDGE_LOOP ( 'NONE', ( #9333, #3519, #491, #16862, #3299, #2133 ) ) ;
#16768=EDGE_CURVE ( 'NONE', #1370, #2004, #743, .T. ) ;
#16775=CARTESIAN_POINT ( 'NONE',  ( 233.4038475772933623, -32.77634618820330559, -53.00000000000010658 ) ) ;
#16776=CARTESIAN_POINT ( 'NONE',  ( 229.8435696437499018, -35.22676555956767430, 98.99674139749697588 ) ) ;
#16780=DIRECTION ( 'NONE',  ( -6.308085367188448025E-15, 0.000000000000000000, -1.000000000000000000 ) ) ;
#16791=CARTESIAN_POINT ( 'NONE',  ( 232.5999999999999943, -32.16562499938547859, -53.18285161636690361 ) ) ;
#16794=CARTESIAN_POINT ( 'NONE',  ( 229.8435696437499871, -31.64062499938547290, 98.40857419181659793 ) ) ;
#16795=CARTESIAN_POINT ( 'NONE',  ( 231.0999999999999375, -34.96874999877096002, -52.59807621135342970 ) ) ;
#16800=CARTESIAN_POINT ( 'NONE',  ( 232.5999999999999659, -32.53124999877096712, -47.00000000000011369 ) ) ;
#16812=CARTESIAN_POINT ( 'NONE',  ( 235.5999999999999943, -32.38124999877096144, 98.26794919243110371 ) ) ;
#16814=DIRECTION ( 'NONE',  ( -0.000000000000000000, -1.000000000000000000, -0.000000000000000000 ) ) ;
#16815=CARTESIAN_POINT ( 'NONE',  ( 235.3564303562499447, -34.00312499938547717, 101.5914258081833879 ) ) ;
#16816=CARTESIAN_POINT ( 'NONE',  ( 233.9782151781249411, -31.34062499938548285, 102.3871387122750889 ) ) ;
#16819=EDGE_CURVE ( 'NONE', #13951, #16293, #7180, .T. ) ;
#16820=CARTESIAN_POINT ( 'NONE',  ( 232.5999999999999375, -31.63124999877096144, 103.4641016151377499 ) ) ;
#16823=ORIENTED_EDGE ( 'NONE', *, *, #111, .F. ) ;
#16828=CARTESIAN_POINT ( 'NONE',  ( 229.8435696437499871, -34.22812499938547148, -51.59142580818350865 ) ) ;
#16834=( BOUNDED_CURVE ( )  B_SPLINE_CURVE ( 2, ( #9319, #10978, #3263, #3559, #7766, #360, #9416, #9517, #9622 ),
 .UNSPECIFIED., .F., .F. ) 
 B_SPLINE_CURVE_WITH_KNOTS ( ( 3, 2, 2, 2, 3 ),
 ( 0.8541666666666668517, 0.8611111111111111605, 0.8750000000000000000, 0.8888888888888888395, 0.8958333333333332593 ),
 .UNSPECIFIED. ) 
 CURVE ( )  GEOMETRIC_REPRESENTATION_ITEM ( )  RATIONAL_B_SPLINE_CURVE ( ( 0.9330127018922194093, 0.9330127018922209636, 1.000000000000000000, 0.8660254037844387076, 1.000000000000000000, 0.8660254037844387076, 1.000000000000000000, 0.9330127018922198534, 0.9330127018922192983 ) ) 
 REPRESENTATION_ITEM ( '' )  );
#16843=CARTESIAN_POINT ( 'NONE',  ( 234.0999999999999375, -31.64999999999999858, -47.40192378864679768 ) ) ;
#16846=CARTESIAN_POINT ( 'NONE',  ( 235.3564303562499447, -32.27812499938548285, 99.99999999999998579 ) ) ;
#16848=CARTESIAN_POINT ( 'NONE',  ( 233.9782151781249411, -32.35312499938547859, -47.61286128772501769 ) ) ;
#16859=CARTESIAN_POINT ( 'NONE',  ( 231.2217848218749339, -30.96562499938547930, -47.61286128772501769 ) ) ;
#16862=ORIENTED_EDGE ( 'NONE', *, *, #645, .F. ) ;
#16870=EDGE_CURVE ( 'NONE', #13568, #1894, #2726, .T. ) ;
#16875=CARTESIAN_POINT ( 'NONE',  ( 229.8435696437499303, -34.30312499938548143, 99.99999999999998579 ) ) ;
#16877=EDGE_LOOP ( 'NONE', ( #7541, #9286, #6202, #14937, #3720 ) ) ;
#16878=CARTESIAN_POINT ( 'NONE',  ( 232.5999999999999375, -34.78124999877096002, 102.9999999999999858 ) ) ;
#16883=DIRECTION ( 'NONE',  ( 1.000000000000000000, 0.000000000000000000, 0.000000000000000000 ) ) ;
#16885=CARTESIAN_POINT ( 'NONE',  ( 230.5523683116323355, -32.00000000000000000, -48.15470523285603832 ) ) ;
#16888=CARTESIAN_POINT ( 'NONE',  ( 231.2217848218749339, -34.82812499938548001, -52.38713871227520968 ) ) ;
#16890=CARTESIAN_POINT ( 'NONE',  ( 235.3564303562499447, -31.86562499938547788, 101.5914258081833879 ) ) ;
#16892=CARTESIAN_POINT ( 'NONE',  ( 232.5999999999999375, -30.81562499938547717, -53.18285161636690361 ) ) ;
#16895=EDGE_LOOP ( 'NONE', ( #10829, #8787, #2252, #5886, #12025 ) ) ;
#16899=LINE ( 'NONE', #13567, #10977 ) ;
#16906=CARTESIAN_POINT ( 'NONE',  ( 234.0999999999999375, -32.34374999877096002, 97.40192378864668399 ) ) ;
#16907=CARTESIAN_POINT ( 'NONE',  ( 233.3129826252977637, -32.00000000000000000, 102.8119722220550898 ) ) ;
#16908=CARTESIAN_POINT ( 'NONE',  ( 229.8435696437499871, -33.77812499938548285, 98.40857419181659793 ) ) ;
#16911=CARTESIAN_POINT ( 'NONE',  ( 235.5999999999999375, -30.61874999877096215, 99.99999999999998579 ) ) ;
#16915=CARTESIAN_POINT ( 'NONE',  ( -1.840441912298296046E-29, -3.702689427376452761E-13, -103.0000000000001137 ) ) ;
#16917=ORIENTED_EDGE ( 'NONE', *, *, #16183, .F. ) ;
#16921=EDGE_LOOP ( 'NONE', ( #8352, #11768, #4591, #5988 ) ) ;
#16936=CARTESIAN_POINT ( 'NONE',  ( 229.5999999999999375, -31.83749999999999858, -51.73205080756898866 ) ) ;
#16938=CARTESIAN_POINT ( 'NONE',  ( 229.8435696437499587, -32.09062499938548285, 98.40857419181659793 ) ) ;
#16940=CARTESIAN_POINT ( 'NONE',  ( 232.5999999999999375, -33.06562499938547717, -53.18285161636690361 ) ) ;
#16942=EDGE_LOOP ( 'NONE', ( #12201, #5472, #15158, #7726 ) ) ;
#16949=CARTESIAN_POINT ( 'NONE',  ( 244.7999999999999545, -32.00000000000000000, -100.0000000000000000 ) ) ;
#16952=CARTESIAN_POINT ( 'NONE',  ( 229.8435696437499871, -31.45312499938547290, -48.40857419181671162 ) ) ;
#16957=ADVANCED_FACE ( 'NONE', ( #9119 ), #14790, .F. ) ;
#16958=CYLINDRICAL_SURFACE ( 'NONE', #5876, 2.199999999999993516 ) ;
#16967=CARTESIAN_POINT ( 'NONE',  ( 233.9782151781249411, -34.15312499938547575, 102.3871387122750889 ) ) ;
#16969=ORIENTED_EDGE ( 'NONE', *, *, #7530, .F. ) ;
#16970=CARTESIAN_POINT ( 'NONE',  ( 229.5999999999999375, -32.69999999999999574, 99.99999999999998579 ) ) ;
#16972=CARTESIAN_POINT ( 'NONE',  ( 229.8848725447336392, -31.99999999999997158, 100.5952676699192381 ) ) ;
#16980=CARTESIAN_POINT ( 'NONE',  ( 231.2217848218749339, -31.97812499938548214, 102.3871387122750889 ) ) ;
#16981=CARTESIAN_POINT ( 'NONE',  ( 235.3564303562499447, -31.79062499938547859, -51.59142580818350865 ) ) ;
#16994=EDGE_CURVE ( 'NONE', #7775, #8999, #2434, .T. ) ;
#16998=LINE ( 'NONE', #10841, #14253 ) ;
#17000=CARTESIAN_POINT ( 'NONE',  ( 232.5999999999999375, -34.30312499938547433, 96.81714838363319586 ) ) ;
#17005=CARTESIAN_POINT ( 'NONE',  ( 229.5999999999999375, -30.84374999877096357, 99.99999999999998579 ) ) ;
#17006=CARTESIAN_POINT ( 'NONE',  ( 229.5999999999999375, -32.19374999877096144, 99.99999999999998579 ) ) ;
#17012=VERTEX_POINT ( 'NONE', #7272 ) ;
#17015=ORIENTED_EDGE ( 'NONE', *, *, #2656, .T. ) ;
#17024=CARTESIAN_POINT ( 'NONE',  ( 232.5999999999999091, -33.03749999999998721, 102.9999999999999858 ) ) ;
#17029=AXIS2_PLACEMENT_3D ( 'NONE', #12860, #15797, #2591 ) ;
#17035=CARTESIAN_POINT ( 'NONE',  ( 229.5999999999999375, -34.91249999999999432, -48.26794919243123161 ) ) ;
#17038=CARTESIAN_POINT ( 'NONE',  ( 229.8435696437499303, -32.50312499938547717, -50.00000000000011369 ) ) ;
#17044=CARTESIAN_POINT ( 'NONE',  ( 230.4319669496466076, -32.00000000000000000, -48.28830862702061921 ) ) ;
#17045=EDGE_CURVE ( 'NONE', #12372, #16126, #11411, .T. ) ;
#17051=CARTESIAN_POINT ( 'NONE',  ( 232.5999999999999375, -34.30312499938547433, -53.18285161636690361 ) ) ;
#17062=CARTESIAN_POINT ( 'NONE',  ( 229.5999999999999375, -34.40624999877096002, -48.26794919243123161 ) ) ;
#17063=CARTESIAN_POINT ( 'NONE',  ( 232.1497501643324881, -35.00000000000000711, -52.97309102824105764 ) ) ;
#17065=CARTESIAN_POINT ( 'NONE',  ( 229.8435696437499871, -31.97812499938548214, 98.40857419181659793 ) ) ;
#17067=CARTESIAN_POINT ( 'NONE',  ( 230.7186334667984227, -32.00000000000000711, -52.01453922190813728 ) ) ;
#17071=CARTESIAN_POINT ( 'NONE',  ( 105.1999999999999744, -34.51168759575591594, -100.0000000000000000 ) ) ;
#17078=CARTESIAN_POINT ( 'NONE',  ( 229.8435696437499871, -33.36562499938548143, 101.5914258081833879 ) ) ;
#17079=CARTESIAN_POINT ( 'NONE',  ( 233.9782151781249411, -32.35312499938547859, -47.61286128772501769 ) ) ;
#17080=STYLED_ITEM ( 'NONE', ( #16530 ), #5537 ) ;
#17082=CARTESIAN_POINT ( 'NONE',  ( 244.7999999999999545, -29.80000000000002203, 150.0000000000000000 ) ) ;
#17083=ORIENTED_EDGE ( 'NONE', *, *, #18438, .F. ) ;
#17089=AXIS2_PLACEMENT_3D ( 'NONE', #10756, #15255, #6663 ) ;
#17097=CARTESIAN_POINT ( 'NONE',  ( 232.1497501643324881, -35.00000000000000711, 97.02690897175904183 ) ) ;
#17099=CARTESIAN_POINT ( 'NONE',  ( 232.5999999999999375, -33.40312499938547575, 96.81714838363319586 ) ) ;
#17103=CARTESIAN_POINT ( 'NONE',  ( 234.0999999999999375, -31.14374999877096428, 102.5980762113533018 ) ) ;
#17108=DIRECTION ( 'NONE',  ( -0.000000000000000000, -1.000000000000000000, -0.000000000000000000 ) ) ;
#17113=( BOUNDED_CURVE ( )  B_SPLINE_CURVE ( 2, ( #7288, #2695, #14804, #1624, #13243, #7385, #5832, #9042, #7484 ),
 .UNSPECIFIED., .F., .F. ) 
 B_SPLINE_CURVE_WITH_KNOTS ( ( 3, 2, 2, 2, 3 ),
 ( 0.5625000000000002220, 0.5694444444444444198, 0.5833333333333333703, 0.5972222222222222099, 0.6041666666666667407 ),
 .UNSPECIFIED. ) 
 CURVE ( )  GEOMETRIC_REPRESENTATION_ITEM ( )  RATIONAL_B_SPLINE_CURVE ( ( 0.9330127018922194093, 0.9330127018922215187, 1.000000000000000000, 0.8660254037844387076, 1.000000000000000000, 0.8660254037844387076, 1.000000000000000000, 0.9330127018922187432, 0.9330127018922192983 ) ) 
 REPRESENTATION_ITEM ( '' )  );
#17115=CARTESIAN_POINT ( 'NONE',  ( 232.5999999999999375, -32.98124999877095576, 102.9999999999999858 ) ) ;
#17123=CARTESIAN_POINT ( 'NONE',  ( 233.2908335840014615, -34.99999999999998579, -52.88685016125990046 ) ) ;
#17130=EDGE_LOOP ( 'NONE', ( #6856, #4986, #9194, #830 ) ) ;
#17133=CYLINDRICAL_SURFACE ( 'NONE', #18966, 3.000000000000009770 ) ;
#17135=EDGE_CURVE ( 'NONE', #3211, #6709, #8601, .T. ) ;
#17136=CARTESIAN_POINT ( 'NONE',  ( 231.2217848218749339, -35.12812499938548427, -47.61286128772501769 ) ) ;
#17140=DIRECTION ( 'NONE',  ( 0.000000000000000000, 0.000000000000000000, 1.000000000000000000 ) ) ;
#17143=CARTESIAN_POINT ( 'NONE',  ( 232.5999999999999943, -32.27812499938547575, -46.81714838363331666 ) ) ;
#17148=CARTESIAN_POINT ( 'NONE',  ( 233.9782151781249411, -32.99062499938548143, -52.38713871227520968 ) ) ;
#17153=CARTESIAN_POINT ( 'NONE',  ( 233.4038475772933623, -32.77634618820330559, 97.00000000000000000 ) ) ;
#17158=FACE_OUTER_BOUND ( 'NONE', #15323, .T. ) ;
#17164=CARTESIAN_POINT ( 'NONE',  ( 232.5999999999999375, -34.16249999999999432, -53.00000000000010658 ) ) ;
#17166=CARTESIAN_POINT ( 'NONE',  ( 229.8435696437499303, -31.04062499938547859, 99.99999999999998579 ) ) ;
#17177=ORIENTED_EDGE ( 'NONE', *, *, #16427, .T. ) ;
#17180=CARTESIAN_POINT ( 'NONE',  ( 232.5999999999999375, -31.94062499938548072, 103.1828516163667899 ) ) ;
#17181=CARTESIAN_POINT ( 'NONE',  ( 235.3564303562499447, -33.14062499938548001, -51.59142580818350865 ) ) ;
#17197=CARTESIAN_POINT ( 'NONE',  ( 229.8435696437499871, -34.15312499938547575, 101.5914258081833879 ) ) ;
#17201=CARTESIAN_POINT ( 'NONE',  ( 229.5999999999999375, -31.33124999877096073, -51.73205080756898866 ) ) ;
#17202=EDGE_LOOP ( 'NONE', ( #15149, #253, #12875, #18621 ) ) ;
#17203=CARTESIAN_POINT ( 'NONE',  ( 231.7961524227065695, -34.40759618943233988, 102.9999999999999858 ) ) ;
#17213=CARTESIAN_POINT ( 'NONE',  ( 232.5999999999999375, -32.30624999877096570, 97.00000000000000000 ) ) ;
#17222=ORIENTED_EDGE ( 'NONE', *, *, #5066, .T. ) ;
#17223=CARTESIAN_POINT ( 'NONE',  ( 229.5999999999999375, -34.94999999999999574, -50.00000000000011369 ) ) ;
#17229=CARTESIAN_POINT ( 'NONE',  ( 231.2217848218749339, -33.32812499938548001, 102.3871387122750889 ) ) ;
#17231=CARTESIAN_POINT ( 'NONE',  ( 232.5999999999999375, -30.70312499938548001, -53.18285161636690361 ) ) ;
#17246=CARTESIAN_POINT ( 'NONE',  ( 235.3564303562499447, -32.61562499938548143, -50.00000000000011369 ) ) ;
#17254=AXIS2_PLACEMENT_3D ( 'NONE', #6745, #3318, #15333 ) ;
#17269=VECTOR ( 'NONE', #17502, 1000.000000000000000 ) ;
#17270=CYLINDRICAL_SURFACE ( 'NONE', #18681, 3.000000000000009770 ) ;
#17278=CARTESIAN_POINT ( 'NONE',  ( 229.8435696437499871, -35.16562499938547148, 101.5914258081833879 ) ) ;
#17279=CARTESIAN_POINT ( 'NONE',  ( 229.8435696437499871, -34.26562499938548001, -48.40857419181671162 ) ) ;
#17282=ORIENTED_EDGE ( 'NONE', *, *, #10313, .F. ) ;
#17296=CARTESIAN_POINT ( 'NONE',  ( 235.5999999999999943, -30.71249999999999858, 101.7320508075688537 ) ) ;
#17299=CARTESIAN_POINT ( 'NONE',  ( 229.5999999999999375, -33.99374999877096570, 99.99999999999998579 ) ) ;
#17300=CARTESIAN_POINT ( 'NONE',  ( 231.0999999999999375, -32.26874999877096428, -52.59807621135342970 ) ) ;
#17307=CARTESIAN_POINT ( 'NONE',  ( 232.5999999999999375, -33.20624999877097139, 97.00000000000000000 ) ) ;
#17315=CARTESIAN_POINT ( 'NONE',  ( 235.3594282536527089, -35.00000000000000000, -49.60353574117735320 ) ) ;
#17322=CARTESIAN_POINT ( 'NONE',  ( 234.0999999999999375, -34.19999999999999574, -52.59807621135342970 ) ) ;
#17323=CARTESIAN_POINT ( 'NONE',  ( 235.2646886264966213, -35.00000000000002132, 98.99456257074425025 ) ) ;
#17325=CARTESIAN_POINT ( 'NONE',  ( 229.8435696437499587, -34.79062499938547859, 98.40857419181659793 ) ) ;
#17327=CARTESIAN_POINT ( 'NONE',  ( 233.9782151781249411, -30.29062499938547859, -52.38713871227520968 ) ) ;
#17334=CARTESIAN_POINT ( 'NONE',  ( 231.7961524227065979, -33.18615380933862724, -53.00000000000009948 ) ) ;
#17336=CARTESIAN_POINT ( 'NONE',  ( 235.3564303562499447, -32.61562499938548143, -50.00000000000011369 ) ) ;
#17342=CARTESIAN_POINT ( 'NONE',  ( 229.8435696437499871, -31.97812499938548214, -51.59142580818350865 ) ) ;
#17345=ORIENTED_EDGE ( 'NONE', *, *, #13150, .T. ) ;
#17347=CARTESIAN_POINT ( 'NONE',  ( 233.4038475772933339, -34.31115380933863435, -47.00000000000012790 ) ) ;
#17353=CARTESIAN_POINT ( 'NONE',  ( 232.5999999999999943, -33.17812499938548143, 103.1828516163667899 ) ) ;
#17354=CARTESIAN_POINT ( 'NONE',  ( 232.5999999999999375, -33.93749999999999289, -47.00000000000011369 ) ) ;
#17359=CARTESIAN_POINT ( 'NONE',  ( 232.5999999999999375, -29.99999999999999645, 96.99999999999998579 ) ) ;
#17361=LINE ( 'NONE', #3971, #4955 ) ;
#17363=CARTESIAN_POINT ( 'NONE',  ( 234.3965303555544608, -32.00000000000000711, 97.67482724152034734 ) ) ;
#17366=CARTESIAN_POINT ( 'NONE',  ( 229.5999999999999375, -34.01249999999999574, 101.7320508075688821 ) ) ;
#17369=CARTESIAN_POINT ( 'NONE',  ( 235.3564303562499447, -34.04062499938547859, 98.40857419181659793 ) ) ;
#17370=CARTESIAN_POINT ( 'NONE',  ( 233.9782151781249411, -31.90312499938548285, -47.61286128772501769 ) ) ;
#17371=EDGE_CURVE ( 'NONE', #14052, #5719, #14285, .T. ) ;
#17377=FACE_OUTER_BOUND ( 'NONE', #14772, .T. ) ;
#17388=CARTESIAN_POINT ( 'NONE',  ( 230.5724978686189672, -35.00000000000000711, 97.77995849557630947 ) ) ;
#17389=EDGE_CURVE ( 'NONE', #17445, #16126, #18665, .T. ) ;
#17392=CARTESIAN_POINT ( 'NONE',  ( 235.5999999999999375, -31.57499999999999218, 99.99999999999998579 ) ) ;
#17395=CARTESIAN_POINT ( 'NONE',  ( 229.5999999999999375, -32.19374999877096144, 99.99999999999998579 ) ) ;
#17396=CARTESIAN_POINT ( 'NONE',  ( 234.0999999999999375, -30.69374999877096499, -47.40192378864679768 ) ) ;
#17402=ORIENTED_EDGE ( 'NONE', *, *, #12826, .T. ) ;
#17406=CARTESIAN_POINT ( 'NONE',  ( 105.1999999999999744, -29.80000000000002203, 150.0000000000000000 ) ) ;
#17410=VECTOR ( 'NONE', #15757, 1000.000000000000000 ) ;
#17424=VECTOR ( 'NONE', #1600, 1000.000000000000000 ) ;
#17429=CARTESIAN_POINT ( 'NONE',  ( 235.3564303562499447, -30.77812499938547575, -51.59142580818350865 ) ) ;
#17431=AXIS2_PLACEMENT_3D ( 'NONE', #14597, #4539, #19015 ) ;
#17437=CARTESIAN_POINT ( 'NONE',  ( 235.3564303562499447, -32.12812499938547717, -51.59142580818350154 ) ) ;
#17442=CARTESIAN_POINT ( 'NONE',  ( 233.9782151781249411, -32.69062499938547717, -47.61286128772501769 ) ) ;
#17445=VERTEX_POINT ( 'NONE', #5884 ) ;
#17453=CARTESIAN_POINT ( 'NONE',  ( 235.3564303562499447, -33.55312499938548143, 101.5914258081833879 ) ) ;
#17460=CARTESIAN_POINT ( 'NONE',  ( 230.2593261479345585, -31.99999999999999289, 98.53339280468536288 ) ) ;
#17465=CARTESIAN_POINT ( 'NONE',  ( 249.9999999999999716, -35.00000000000000000, 150.0000000000000000 ) ) ;
#17466=EDGE_LOOP ( 'NONE', ( #12869, #16020, #13826, #10166 ) ) ;
#17468=CARTESIAN_POINT ( 'NONE',  ( 231.2217848218749339, -35.12812499938548427, 102.3871387122750889 ) ) ;
#17469=CARTESIAN_POINT ( 'NONE',  ( 231.2217848218749339, -33.77812499938547575, -47.61286128772501769 ) ) ;
#17471=EDGE_CURVE ( 'NONE', #7231, #19103, #1481, .T. ) ;
#17474=ORIENTED_EDGE ( 'NONE', *, *, #757, .F. ) ;
#17476=DIRECTION ( 'NONE',  ( 1.735459783503185124E-31, 3.491481338843133355E-15, 1.000000000000000000 ) ) ;
#17477=ORIENTED_EDGE ( 'NONE', *, *, #12861, .F. ) ;
#17484=ADVANCED_FACE ( 'NONE', ( #2721 ), #7600, .T. ) ;
#17485=DIRECTION ( 'NONE',  ( 0.000000000000000000, 0.000000000000000000, -1.000000000000000000 ) ) ;
#17488=ADVANCED_FACE ( 'NONE', ( #12094 ), #16501, .T. ) ;
#17490=CARTESIAN_POINT ( 'NONE',  ( 229.5999999999999375, -32.24999999999999289, 99.99999999999998579 ) ) ;
#17492=CARTESIAN_POINT ( 'NONE',  ( 230.5523683116323355, -32.00000000000000000, -48.15470523285603832 ) ) ;
#17493=CARTESIAN_POINT ( 'NONE',  ( 234.0999999999999375, -33.39374999877096428, 102.5980762113533018 ) ) ;
#17494=CARTESIAN_POINT ( 'NONE',  ( 231.0999999999999375, -31.21874999877096357, -47.40192378864679768 ) ) ;
#17502=DIRECTION ( 'NONE',  ( 1.000000000000000000, 0.000000000000000000, 0.000000000000000000 ) ) ;
#17507=CARTESIAN_POINT ( 'NONE',  ( 235.2218879900010506, -35.00000000000000000, -49.14934632385183022 ) ) ;
#17516=CARTESIAN_POINT ( 'NONE',  ( 234.9631320699431001, -35.00000000000000000, 98.35371953419910085 ) ) ;
#17518=CARTESIAN_POINT ( 'NONE',  ( 229.8435696437499587, -34.34062499938547575, 98.40857419181659793 ) ) ;
#17521=CARTESIAN_POINT ( 'NONE',  ( 229.8435696437499303, -34.75312499938547717, -50.00000000000011369 ) ) ;
#17528=CARTESIAN_POINT ( 'NONE',  ( 232.5999999999999375, -30.47812499938547859, 103.1828516163667899 ) ) ;
#17529=CARTESIAN_POINT ( 'NONE',  ( 229.8435696437499587, -32.35312499938547859, -48.40857419181671162 ) ) ;
#17534=CARTESIAN_POINT ( 'NONE',  ( 231.0999999999999375, -31.27499999999999858, -47.40192378864679768 ) ) ;
#17537=EDGE_LOOP ( 'NONE', ( #6989, #18850, #9970, #4077 ) ) ;
#17547=CARTESIAN_POINT ( 'NONE',  ( 231.2217848218749339, -32.91562499938547148, 97.61286128772489690 ) ) ;
#17548=DIRECTION ( 'NONE',  ( 1.000000000000000000, -0.000000000000000000, -0.000000000000000000 ) ) ;
#17564=CARTESIAN_POINT ( 'NONE',  ( 231.2217848218749339, -34.82812499938548001, 97.61286128772489690 ) ) ;
#17567=CARTESIAN_POINT ( 'NONE',  ( 231.7961524227065979, -32.60759618943232852, -47.00000000000010658 ) ) ;
#17580=CARTESIAN_POINT ( 'NONE',  ( 231.9680721332268831, -35.00000000000000000, 102.6890373435399937 ) ) ;
#17582=CARTESIAN_POINT ( 'NONE',  ( 235.5999999999999375, -31.12499999999999645, 99.99999999999998579 ) ) ;
#17583=ORIENTED_EDGE ( 'NONE', *, *, #539, .T. ) ;
#17585=CARTESIAN_POINT ( 'NONE',  ( 234.0999999999999375, -32.34374999877096002, 97.40192378864668399 ) ) ;
#17586=CARTESIAN_POINT ( 'NONE',  ( 229.5999999999999375, -32.68124999877096570, -51.73205080756898866 ) ) ;
#17587=CARTESIAN_POINT ( 'NONE',  ( 232.5999999999999659, -32.53124999877096712, 102.9999999999999858 ) ) ;
#17600=CARTESIAN_POINT ( 'NONE',  ( 234.0999999999999375, -32.34374999877096002, -52.59807621135342970 ) ) ;
#17605=CARTESIAN_POINT ( 'NONE',  ( 233.9782151781249411, -30.29062499938547859, 97.61286128772489690 ) ) ;
#17610=CARTESIAN_POINT ( 'NONE',  ( 229.8435696437499303, -33.85312499938548569, 99.99999999999998579 ) ) ;
#17614=CARTESIAN_POINT ( 'NONE',  ( 231.2217848218749339, -33.66562499938547859, -47.61286128772501769 ) ) ;
#17619=EDGE_CURVE ( 'NONE', #12080, #4350, #17729, .T. ) ;
#17623=CARTESIAN_POINT ( 'NONE',  ( 235.3564303562499447, -30.81562499938547717, 99.99999999999998579 ) ) ;
#17625=CARTESIAN_POINT ( 'NONE',  ( 232.5999999999999943, -34.52812499938547575, -46.81714838363331666 ) ) ;
#17630=CARTESIAN_POINT ( 'NONE',  ( 231.7447645400923193, -35.19352049914630953, -53.26902605122407408 ) ) ;
#17637=CARTESIAN_POINT ( 'NONE',  ( 231.2217848218749339, -31.67812499938547788, -52.38713871227520968 ) ) ;
#17643=CARTESIAN_POINT ( 'NONE',  ( 232.5999999999999943, -32.50312499938547717, 96.81714838363319586 ) ) ;
#17647=CARTESIAN_POINT ( 'NONE',  ( 232.5999999999999659, -32.13749999999999574, 103.0000000000000000 ) ) ;
#17652=CARTESIAN_POINT ( 'NONE',  ( 232.5999999999999375, -33.71249999999999147, -53.00000000000010658 ) ) ;
#17656=VECTOR ( 'NONE', #18225, 1000.000000000000000 ) ;
#17659=CARTESIAN_POINT ( 'NONE',  ( 232.1454721953968772, -35.00000000000000711, -47.27546421900289886 ) ) ;
#17660=CARTESIAN_POINT ( 'NONE',  ( 102.9999999999999858, -5.200000000000008171, -100.0000000000000000 ) ) ;
#17671=CARTESIAN_POINT ( 'NONE',  ( 232.5999999999999375, -32.61562499938548143, 96.81714838363319586 ) ) ;
#17678=CARTESIAN_POINT ( 'NONE',  ( 231.0999999999999375, -30.82499999999999574, 102.5980762113533018 ) ) ;
#17680=ORIENTED_EDGE ( 'NONE', *, *, #3467, .T. ) ;
#17683=CARTESIAN_POINT ( 'NONE',  ( 234.0999999999999375, -33.24374999877096570, 97.40192378864668399 ) ) ;
#17684=CARTESIAN_POINT ( 'NONE',  ( 234.0999999999999375, -34.29374999877096286, -47.40192378864679768 ) ) ;
#17686=ORIENTED_EDGE ( 'NONE', *, *, #14467, .F. ) ;
#17699=CARTESIAN_POINT ( 'NONE',  ( 230.7186334667984227, -32.00000000000000711, -52.01453922190813728 ) ) ;
#17704=STYLED_ITEM('',(#19350),#3102);
#17708=ADVANCED_FACE ( 'NONE', ( #6143 ), #11707, .T. ) ;
#17713=CARTESIAN_POINT ( 'NONE',  ( 235.3564303562499447, -33.92812499938548143, -51.59142580818350865 ) ) ;
#17716=VECTOR ( 'NONE', #18047, 1000.000000000000000 ) ;
#17726=CARTESIAN_POINT ( 'NONE',  ( 235.3564303562499447, -30.40312499938547575, 101.5914258081833879 ) ) ;
#17727=CARTESIAN_POINT ( 'NONE',  ( 232.5999999999999943, -34.07812499938548001, -46.81714838363331666 ) ) ;
#17729=CIRCLE ( 'NONE', #16483, 2.200000000000007283 ) ;
#17734=CARTESIAN_POINT ( 'NONE',  ( 235.5999999999999375, -31.12499999999999645, -50.00000000000011369 ) ) ;
#17748=CARTESIAN_POINT ( 'NONE',  ( 231.2217848218749339, -32.46562499938547575, 97.61286128772489690 ) ) ;
#17752=DIRECTION ( 'NONE',  ( 1.000000000000000000, -4.970554372426382520E-17, -0.000000000000000000 ) ) ;
#17754=CARTESIAN_POINT ( 'NONE',  ( 230.2491162085250664, -34.99999999999999289, 101.6079878054125487 ) ) ;
#17759=VERTEX_POINT ( 'NONE', #2127 ) ;
#17762=CARTESIAN_POINT ( 'NONE',  ( 232.5999999999999375, -35.09062499938547575, -46.81714838363331666 ) ) ;
#17769=CARTESIAN_POINT ( 'NONE',  ( 229.5999999999999375, -33.60000000000000142, -50.00000000000011369 ) ) ;
#17774=CARTESIAN_POINT ( 'NONE',  ( 235.3564303562499447, -32.76562499938548001, 101.5914258081833879 ) ) ;
#17781=CARTESIAN_POINT ( 'NONE',  ( 235.5999999999999943, -33.41250000000000142, 101.7320508075688537 ) ) ;
#17784=CARTESIAN_POINT ( 'NONE',  ( 105.1999999999999602, -29.80000000000001492, -97.80000000000002558 ) ) ;
#17785=CARTESIAN_POINT ( 'NONE',  ( 230.3018604581529871, -35.39427337414328889, 98.07164457472185859 ) ) ;
#17786=CARTESIAN_POINT ( 'NONE',  ( 232.5999999999999375, -32.30624999877095860, -53.46410161513786363 ) ) ;
#17793=ORIENTED_EDGE ( 'NONE', *, *, #11611, .T. ) ;
#17800=CARTESIAN_POINT ( 'NONE',  ( 235.3564303562499447, -30.32812499938548001, 98.40857419181659793 ) ) ;
#17806=CARTESIAN_POINT ( 'NONE',  ( 244.7999999999999545, -4.999999999999976907, 153.0000000000000000 ) ) ;
#17810=CARTESIAN_POINT ( 'NONE',  ( 235.3564303562499447, -32.65312499938547575, -48.40857419181671162 ) ) ;
#17818=CARTESIAN_POINT ( 'NONE',  ( 235.3564303562499447, -34.00312499938547717, 101.5914258081833879 ) ) ;
#17821=EDGE_CURVE ( 'NONE', #10754, #16690, #13747, .T. ) ;
#17823=CARTESIAN_POINT ( 'NONE',  ( 229.8435696437499871, -35.05312499938547433, -48.40857419181671162 ) ) ;
#17827=DIRECTION ( 'NONE',  ( 0.000000000000000000, 0.000000000000000000, 1.000000000000000000 ) ) ;
#17829=CARTESIAN_POINT ( 'NONE',  ( 229.8435696437499303, -31.60312499938548214, -50.00000000000011369 ) ) ;
#17831=ORIENTED_EDGE ( 'NONE', *, *, #12813, .T. ) ;
#17837=DIRECTION ( 'NONE',  ( 1.000000000000000000, 0.000000000000000000, -0.000000000000000000 ) ) ;
#17838=CARTESIAN_POINT ( 'NONE',  ( 230.8769377533405986, -32.00000000000000711, -47.80849716182774500 ) ) ;
#17844=CARTESIAN_POINT ( 'NONE',  ( 231.0999999999999375, -34.81874999877096144, 102.5980762113533018 ) ) ;
#17851=CARTESIAN_POINT ( 'NONE',  ( 235.3564303562499447, -34.94062499938547717, -51.59142580818350865 ) ) ;
#17852=CIRCLE ( 'NONE', #389, 2.200000000000007283 ) ;
#17854=VECTOR ( 'NONE', #10378, 1000.000000000000000 ) ;
#17861=CARTESIAN_POINT ( 'NONE',  ( 231.7961524227065979, -33.50759618943233420, -47.00000000000011369 ) ) ;
#17863=CARTESIAN_POINT ( 'NONE',  ( 229.5999999999999375, -33.50624999877096144, -48.26794919243123161 ) ) ;
#17865=CARTESIAN_POINT ( 'NONE',  ( 235.3564303562499447, -31.37812499938547717, 99.99999999999998579 ) ) ;
#17873=CARTESIAN_POINT ( 'NONE',  ( 235.5999999999999943, -33.35624999877096286, 101.7320508075688537 ) ) ;
#17875=CARTESIAN_POINT ( 'NONE',  ( 235.5999999999999943, -33.86249999999999716, 101.7320508075688537 ) ) ;
#17877=CARTESIAN_POINT ( 'NONE',  ( 233.9782151781249411, -33.10312499938547859, -52.38713871227520968 ) ) ;
#17879=ADVANCED_FACE ( 'NONE', ( #4678 ), #12290, .F. ) ;
#17880=CARTESIAN_POINT ( 'NONE',  ( 229.5999999999999943, -35.36739044046695568, 98.90809476984486537 ) ) ;
#17881=CARTESIAN_POINT ( 'NONE',  ( 229.5999999999999375, -33.58124999877096428, -51.73205080756898866 ) ) ;
#17883=ORIENTED_EDGE ( 'NONE', *, *, #3514, .T. ) ;
#17889=VERTEX_POINT ( 'NONE', #3198 ) ;
#17890=DIRECTION ( 'NONE',  ( 0.000000000000000000, 6.982962677686266711E-15, -1.000000000000000000 ) ) ;
#17895=DIRECTION ( 'NONE',  ( 0.000000000000000000, 0.000000000000000000, -1.000000000000000000 ) ) ;
#17899=DIRECTION ( 'NONE',  ( -1.000000000000000000, 0.000000000000000000, 0.000000000000000000 ) ) ;
#17909=CARTESIAN_POINT ( 'NONE',  ( 232.5999999999999375, -33.17812499938548143, -46.81714838363331666 ) ) ;
#17912=CYLINDRICAL_SURFACE ( 'NONE', #3840, 3.000000000000009770 ) ;
#17917=CARTESIAN_POINT ( 'NONE',  ( 231.2217848218749339, -33.66562499938547859, 102.3871387122750889 ) ) ;
#17918=CARTESIAN_POINT ( 'NONE',  ( 229.8435696437499587, -34.60312499938547859, -48.40857419181671162 ) ) ;
#17922=CARTESIAN_POINT ( 'NONE',  ( 229.5999999999999375, -30.48749999999999005, -51.73205080756898866 ) ) ;
#17926=DIRECTION ( 'NONE',  ( 0.000000000000000000, 0.000000000000000000, -1.000000000000000000 ) ) ;
#17927=CARTESIAN_POINT ( 'NONE',  ( 233.9782151781249411, -30.40312499938547930, -52.38713871227520968 ) ) ;
#17938=CARTESIAN_POINT ( 'NONE',  ( 244.7999999999999545, -4.999999999999976907, 150.0000000000000000 ) ) ;
#17944=ORIENTED_EDGE ( 'NONE', *, *, #13225, .T. ) ;
#17948=EDGE_CURVE ( 'NONE', #8464, #8905, #12189, .T. ) ;
#17952=CARTESIAN_POINT ( 'NONE',  ( 244.7999999999999545, -29.80000000000000426, -100.0000000000000000 ) ) ;
#17959=CARTESIAN_POINT ( 'NONE',  ( 231.0999999999999375, -33.46874999877096002, -47.40192378864679768 ) ) ;
#17960=CARTESIAN_POINT ( 'NONE',  ( 232.5999999999999375, -32.16562499938547859, 96.81714838363319586 ) ) ;
#17969=CARTESIAN_POINT ( 'NONE',  ( 235.5999999999999375, -33.37499999999999289, 99.99999999999998579 ) ) ;
#17973=CARTESIAN_POINT ( 'NONE',  ( 232.5999999999999943, -33.96562499938547575, -53.18285161636690361 ) ) ;
#17975=CARTESIAN_POINT ( 'NONE',  ( 232.5999999999999375, -34.10624999877096286, 96.53589838486223584 ) ) ;
#17976=CARTESIAN_POINT ( 'NONE',  ( 235.5999999999999943, -32.38124999877096144, -51.73205080756900287 ) ) ;
#17981=CARTESIAN_POINT ( 'NONE',  ( 229.5999999999999375, -32.64374999877096428, -50.00000000000011369 ) ) ;
#17984=DIRECTION ( 'NONE',  ( 0.000000000000000000, 0.000000000000000000, 1.000000000000000000 ) ) ;
#17991=CARTESIAN_POINT ( 'NONE',  ( 235.4117376914898898, -32.00000000000000000, -51.04600724388262023 ) ) ;
#17993=CARTESIAN_POINT ( 'NONE',  ( 235.5999999999999943, -33.33749999999999147, 98.26794919243110371 ) ) ;
#17999=( LENGTH_UNIT ( ) NAMED_UNIT ( * ) SI_UNIT ( .MILLI., .METRE. ) );
#18002=CARTESIAN_POINT ( 'NONE',  ( 231.0999999999999375, -34.36874999877096570, 102.5980762113533018 ) ) ;
#18006=CARTESIAN_POINT ( 'NONE',  ( 231.2217848218749339, -32.46562499938547575, -52.38713871227520968 ) ) ;
#18015=EDGE_CURVE ( 'NONE', #6930, #2849, #17361, .T. ) ;
#18016=PRODUCT_DEFINITION ( 'UNKNOWN', '', #9886, #12171 ) ;
#18017=CARTESIAN_POINT ( 'NONE',  ( 232.5999999999999375, -32.00000000000000000, 99.99999999999998579 ) ) ;
#18018=CARTESIAN_POINT ( 'NONE',  ( 231.2217848218749339, -33.81562499938547717, 97.61286128772489690 ) ) ;
#18019=CARTESIAN_POINT ( 'NONE',  ( 231.2217848218749339, -33.81562499938547717, -52.38713871227520968 ) ) ;
#18025=CARTESIAN_POINT ( 'NONE',  ( 232.5999999999999375, -33.26249999999999574, -53.46410161513786363 ) ) ;
#18042=CARTESIAN_POINT ( 'NONE',  ( 235.3140393761304665, -32.00000000000000000, -48.72172371342785624 ) ) ;
#18047=DIRECTION ( 'NONE',  ( -0.000000000000000000, -0.000000000000000000, -1.000000000000000000 ) ) ;
#18057=ORIENTED_EDGE ( 'NONE', *, *, #3143, .T. ) ;
#18062=CARTESIAN_POINT ( 'NONE',  ( 235.3564303562499447, -31.86562499938547788, 101.5914258081833879 ) ) ;
#18067=CARTESIAN_POINT ( 'NONE',  ( 105.1999999999999744, -31.99999999999999289, 150.0000000000000000 ) ) ;
#18068=CARTESIAN_POINT ( 'NONE',  ( 233.4038475772932770, -33.41115380933862156, 103.0000000000000000 ) ) ;
#18070=CARTESIAN_POINT ( 'NONE',  ( 231.0999999999999375, -33.22499999999999432, 97.40192378864668399 ) ) ;
#18074=CARTESIAN_POINT ( 'NONE',  ( 229.8435696437499587, -32.99062499938548143, -51.59142580818350154 ) ) ;
#18076=CARTESIAN_POINT ( 'NONE',  ( 231.0999999999999375, -34.81874999877096144, 102.5980762113533018 ) ) ;
#18077=CARTESIAN_POINT ( 'NONE',  ( 233.9782151781249411, -31.30312499938547788, -52.38713871227520968 ) ) ;
#18079=ORIENTED_EDGE ( 'NONE', *, *, #5066, .F. ) ;
#18084=ORIENTED_EDGE ( 'NONE', *, *, #162, .F. ) ;
#18091=CARTESIAN_POINT ( 'NONE',  ( 232.5999999999999375, -33.71249999999999147, 96.99999999999998579 ) ) ;
#18092=( BOUNDED_CURVE ( )  B_SPLINE_CURVE ( 2, ( #13822, #4954, #10896, #3470, #6515, #14208, #944, #6900, #6991 ),
 .UNSPECIFIED., .F., .F. ) 
 B_SPLINE_CURVE_WITH_KNOTS ( ( 3, 2, 2, 2, 3 ),
 ( 0.3958333333333333148, 0.4027777777777777901, 0.4166666666666666852, 0.4305555555555555802, 0.4374999999999999445 ),
 .UNSPECIFIED. ) 
 CURVE ( )  GEOMETRIC_REPRESENTATION_ITEM ( )  RATIONAL_B_SPLINE_CURVE ( ( 0.9330127018922194093, 0.9330127018922190762, 1.000000000000000000, 0.8660254037844387076, 1.000000000000000000, 0.8660254037844387076, 1.000000000000000000, 0.9330127018922198534, 0.9330127018922192983 ) ) 
 REPRESENTATION_ITEM ( '' )  );
#18094=CARTESIAN_POINT ( 'NONE',  ( 232.5999999999999375, -33.26249999999999574, 97.00000000000000000 ) ) ;
#18098=CARTESIAN_POINT ( 'NONE',  ( 233.9782151781249411, -31.64062499938547646, 97.61286128772489690 ) ) ;
#18101=CARTESIAN_POINT ( 'NONE',  ( 234.0999999999999375, -32.54999999999999716, -47.40192378864679768 ) ) ;
#18105=CARTESIAN_POINT ( 'NONE',  ( 231.2217848218749339, -34.71562499938547575, -52.38713871227520968 ) ) ;
#18113=CARTESIAN_POINT ( 'NONE',  ( 231.2217848218749339, -32.76562499938548001, 102.3871387122750889 ) ) ;
#18118=CARTESIAN_POINT ( 'NONE',  ( 231.0999999999999375, -32.77499999999999147, -52.59807621135342970 ) ) ;
#18123=ADVANCED_FACE ( 'NONE', ( #10199 ), #16063, .T. ) ;
#18124=CARTESIAN_POINT ( 'NONE',  ( 232.5999999999999375, -32.16562499938547859, -53.18285161636690361 ) ) ;
#18132=CARTESIAN_POINT ( 'NONE',  ( 232.5999999999999659, -32.13749999999999574, 102.9999999999999858 ) ) ;
#18136=CARTESIAN_POINT ( 'NONE',  ( 235.3564303562499447, -31.71562499938547575, -50.00000000000011369 ) ) ;
#18145=CARTESIAN_POINT ( 'NONE',  ( 232.5999999999999659, -32.53124999877096712, 103.0000000000000000 ) ) ;
#18146=ORIENTED_EDGE ( 'NONE', *, *, #17135, .T. ) ;
#18151=CARTESIAN_POINT ( 'NONE',  ( 234.0999999999999375, -32.79374999877096286, -52.59807621135342970 ) ) ;
#18152=CARTESIAN_POINT ( 'NONE',  ( 229.8435696437499303, -34.75312499938547717, 99.99999999999998579 ) ) ;
#18164=CARTESIAN_POINT ( 'NONE',  ( 233.9782151781249411, -33.70312499938548001, -47.61286128772501769 ) ) ;
#18166=CARTESIAN_POINT ( 'NONE',  ( 235.3564303562499447, -30.96562499938547930, 101.5914258081833879 ) ) ;
#18167=CARTESIAN_POINT ( 'NONE',  ( 235.3564303562499447, -30.44062499938548072, -51.59142580818350865 ) ) ;
#18171=CARTESIAN_POINT ( 'NONE',  ( 231.0999999999999375, -32.56874999877096144, -47.40192378864679768 ) ) ;
#18172=CARTESIAN_POINT ( 'NONE',  ( 231.7961524227065979, -34.85759618943232852, 103.0000000000000000 ) ) ;
#18187=CARTESIAN_POINT ( 'NONE',  ( 232.5999999999999375, -32.50312499938547717, 96.81714838363319586 ) ) ;
#18188=ORIENTED_EDGE ( 'NONE', *, *, #15209, .F. ) ;
#18191=DIRECTION ( 'NONE',  ( -4.625929269271485174E-17, -1.000000000000000000, 0.000000000000000000 ) ) ;
#18197=CARTESIAN_POINT ( 'NONE',  ( 231.7960411235079050, -35.00000000000002132, -47.36341917746382535 ) ) ;
#18200=ORIENTED_EDGE ( 'NONE', *, *, #16679, .F. ) ;
#18207=AXIS2_PLACEMENT_3D ( 'NONE', #8393, #1167, #17485 ) ;
#18208=CARTESIAN_POINT ( 'NONE',  ( 229.8435696437499871, -32.80312499938548143, 101.5914258081833879 ) ) ;
#18213=CARTESIAN_POINT ( 'NONE',  ( 232.5999999999999375, -31.68749999999999289, -46.53589838486234953 ) ) ;
#18217=FACE_OUTER_BOUND ( 'NONE', #3504, .T. ) ;
#18219=CARTESIAN_POINT ( 'NONE',  ( 231.2217848218749339, -34.22812499938548569, -47.61286128772501769 ) ) ;
#18223=CARTESIAN_POINT ( 'NONE',  ( 232.3466685930879123, -34.99995246259152282, 97.01071553687879145 ) ) ;
#18225=DIRECTION ( 'NONE',  ( -0.000000000000000000, -1.000000000000000000, -0.000000000000000000 ) ) ;
#18232=CARTESIAN_POINT ( 'NONE',  ( 235.3564303562499447, -30.85312499938547859, -48.40857419181671162 ) ) ;
#18237=CARTESIAN_POINT ( 'NONE',  ( 235.5999999999999375, -34.27499999999999147, 99.99999999999998579 ) ) ;
#18247=CARTESIAN_POINT ( 'NONE',  ( 235.5999999999999943, -32.90624999877096002, -48.26794919243124582 ) ) ;
#18248=CARTESIAN_POINT ( 'NONE',  ( 233.9782151781249411, -35.05312499938548143, 102.3871387122750889 ) ) ;
#18250=ORIENTED_EDGE ( 'NONE', *, *, #12736, .T. ) ;
#18259=CARTESIAN_POINT ( 'NONE',  ( 229.5999999999999375, -34.94999999999999574, 99.99999999999998579 ) ) ;
#18261=CARTESIAN_POINT ( 'NONE',  ( 229.8435696437499587, -33.44062499938547717, -51.59142580818350154 ) ) ;
#18263=CARTESIAN_POINT ( 'NONE',  ( 235.3564303562499447, -32.24062499938548143, 98.40857419181659793 ) ) ;
#18264=CARTESIAN_POINT ( 'NONE',  ( 235.5999999999999943, -35.08124999877096428, -51.73205080756900287 ) ) ;
#18268=CARTESIAN_POINT ( 'NONE',  ( 244.7999999999999545, -32.00000000000000000, -100.0000000000000000 ) ) ;
#18270=CARTESIAN_POINT ( 'NONE',  ( 102.9999999999999858, -5.200000000000008171, -100.0000000000000000 ) ) ;
#18281=CARTESIAN_POINT ( 'NONE',  ( 232.5999999999999375, -34.55624999877095860, -53.00000000000011369 ) ) ;
#18282=CARTESIAN_POINT ( 'NONE',  ( 233.9782151781249411, -33.89062499938548001, 97.61286128772489690 ) ) ;
#18283=CARTESIAN_POINT ( 'NONE',  ( 229.8435696437499303, -32.84062499938547575, 99.99999999999998579 ) ) ;
#18292=CARTESIAN_POINT ( 'NONE',  ( 232.5999999999999375, -34.07812499938548001, -46.81714838363331666 ) ) ;
#18294=ORIENTED_EDGE ( 'NONE', *, *, #6132, .F. ) ;
#18301=VECTOR ( 'NONE', #18835, 1000.000000000000000 ) ;
#18307=CARTESIAN_POINT ( 'NONE',  ( 235.5999999999999943, -32.51249999999998863, -48.26794919243124582 ) ) ;
#18312=CARTESIAN_POINT ( 'NONE',  ( 229.8435696437499587, -32.99062499938548143, 98.40857419181659793 ) ) ;
#18314=CARTESIAN_POINT ( 'NONE',  ( 231.2217848218749339, -32.87812499938547717, -47.61286128772501769 ) ) ;
#18316=ORIENTED_EDGE ( 'NONE', *, *, #175, .T. ) ;
#18322=CARTESIAN_POINT ( 'NONE',  ( 230.4677467024383475, -31.99999999999998579, -51.75590051601145092 ) ) ;
#18325=AXIS2_PLACEMENT_3D ( 'NONE', #7913, #14157, #9372 ) ;
#18330=CARTESIAN_POINT ( 'NONE',  ( 234.0999999999999375, -32.99999999999999289, -47.40192378864679768 ) ) ;
#18335=( NAMED_UNIT ( * ) SI_UNIT ( $, .STERADIAN. ) SOLID_ANGLE_UNIT ( ) );
#18337=CARTESIAN_POINT ( 'NONE',  ( 232.5999999999999375, -33.48749999999999716, 103.0000000000000000 ) ) ;
#18338=ORIENTED_EDGE ( 'NONE', *, *, #1500, .F. ) ;
#18341=DIRECTION ( 'NONE',  ( 1.000000000000000000, -0.000000000000000000, -0.000000000000000000 ) ) ;
#18343=FACE_OUTER_BOUND ( 'NONE', #10097, .T. ) ;
#18345=CARTESIAN_POINT ( 'NONE',  ( 233.9782151781249411, -33.10312499938547859, 97.61286128772489690 ) ) ;
#18348=LINE ( 'NONE', #4971, #18988 ) ;
#18349=CARTESIAN_POINT ( 'NONE',  ( 232.5999999999999375, -32.75624999877096144, -53.00000000000010658 ) ) ;
#18357=CARTESIAN_POINT ( 'NONE',  ( 235.3564303562499163, -34.98839802032724577, -49.56403331587380023 ) ) ;
#18359=CARTESIAN_POINT ( 'NONE',  ( 231.2217848218749339, -32.12812499938547717, 97.61286128772489690 ) ) ;
#18360=CARTESIAN_POINT ( 'NONE',  ( 229.8435696437499871, -31.64062499938547290, -51.59142580818350865 ) ) ;
#18368=DIRECTION ( 'NONE',  ( 0.000000000000000000, 0.000000000000000000, -1.000000000000000000 ) ) ;
#18374=( BOUNDED_SURFACE ( )  B_SPLINE_SURFACE ( 1, 2, ( 
 ( #8061, #7960, #9523, #7668, #13724, #4949, #15099, #15190, #15489, #5136, #3270, #12268, #365, #10891, #9226, #6314, #12548, #13914, #4849, #18232, #10983, #12362, #16859, #1903, #552, #18519, #6510, #7865, #14016, #13624, #652, #16574, #16756, #3174, #3464, #16952, #9134, #18421, #3564, #1714, #12168, #3372, #18136, #4756, #10699, #9324, #13816, #459, #13034, #17342, #8159, #3663, #6700, #2198, #1032, #3952, #9720, #15879, #15778, #12644, #6895, #5340, #6985, #14108, #12844, #745, #17246, #18813, #17442, #15686, #2290, #8254, #5527, #11081, #2387, #8441, #17148, #18618, #841, #14204, #4053, #5437, #6804, #10012, #9627, #11376, #18719, #5236, #9917, #12750, #15589, #15970, #11185, #2483, #12936, #3755, #1118, #11278, #3853, #9816, #8349, #18908, #14303, #14394, #939, #14487, #11475, #2576, #8537, #7078, #19005, #17051, #4245, #11666, #51, #4341, #11855, #7556, #6002, #1219, #10393, #7363, #2871, #13421, #13320, #19296, #16355, #16452, #10303, #10202, #5909, #17823, #4435, #16261, #16166, #11571, #17630 ),
 ( #10489, #2777, #14588, #8828, #14785, #8630, #2965, #8920, #11952, #5810, #13513, #7175, #14882, #17922, #8730, #14684, #16065, #1319, #3062, #1512, #4531, #2670, #7267, #7461, #4149, #13222, #9024, #5625, #19194, #11760, #17734, #14983, #1411, #1607, #17534, #10110, #13125, #19095, #5716, #9308, #1886, #4833, #12343, #15470, #16843, #18213, #10966, #10588, #12437, #16936, #12150, #3546, #7844, #13894, #9502, #15368, #9404, #6387, #18405, #244, #8037, #2080, #3449, #1984, #5025, #13799, #150, #18307, #16553, #12049, #15077, #3152, #7942, #4927, #18118, #10872, #10774, #1696, #15271, #13708, #532, #9115, #442, #7648, #6295, #6485, #6101, #18025, #4638, #13603, #6203, #4732, #10677, #16738, #16647, #3248, #9206, #15171, #1788, #3348, #7753, #348, #12246, #15759, #5318, #5215, #633, #730, #15950, #11163, #12730, #2367, #17322, #823, #18502, #14376, #11457, #3931, #9897, #3642, #6683, #2551, #14186, #6968, #12626, #6781, #18599, #1012, #18789, #12919, #4034, #11061, #17223, #14283, #920, #8138, #5510 ) ),
 .UNSPECIFIED., .F., .F., .F. ) 
 B_SPLINE_SURFACE_WITH_KNOTS ( ( 2, 2 ),
 ( 3, 2, 2, 2, 2, 2, 2, 2, 2, 2, 2, 2, 2, 2, 2, 2, 2, 2, 2, 2, 2, 2, 2, 2, 2, 2, 2, 2, 2, 2, 2, 2, 2, 2, 2, 2, 2, 2, 2, 2, 2, 2, 2, 2, 2, 2, 2, 2, 2, 2, 2, 2, 2, 2, 2, 2, 2, 2, 2, 2, 2, 2, 2, 2, 2, 2, 2, 2, 3 ),
 ( 0.000000000000000000, 1.000000000000000000 ),
 ( 0.000000000000000000, 0.01388888888888888812, 0.02777777777777777624, 0.04166666666666666435, 0.05555555555555555247, 0.06944444444444444753, 0.08333333333333332871, 0.09722222222222222376, 0.1111111111111111049, 0.1250000000000000000, 0.1388888888888888951, 0.1527777777777777901, 0.1666666666666666574, 0.1805555555555555525, 0.1944444444444444475, 0.2083333333333333426, 0.2222222222222222099, 0.2361111111111111049, 0.2500000000000000000, 0.2638888888888888951, 0.2777777777777777901, 0.2916666666666666852, 0.3055555555555555802, 0.3194444444444444198, 0.3333333333333333148, 0.3472222222222222099, 0.3611111111111111049, 0.3750000000000000000, 0.3888888888888888951, 0.4027777777777777901, 0.4166666666666666852, 0.4305555555555555802, 0.4444444444444444198, 0.4583333333333333148, 0.4722222222222222099, 0.4861111111111111049, 0.5000000000000000000, 0.5138888888888888395, 0.5277777777777777901, 0.5416666666666666297, 0.5555555555555555802, 0.5694444444444444198, 0.5833333333333333703, 0.5972222222222222099, 0.6111111111111111605, 0.6250000000000000000, 0.6388888888888888395, 0.6527777777777777901, 0.6666666666666666297, 0.6805555555555555802, 0.6944444444444444198, 0.7083333333333333703, 0.7222222222222222099, 0.7361111111111111605, 0.7500000000000000000, 0.7638888888888888395, 0.7777777777777777901, 0.7916666666666666297, 0.8055555555555555802, 0.8194444444444444198, 0.8333333333333333703, 0.8472222222222222099, 0.8611111111111111605, 0.8750000000000000000, 0.8888888888888888395, 0.9027777777777777901, 0.9166666666666666297, 0.9258785066912882389, 0.9351372917582011501 ),
 .UNSPECIFIED. ) 
 GEOMETRIC_REPRESENTATION_ITEM ( )  RATIONAL_B_SPLINE_SURFACE ( (
 ( 1.000000000000000000, 0.8660254037844387076, 1.000000000000000000, 0.8660254037844387076, 1.000000000000000000, 0.8660254037844387076, 1.000000000000000000, 0.8660254037844387076, 1.000000000000000000, 0.8660254037844387076, 1.000000000000000000, 0.8660254037844387076, 1.000000000000000000, 0.8660254037844387076, 1.000000000000000000, 0.8660254037844387076, 1.000000000000000000, 0.8660254037844387076, 1.000000000000000000, 0.8660254037844387076, 1.000000000000000000, 0.8660254037844387076, 1.000000000000000000, 0.8660254037844387076, 1.000000000000000000, 0.8660254037844387076, 1.000000000000000000, 0.8660254037844387076, 1.000000000000000000, 0.8660254037844387076, 1.000000000000000000, 0.8660254037844387076, 1.000000000000000000, 0.8660254037844387076, 1.000000000000000000, 0.8660254037844387076, 1.000000000000000000, 0.8660254037844387076, 1.000000000000000000, 0.8660254037844387076, 1.000000000000000000, 0.8660254037844387076, 1.000000000000000000, 0.8660254037844387076, 1.000000000000000000, 0.8660254037844387076, 1.000000000000000000, 0.8660254037844387076, 1.000000000000000000, 0.8660254037844387076, 1.000000000000000000, 0.8660254037844387076, 1.000000000000000000, 0.8660254037844387076, 1.000000000000000000, 0.8660254037844387076, 1.000000000000000000, 0.8660254037844387076, 1.000000000000000000, 0.8660254037844387076, 1.000000000000000000, 0.8660254037844387076, 1.000000000000000000, 0.8660254037844387076, 1.000000000000000000, 0.8660254037844387076, 1.000000000000000000, 0.8660254037844387076, 1.000000000000000000, 0.8660254037844387076, 1.000000000000000000, 0.8660254037844387076, 1.000000000000000000, 0.8660254037844387076, 1.000000000000000000, 0.8660254037844387076, 1.000000000000000000, 0.8660254037844387076, 1.000000000000000000, 0.8660254037844387076, 1.000000000000000000, 0.8660254037844387076, 1.000000000000000000, 0.8660254037844387076, 1.000000000000000000, 0.8660254037844387076, 1.000000000000000000, 0.8660254037844387076, 1.000000000000000000, 0.8660254037844387076, 1.000000000000000000, 0.8660254037844387076, 1.000000000000000000, 0.8660254037844387076, 1.000000000000000000, 0.8660254037844387076, 1.000000000000000000, 0.8660254037844387076, 1.000000000000000000, 0.8660254037844387076, 1.000000000000000000, 0.8660254037844387076, 1.000000000000000000, 0.8660254037844387076, 1.000000000000000000, 0.8660254037844387076, 1.000000000000000000, 0.8660254037844387076, 1.000000000000000000, 0.8660254037844387076, 1.000000000000000000, 0.8660254037844387076, 1.000000000000000000, 0.8660254037844387076, 1.000000000000000000, 0.8660254037844387076, 1.000000000000000000, 0.8660254037844387076, 1.000000000000000000, 0.8660254037844387076, 1.000000000000000000, 0.8660254037844387076, 1.000000000000000000, 0.8660254037844387076, 1.000000000000000000, 0.8660254037844387076, 1.000000000000000000, 0.8660254037844387076, 1.000000000000000000, 0.8660254037844387076, 1.000000000000000000, 0.8660254037844387076, 1.000000000000000000, 0.9111410165655264848, 0.9401539157124900736, 0.9401539157124900736, 0.9401539157124900736),
 ( 1.000000000000000000, 0.8660254037844387076, 1.000000000000000000, 0.8660254037844387076, 1.000000000000000000, 0.8660254037844387076, 1.000000000000000000, 0.8660254037844387076, 1.000000000000000000, 0.8660254037844387076, 1.000000000000000000, 0.8660254037844387076, 1.000000000000000000, 0.8660254037844387076, 1.000000000000000000, 0.8660254037844387076, 1.000000000000000000, 0.8660254037844387076, 1.000000000000000000, 0.8660254037844387076, 1.000000000000000000, 0.8660254037844387076, 1.000000000000000000, 0.8660254037844387076, 1.000000000000000000, 0.8660254037844387076, 1.000000000000000000, 0.8660254037844387076, 1.000000000000000000, 0.8660254037844387076, 1.000000000000000000, 0.8660254037844387076, 1.000000000000000000, 0.8660254037844387076, 1.000000000000000000, 0.8660254037844387076, 1.000000000000000000, 0.8660254037844387076, 1.000000000000000000, 0.8660254037844387076, 1.000000000000000000, 0.8660254037844387076, 1.000000000000000000, 0.8660254037844387076, 1.000000000000000000, 0.8660254037844387076, 1.000000000000000000, 0.8660254037844387076, 1.000000000000000000, 0.8660254037844387076, 1.000000000000000000, 0.8660254037844387076, 1.000000000000000000, 0.8660254037844387076, 1.000000000000000000, 0.8660254037844387076, 1.000000000000000000, 0.8660254037844387076, 1.000000000000000000, 0.8660254037844387076, 1.000000000000000000, 0.8660254037844387076, 1.000000000000000000, 0.8660254037844387076, 1.000000000000000000, 0.8660254037844387076, 1.000000000000000000, 0.8660254037844387076, 1.000000000000000000, 0.8660254037844387076, 1.000000000000000000, 0.8660254037844387076, 1.000000000000000000, 0.8660254037844387076, 1.000000000000000000, 0.8660254037844387076, 1.000000000000000000, 0.8660254037844387076, 1.000000000000000000, 0.8660254037844387076, 1.000000000000000000, 0.8660254037844387076, 1.000000000000000000, 0.8660254037844387076, 1.000000000000000000, 0.8660254037844387076, 1.000000000000000000, 0.8660254037844387076, 1.000000000000000000, 0.8660254037844387076, 1.000000000000000000, 0.8660254037844387076, 1.000000000000000000, 0.8660254037844387076, 1.000000000000000000, 0.8660254037844387076, 1.000000000000000000, 0.8660254037844387076, 1.000000000000000000, 0.8660254037844387076, 1.000000000000000000, 0.8660254037844387076, 1.000000000000000000, 0.8660254037844387076, 1.000000000000000000, 0.8660254037844387076, 1.000000000000000000, 0.8660254037844387076, 1.000000000000000000, 0.8660254037844387076, 1.000000000000000000, 0.8660254037844387076, 1.000000000000000000, 0.8660254037844387076, 1.000000000000000000, 0.8660254037844387076, 1.000000000000000000, 0.8660254037844387076, 1.000000000000000000, 0.8660254037844387076, 1.000000000000000000, 0.8660254037844387076, 1.000000000000000000, 0.8660254037844387076, 1.000000000000000000, 0.8660254037844387076, 1.000000000000000000, 0.8660254037844387076, 1.000000000000000000, 0.8660254037844387076, 1.000000000000000000, 0.8660254037844387076, 1.000000000000000000, 0.9111410165655264848, 0.9401539157124900736, 0.9401539157124900736, 0.9401539157124900736) ) ) 
 REPRESENTATION_ITEM ( '' )  SURFACE ( )  );
#18378=DIRECTION ( 'NONE',  ( 1.000000000000000000, 0.000000000000000000, 0.000000000000000000 ) ) ;
#18380=CARTESIAN_POINT ( 'NONE',  ( 231.2217848218749339, -34.11562499938548143, 102.3871387122750889 ) ) ;
#18382=SURFACE_STYLE_USAGE ( .BOTH. , #9090 ) ;
#18383=CARTESIAN_POINT ( 'NONE',  ( 235.5999999999999943, -31.03124999877096357, 98.26794919243110371 ) ) ;
#18385=ORIENTED_EDGE ( 'NONE', *, *, #6183, .T. ) ;
#18389=CARTESIAN_POINT ( 'NONE',  ( 229.7688980899055196, -35.00000000000000000, -50.85751801881856693 ) ) ;
#18391=CARTESIAN_POINT ( 'NONE',  ( 231.2217848218749339, -34.56562499938547717, -47.61286128772501769 ) ) ;
#18394=CARTESIAN_POINT ( 'NONE',  ( 234.0999999999999375, -33.44999999999999574, -47.40192378864679768 ) ) ;
#18401=DIRECTION ( 'NONE',  ( 1.000000000000000000, 0.000000000000000000, -0.000000000000000000 ) ) ;
#18405=CARTESIAN_POINT ( 'NONE',  ( 231.0999999999999375, -32.17499999999999716, -47.40192378864679768 ) ) ;
#18408=CARTESIAN_POINT ( 'NONE',  ( 231.2217848218749339, -32.12812499938547717, 97.61286128772489690 ) ) ;
#18410=CARTESIAN_POINT ( 'NONE',  ( 229.8435696437499871, -32.54062499938547859, -51.59142580818350865 ) ) ;
#18412=VERTEX_POINT ( 'NONE', #629 ) ;
#18421=CARTESIAN_POINT ( 'NONE',  ( 229.8435696437499871, -31.52812499938547575, -51.59142580818350865 ) ) ;
#18424=ORIENTED_EDGE ( 'NONE', *, *, #7530, .T. ) ;
#18438=EDGE_CURVE ( 'NONE', #7254, #15345, #15659, .T. ) ;
#18439=CARTESIAN_POINT ( 'NONE',  ( 229.8435696437499303, -35.20312499938548001, 99.99999999999998579 ) ) ;
#18444=DIRECTION ( 'NONE',  ( -0.000000000000000000, -1.000000000000000000, -0.000000000000000000 ) ) ;
#18452=CARTESIAN_POINT ( 'NONE',  ( 229.8435696437499303, -32.95312499938548001, 99.99999999999998579 ) ) ;
#18453=CARTESIAN_POINT ( 'NONE',  ( 229.8435696437499871, -31.11562499938547788, -48.40857419181671162 ) ) ;
#18462=CARTESIAN_POINT ( 'NONE',  ( 232.5999999999999375, -34.55624999877095860, 97.00000000000000000 ) ) ;
#18463=ORIENTED_EDGE ( 'NONE', *, *, #8045, .T. ) ;
#18471=CARTESIAN_POINT ( 'NONE',  ( 244.7999999999999545, -32.00000000000001421, -103.0000000000000142 ) ) ;
#18472=CARTESIAN_POINT ( 'NONE',  ( 229.8435696437499871, -33.32812499938548001, 98.40857419181659793 ) ) ;
#18473=ORIENTED_EDGE ( 'NONE', *, *, #6395, .T. ) ;
#18474=CARTESIAN_POINT ( 'NONE',  ( 231.0999999999999375, -30.76874999877096428, 102.5980762113533018 ) ) ;
#18478=CARTESIAN_POINT ( 'NONE',  ( 244.7999999999999545, -35.00000000000002842, 147.7999999999999829 ) ) ;
#18484=AXIS2_PLACEMENT_3D ( 'NONE', #18678, #17108, #6949 ) ;
#18485=CARTESIAN_POINT ( 'NONE',  ( 233.4038475772933339, -33.86115380933863150, -47.00000000000012790 ) ) ;
#18490=DIRECTION ( 'NONE',  ( -0.000000000000000000, -1.000000000000000000, -0.000000000000000000 ) ) ;
#18502=CARTESIAN_POINT ( 'NONE',  ( 235.5999999999999375, -34.27499999999999147, -50.00000000000011369 ) ) ;
#18507=CARTESIAN_POINT ( 'NONE',  ( 231.2217848218749339, -32.12812499938547717, -52.38713871227520968 ) ) ;
#18509=ORIENTED_EDGE ( 'NONE', *, *, #4830, .T. ) ;
#18519=CARTESIAN_POINT ( 'NONE',  ( 229.8435696437499871, -31.07812499938548001, -51.59142580818350865 ) ) ;
#18524=CARTESIAN_POINT ( 'NONE',  ( 232.5999999999999375, -33.88124999877096855, -47.00000000000011369 ) ) ;
#18525=CARTESIAN_POINT ( 'NONE',  ( 105.1999999999999744, -34.99999999999999289, -100.0000000000000000 ) ) ;
#18529=EDGE_LOOP ( 'NONE', ( #11624, #17944, #13442, #9186, #1061, #13657 ) ) ;
#18534=CARTESIAN_POINT ( 'NONE',  ( 229.8435696437499871, -33.89062499938548001, 98.40857419181659793 ) ) ;
#18547=CARTESIAN_POINT ( 'NONE',  ( 229.8435696437499871, -32.09062499938548285, 98.40857419181659793 ) ) ;
#18548=CARTESIAN_POINT ( 'NONE',  ( 235.3564303562499447, -34.07812499938548001, -50.00000000000011369 ) ) ;
#18550=EDGE_CURVE ( 'NONE', #8999, #15031, #11452, .T. ) ;
#18570=CARTESIAN_POINT ( 'NONE',  ( 233.9782151781249411, -34.34062499938547575, 97.61286128772489690 ) ) ;
#18575=CARTESIAN_POINT ( 'NONE',  ( 231.0999999999999375, -31.36874999877096215, 97.40192378864668399 ) ) ;
#18576=CARTESIAN_POINT ( 'NONE',  ( 232.5999999999999375, -32.30624999877096570, 97.00000000000000000 ) ) ;
#18577=EDGE_LOOP ( 'NONE', ( #5739, #5842, #8597, #13082 ) ) ;
#18591=CARTESIAN_POINT ( 'NONE',  ( 105.1999999999999744, -31.99999999999999289, 150.0000000000000000 ) ) ;
#18598=VERTEX_POINT ( 'NONE', #7152 ) ;
#18599=CARTESIAN_POINT ( 'NONE',  ( 235.5999999999999375, -34.72499999999999432, -50.00000000000011369 ) ) ;
#18604=CARTESIAN_POINT ( 'NONE',  ( 235.3564303562499447, -32.24062499938548143, 98.40857419181659793 ) ) ;
#18606=CARTESIAN_POINT ( 'NONE',  ( 229.8435696437499871, -35.16562499938547148, -48.40857419181671162 ) ) ;
#18607=VERTEX_POINT ( 'NONE', #4030 ) ;
#18618=CARTESIAN_POINT ( 'NONE',  ( 235.3564303562499447, -33.02812499938547575, -51.59142580818350865 ) ) ;
#18621=ORIENTED_EDGE ( 'NONE', *, *, #16631, .T. ) ;
#18633=CARTESIAN_POINT ( 'NONE',  ( 235.3564303562499447, -30.85312499938547859, 101.5914258081833879 ) ) ;
#18639=VECTOR ( 'NONE', #11742, 1000.000000000000000 ) ;
#18640=CARTESIAN_POINT ( 'NONE',  ( 231.7961524227065695, -34.80134618820329706, -47.00000000000011369 ) ) ;
#18644=( BOUNDED_CURVE ( )  B_SPLINE_CURVE ( 2, ( #11619, #8782, #5862, #11815, #15926, #2528, #16313, #1174, #4391 ),
 .UNSPECIFIED., .F., .F. ) 
 B_SPLINE_CURVE_WITH_KNOTS ( ( 3, 2, 2, 2, 3 ),
 ( 0.7708333333333332593, 0.7777777777777777901, 0.7916666666666666297, 0.8055555555555555802, 0.8125000000000000000 ),
 .UNSPECIFIED. ) 
 CURVE ( )  GEOMETRIC_REPRESENTATION_ITEM ( )  RATIONAL_B_SPLINE_CURVE ( ( 0.9330127018922192983, 0.9330127018922187432, 1.000000000000000000, 0.8660254037844387076, 1.000000000000000000, 0.8660254037844387076, 1.000000000000000000, 0.9330127018922194093, 0.9330127018922194093 ) ) 
 REPRESENTATION_ITEM ( '' )  );
#18646=PRODUCT_CONTEXT ( 'NONE', #4709, 'mechanical' ) ;
#18647=CARTESIAN_POINT ( 'NONE',  ( 232.5999999999999375, -32.39062499938548001, 103.1828516163667899 ) ) ;
#18648=CARTESIAN_POINT ( 'NONE',  ( 235.3564303562499447, -32.72812499938547859, -50.00000000000011369 ) ) ;
#18656=CARTESIAN_POINT ( 'NONE',  ( 105.1999999999999744, -4.999999999999976907, 153.0000000000000000 ) ) ;
#18662=CARTESIAN_POINT ( 'NONE',  ( 229.8435696437499871, -30.29062499938548214, 98.40857419181659793 ) ) ;
#18665=CIRCLE ( 'NONE', #1800, 5.200000000000009948 ) ;
#18669=CARTESIAN_POINT ( 'NONE',  ( 235.5999999999999943, -32.45624999877096428, 101.7320508075688537 ) ) ;
#18670=CARTESIAN_POINT ( 'NONE',  ( 231.2583267490322783, -32.00000000000000000, 102.4658751321104120 ) ) ;
#18671=CARTESIAN_POINT ( 'NONE',  ( 235.3564303562499447, -33.55312499938548143, 101.5914258081833879 ) ) ;
#18674=CARTESIAN_POINT ( 'NONE',  ( 234.0999999999999375, -31.59374999877096712, 102.5980762113533018 ) ) ;
#18675=CARTESIAN_POINT ( 'NONE',  ( 229.5999999999999375, -31.70624999877096073, -48.26794919243123161 ) ) ;
#18678=CARTESIAN_POINT ( 'NONE',  ( 232.5999999999999375, -29.99999999999999645, 99.99999999999998579 ) ) ;
#18681=AXIS2_PLACEMENT_3D ( 'NONE', #1051, #11302, #19023 ) ;
#18697=VECTOR ( 'NONE', #15804, 1000.000000000000000 ) ;
#18703=CARTESIAN_POINT ( 'NONE',  ( 233.9782151781249411, -32.80312499938548143, 102.3871387122750889 ) ) ;
#18705=CARTESIAN_POINT ( 'NONE',  ( 229.8435696437499871, -30.17812499938547433, -51.59142580818350865 ) ) ;
#18709=CYLINDRICAL_SURFACE ( 'NONE', #14404, 5.200000000000009948 ) ;
#18711=CARTESIAN_POINT ( 'NONE',  ( 229.5999999999999375, -33.13124999877096144, -51.73205080756898866 ) ) ;
#18712=DIRECTION ( 'NONE',  ( -0.000000000000000000, -1.000000000000000000, 0.000000000000000000 ) ) ;
#18718=EDGE_CURVE ( 'NONE', #15440, #2968, #15146, .T. ) ;
#18719=CARTESIAN_POINT ( 'NONE',  ( 231.2217848218749339, -33.36562499938548143, -52.38713871227520968 ) ) ;
#18723=CARTESIAN_POINT ( 'NONE',  ( 234.0999999999999375, -34.14374999877096428, -52.59807621135342970 ) ) ;
#18735=EDGE_CURVE ( 'NONE', #8905, #4556, #7723, .T. ) ;
#18744=VERTEX_POINT ( 'NONE', #18281 ) ;
#18747=CARTESIAN_POINT ( 'NONE',  ( 235.3564303562499447, -34.56562499938547717, 101.5914258081833879 ) ) ;
#18748=CARTESIAN_POINT ( 'NONE',  ( 235.3564303562499447, -33.17812499938548143, -50.00000000000011369 ) ) ;
#18763=CARTESIAN_POINT ( 'NONE',  ( 234.0999999999999375, -31.49999999999999289, 97.40192378864668399 ) ) ;
#18766=CARTESIAN_POINT ( 'NONE',  ( 232.5999999999999375, -33.88124999877096144, 103.4641016151377499 ) ) ;
#18767=CARTESIAN_POINT ( 'NONE',  ( 232.5999999999999375, -30.73124999877096286, -46.53589838486234953 ) ) ;
#18772=FACE_OUTER_BOUND ( 'NONE', #4952, .T. ) ;
#18773=EDGE_LOOP ( 'NONE', ( #10945, #2010, #7978, #8919 ) ) ;
#18777=DIRECTION ( 'NONE',  ( 0.000000000000000000, -6.672013369141570147E-16, 1.000000000000000000 ) ) ;
#18782=CARTESIAN_POINT ( 'NONE',  ( 235.3288510558096789, -34.99999999999999289, -50.77688434087658464 ) ) ;
#18783=CARTESIAN_POINT ( 'NONE',  ( 231.4797793666090229, -31.99999999999997868, -52.57317574659983705 ) ) ;
#18789=CARTESIAN_POINT ( 'NONE',  ( 234.0999999999999375, -34.79999999999999716, -47.40192378864679768 ) ) ;
#18795=CARTESIAN_POINT ( 'NONE',  ( 235.3564303562499447, -34.11562499938548143, 101.5914258081833879 ) ) ;
#18797=CARTESIAN_POINT ( 'NONE',  ( 235.3564303562499447, -30.85312499938547859, -48.40857419181671162 ) ) ;
#18813=CARTESIAN_POINT ( 'NONE',  ( 235.3564303562499447, -32.65312499938547575, -48.40857419181671162 ) ) ;
#18818=ORIENTED_EDGE ( 'NONE', *, *, #3851, .F. ) ;
#18827=CARTESIAN_POINT ( 'NONE',  ( 235.3564303562499447, -32.57812499938548001, 98.40857419181659793 ) ) ;
#18829=ADVANCED_FACE ( 'NONE', ( #9183 ), #12217, .F. ) ;
#18835=DIRECTION ( 'NONE',  ( 0.000000000000000000, 0.000000000000000000, 1.000000000000000000 ) ) ;
#18842=CARTESIAN_POINT ( 'NONE',  ( 235.3564303562499447, -34.52812499938547575, 99.99999999999998579 ) ) ;
#18844=CARTESIAN_POINT ( 'NONE',  ( 231.2217848218749339, -32.57812499938548001, -52.38713871227520968 ) ) ;
#18850=ORIENTED_EDGE ( 'NONE', *, *, #1016, .T. ) ;
#18860=CARTESIAN_POINT ( 'NONE',  ( 233.5505106857032445, -35.00000000000000711, 102.5934467159355421 ) ) ;
#18862=CARTESIAN_POINT ( 'NONE',  ( 232.5999999999999375, -31.46249999999999858, 96.53589838486223584 ) ) ;
#18865=CARTESIAN_POINT ( 'NONE',  ( 231.0999999999999375, -32.26874999877096428, 97.40192378864668399 ) ) ;
#18866=FACE_OUTER_BOUND ( 'NONE', #381, .T. ) ;
#18873=CARTESIAN_POINT ( 'NONE',  ( 229.5999999999999375, -33.13124999877096144, 98.26794919243111792 ) ) ;
#18880=CARTESIAN_POINT ( 'NONE',  ( 235.2646886264966497, -35.00000000000002132, -51.00543742925584212 ) ) ;
#18881=CARTESIAN_POINT ( 'NONE',  ( 234.9223452063436639, -32.00000000000001421, -51.84871274668164176 ) ) ;
#18888=CARTESIAN_POINT ( 'NONE',  ( 246.9999999999999716, -5.000000000000004441, 150.0000000000000000 ) ) ;
#18895=CARTESIAN_POINT ( 'NONE',  ( 230.4884518427504076, -35.25364861271050643, -51.77179927996177611 ) ) ;
#18898=LINE ( 'NONE', #12836, #14729 ) ;
#18900=CARTESIAN_POINT ( 'NONE',  ( 105.1999999999999744, -4.999999999999976907, 150.0000000000000000 ) ) ;
#18906=EDGE_CURVE ( 'NONE', #13209, #3413, #6212, .T. ) ;
#18908=CARTESIAN_POINT ( 'NONE',  ( 235.3564303562499447, -33.92812499938548143, -51.59142580818350865 ) ) ;
#18911=ORIENTED_EDGE ( 'NONE', *, *, #2906, .T. ) ;
#18913=CARTESIAN_POINT ( 'NONE',  ( 232.5999999999999375, -34.33124999877097139, -47.00000000000011369 ) ) ;
#18919=EDGE_CURVE ( 'NONE', #5195, #10996, #8557, .T. ) ;
#18921=CARTESIAN_POINT ( 'NONE',  ( 231.2217848218749339, -32.01562499938548001, 97.61286128772489690 ) ) ;
#18922=CARTESIAN_POINT ( 'NONE',  ( 232.5999999999999375, -29.99999999999999645, 103.0000000000000000 ) ) ;
#18930=LINE ( 'NONE', #13057, #6475 ) ;
#18938=CARTESIAN_POINT ( 'NONE',  ( 232.5999999999999375, -33.51562499938548001, -53.18285161636690361 ) ) ;
#18941=VERTEX_POINT ( 'NONE', #13058 ) ;
#18943=DIRECTION ( 'NONE',  ( 1.000000000000000000, 0.000000000000000000, 0.000000000000000000 ) ) ;
#18954=CARTESIAN_POINT ( 'NONE',  ( 233.0319854768594041, -35.00000000000000000, 102.7281823352557097 ) ) ;
#18957=CARTESIAN_POINT ( 'NONE',  ( 235.5999999999999943, -32.06249999999999289, 101.7320508075688537 ) ) ;
#18958=VERTEX_POINT ( 'NONE', #6918 ) ;
#18962=CARTESIAN_POINT ( 'NONE',  ( 229.5999999999999375, -33.09374999877096002, 99.99999999999998579 ) ) ;
#18963=CARTESIAN_POINT ( 'NONE',  ( 234.0999999999999375, -30.99374999877096215, -52.59807621135342970 ) ) ;
#18964=CARTESIAN_POINT ( 'NONE',  ( 231.0999999999999375, -34.57499999999999574, 97.40192378864668399 ) ) ;
#18966=AXIS2_PLACEMENT_3D ( 'NONE', #10875, #12346, #732 ) ;
#18970=VERTEX_POINT ( 'NONE', #505 ) ;
#18977=CARTESIAN_POINT ( 'NONE',  ( 233.5509609210265296, -31.99999999999997868, -52.74042984513003063 ) ) ;
#18978=DIRECTION ( 'NONE',  ( 1.000000000000000000, -0.000000000000000000, -0.000000000000000000 ) ) ;
#18986=CARTESIAN_POINT ( 'NONE',  ( 232.5880334581522391, -34.99999999999999289, 97.00083539721710224 ) ) ;
#18988=VECTOR ( 'NONE', #10912, 1000.000000000000000 ) ;
#18990=CARTESIAN_POINT ( 'NONE',  ( 235.3564303562499447, -34.56562499938547717, 101.5914258081833879 ) ) ;
#18993=CARTESIAN_POINT ( 'NONE',  ( 229.8435696437499871, -34.79062499938547859, -51.59142580818350865 ) ) ;
#18999=CARTESIAN_POINT ( 'NONE',  ( 235.3564303562499447, -32.65312499938547575, 101.5914258081833879 ) ) ;
#19005=CARTESIAN_POINT ( 'NONE',  ( 231.2217848218749339, -34.26562499938548001, -52.38713871227520968 ) ) ;
#19015=DIRECTION ( 'NONE',  ( 0.000000000000000000, 0.000000000000000000, -1.000000000000000000 ) ) ;
#19016=CARTESIAN_POINT ( 'NONE',  ( 232.5999999999999943, -33.40312499938547575, 96.81714838363319586 ) ) ;
#19023=DIRECTION ( 'NONE',  ( 0.000000000000000000, 0.000000000000000000, -1.000000000000000000 ) ) ;
#19024=DIRECTION ( 'NONE',  ( -0.000000000000000000, -1.000000000000000000, -0.000000000000000000 ) ) ;
#19029=CARTESIAN_POINT ( 'NONE',  ( 233.9782151781249411, -34.60312499938548569, 102.3871387122750889 ) ) ;
#19030=CARTESIAN_POINT ( 'NONE',  ( 235.3564303562499447, -34.56562499938547717, -48.40857419181671162 ) ) ;
#19036=EDGE_CURVE ( 'NONE', #15781, #13743, #16366, .T. ) ;
#19046=CARTESIAN_POINT ( 'NONE',  ( 235.0940413310670465, -34.99999999999999289, 101.1871036926526557 ) ) ;
#19049=CARTESIAN_POINT ( 'NONE',  ( 229.5999999999999375, -30.93749999999999289, 98.26794919243111792 ) ) ;
#19051=ORIENTED_EDGE ( 'NONE', *, *, #7495, .T. ) ;
#19054=CARTESIAN_POINT ( 'NONE',  ( 231.0999999999999375, -31.81874999877096144, 97.40192378864668399 ) ) ;
#19055=CARTESIAN_POINT ( 'NONE',  ( 232.5999999999999375, -31.18124999877096215, -46.53589838486234953 ) ) ;
#19077=CARTESIAN_POINT ( 'NONE',  ( 235.2218879900010791, -34.99999999999999289, 100.8506536761482124 ) ) ;
#19079=CARTESIAN_POINT ( 'NONE',  ( 235.3564303562499447, -34.52812499938547575, 99.99999999999998579 ) ) ;
#19083=CARTESIAN_POINT ( 'NONE',  ( 235.3564303562499447, -33.10312499938547859, -48.40857419181671162 ) ) ;
#19090=CARTESIAN_POINT ( 'NONE',  ( 231.2217848218749339, -31.86562499938547788, 102.3871387122750889 ) ) ;
#19091=CARTESIAN_POINT ( 'NONE',  ( 229.8435696437499587, -32.87812499938547717, -51.59142580818350154 ) ) ;
#19095=CARTESIAN_POINT ( 'NONE',  ( 229.5999999999999375, -31.38749999999999218, -51.73205080756898866 ) ) ;
#19099=CARTESIAN_POINT ( 'NONE',  ( 232.5999999999999375, -29.99999999999999645, -50.00000000000011369 ) ) ;
#19100=DIRECTION ( 'NONE',  ( -0.000000000000000000, -0.000000000000000000, 1.000000000000000000 ) ) ;
#19101=CARTESIAN_POINT ( 'NONE',  ( 232.5999999999999375, -30.81562499938547717, -53.18285161636690361 ) ) ;
#19103=VERTEX_POINT ( 'NONE', #13143 ) ;
#19105=VECTOR ( 'NONE', #3310, 1000.000000000000000 ) ;
#19107=AXIS2_PLACEMENT_3D ( 'NONE', #15842, #6765, #2351 ) ;
#19108=CARTESIAN_POINT ( 'NONE',  ( 231.2217848218749339, -33.21562499938547575, 102.3871387122750889 ) ) ;
#19112=CARTESIAN_POINT ( 'NONE',  ( 233.5451393107506988, -32.00000000000000711, -47.24663084804295465 ) ) ;
#19123=CARTESIAN_POINT ( 'NONE',  ( 232.6775203606193543, -35.00000000000000000, -47.23891671615874088 ) ) ;
#19125=CARTESIAN_POINT ( 'NONE',  ( 235.5999999999999943, -34.18124999877096570, 98.26794919243110371 ) ) ;
#19133=VECTOR ( 'NONE', #11328, 1000.000000000000000 ) ;
#19136=CARTESIAN_POINT ( 'NONE',  ( 235.3564303562499447, -31.79062499938547859, 98.40857419181659793 ) ) ;
#19141=DIRECTION ( 'NONE',  ( 0.000000000000000000, 0.000000000000000000, 1.000000000000000000 ) ) ;
#19144=CARTESIAN_POINT ( 'NONE',  ( 232.5999999999999375, -32.13749999999998863, 103.4641016151377499 ) ) ;
#19145=EDGE_CURVE ( 'NONE', #8738, #13854, #17113, .T. ) ;
#19147=EDGE_LOOP ( 'NONE', ( #901, #10143, #2727, #1326 ) ) ;
#19150=CARTESIAN_POINT ( 'NONE',  ( 235.5999999999999943, -33.35624999877096997, 101.7320508075688537 ) ) ;
#19151=CARTESIAN_POINT ( 'NONE',  ( 235.5999999999999375, -34.21874999877096002, -50.00000000000011369 ) ) ;
#19158=EDGE_LOOP ( 'NONE', ( #2836, #8376, #7868, #14559, #9073, #5615 ) ) ;
#19161=CARTESIAN_POINT ( 'NONE',  ( 105.1999999999999744, -34.99999999999999289, -100.0000000000000000 ) ) ;
#19167=CARTESIAN_POINT ( 'NONE',  ( 99.99999999999997158, -5.200000000000008171, -100.0000000000000000 ) ) ;
#19168=EDGE_CURVE ( 'NONE', #8464, #11929, #6119, .T. ) ;
#19171=CARTESIAN_POINT ( 'NONE',  ( 235.3564303562499447, -30.77812499938547575, 98.40857419181659793 ) ) ;
#19176=CARTESIAN_POINT ( 'NONE',  ( 229.8435696437499303, -34.30312499938548143, 99.99999999999998579 ) ) ;
#19179=CARTESIAN_POINT ( 'NONE',  ( 233.9782151781249411, -33.89062499938548001, -52.38713871227520968 ) ) ;
#19180=ORIENTED_EDGE ( 'NONE', *, *, #15378, .F. ) ;
#19187=CARTESIAN_POINT ( 'NONE',  ( 232.5999999999999375, -30.92812499938547433, 103.1828516163667899 ) ) ;
#19188=CARTESIAN_POINT ( 'NONE',  ( 232.5999999999999943, -33.62812499938547717, -46.81714838363331666 ) ) ;
#19189=EDGE_CURVE ( 'NONE', #13951, #5496, #10991, .T. ) ;
#19190=EDGE_CURVE ( 'NONE', #10239, #8738, #12998, .T. ) ;
#19194=CARTESIAN_POINT ( 'NONE',  ( 234.0999999999999375, -31.04999999999999361, -52.59807621135342970 ) ) ;
#19198=APPLICATION_CONTEXT ( 'automotive_design' ) ;
#19202=CARTESIAN_POINT ( 'NONE',  ( 232.5999999999999375, -31.26562499938548356, -53.18285161636690361 ) ) ;
#19206=VECTOR ( 'NONE', #15403, 1000.000000000000000 ) ;
#19207=CARTESIAN_POINT ( 'NONE',  ( 235.3564303562499447, -32.16562499938547859, 99.99999999999998579 ) ) ;
#19212=FACE_OUTER_BOUND ( 'NONE', #6462, .T. ) ;
#19235=CARTESIAN_POINT ( 'NONE',  ( 231.2217848218749339, -30.77812499938548285, 97.61286128772489690 ) ) ;
#19242=CARTESIAN_POINT ( 'NONE',  ( 229.5999999999999375, -33.14999999999999147, 99.99999999999998579 ) ) ;
#19244=ORIENTED_EDGE ( 'NONE', *, *, #16994, .F. ) ;
#19245=FACE_OUTER_BOUND ( 'NONE', #19158, .T. ) ;
#19247=CARTESIAN_POINT ( 'NONE',  ( 232.5999999999999375, -34.78124999877096002, 103.4641016151377499 ) ) ;
#19248=CARTESIAN_POINT ( 'NONE',  ( 229.5999999999999375, -34.48124999877096286, -51.73205080756898866 ) ) ;
#19250=EDGE_LOOP ( 'NONE', ( #14375, #11336, #10280, #9944, #2533 ) ) ;
#19254=CARTESIAN_POINT ( 'NONE',  ( 232.5999999999999091, -34.38749999999999574, -47.00000000000011369 ) ) ;
#19255=VERTEX_POINT ( 'NONE', #10794 ) ;
#19258=CARTESIAN_POINT ( 'NONE',  ( 233.4038475772933339, -32.38259618943233420, 97.00000000000000000 ) ) ;
#19259=ADVANCED_FACE ( 'NONE', ( #12455 ), #18374, .F. ) ;
#19263=CIRCLE ( 'NONE', #2709, 2.200000000000007283 ) ;
#19267=CARTESIAN_POINT ( 'NONE',  ( 232.5999999999999375, -30.25312499938548072, 96.81714838363319586 ) ) ;
#19270=DIRECTION ( 'NONE',  ( 0.000000000000000000, 0.000000000000000000, 1.000000000000000000 ) ) ;
#19274=DIRECTION ( 'NONE',  ( -0.000000000000000000, -1.000000000000000000, 0.000000000000000000 ) ) ;
#19278=CARTESIAN_POINT ( 'NONE',  ( 235.3564303562499447, -32.20312499938548001, -48.40857419181671162 ) ) ;
#19282=VERTEX_POINT ( 'NONE', #5121 ) ;
#19285=EDGE_CURVE ( 'NONE', #13568, #4792, #15663, .T. ) ;
#19290=CARTESIAN_POINT ( 'NONE',  ( 235.3564303562499447, -31.67812499938547788, 98.40857419181659793 ) ) ;
#19291=CARTESIAN_POINT ( 'NONE',  ( 229.8435696437499587, -34.15312499938547575, -48.40857419181671162 ) ) ;
#19294=AXIS2_PLACEMENT_3D ( 'NONE', #144, #15069, #1879 ) ;
#19296=CARTESIAN_POINT ( 'NONE',  ( 235.3564303562499447, -34.82812499938548001, -51.59142580818350865 ) ) ;
#19299=EDGE_CURVE ( 'NONE', #12317, #1971, #12369, .T. ) ;
#19303=CARTESIAN_POINT ( 'NONE',  ( 235.3564303562499447, -31.34062499938548285, -51.59142580818350865 ) ) ;
#19308=( BOUNDED_CURVE ( )  B_SPLINE_CURVE ( 2, ( #3120, #16325, #15238, #4694, #8887, #312, #6262, #10740, #4404 ),
 .UNSPECIFIED., .F., .F. ) 
 B_SPLINE_CURVE_WITH_KNOTS ( ( 3, 2, 2, 2, 3 ),
 ( 0.6458333333333331483, 0.6527777777777777901, 0.6666666666666666297, 0.6805555555555555802, 0.6874999999999997780 ),
 .UNSPECIFIED. ) 
 CURVE ( )  GEOMETRIC_REPRESENTATION_ITEM ( )  RATIONAL_B_SPLINE_CURVE ( ( 0.9330127018922194093, 0.9330127018922177440, 1.000000000000000000, 0.8660254037844387076, 1.000000000000000000, 0.8660254037844387076, 1.000000000000000000, 0.9330127018922215187, 0.9330127018922194093 ) ) 
 REPRESENTATION_ITEM ( '' )  );
#19309=CARTESIAN_POINT ( 'NONE',  ( 232.5999999999999943, -34.07812499938548001, 103.1828516163667899 ) ) ;
#19313=EDGE_CURVE ( 'NONE', #15345, #1884, #8422, .T. ) ;
#19314=CARTESIAN_POINT ( 'NONE',  ( 233.3129826252978205, -32.00000000000000000, -47.18802777794501679 ) ) ;
#19316=CARTESIAN_POINT ( 'NONE',  ( 230.7429016803060051, -35.00000000000000711, 102.1174602701823488 ) ) ;
#19344=COLOUR_RGB('Light Blue',0.38,0.62,0.78);
#19345=FILL_AREA_STYLE_COLOUR('',#19344);
#19346=FILL_AREA_STYLE('',(#19345));
#19347=SURFACE_STYLE_FILL_AREA(#19346);
#19348=SURFACE_SIDE_STYLE('',(#19347));
#19349=SURFACE_STYLE_USAGE(.BOTH.,#19348);
#19350=PRESENTATION_STYLE_ASSIGNMENT((#19349));
ENDSEC;
END-ISO-10303-21;
